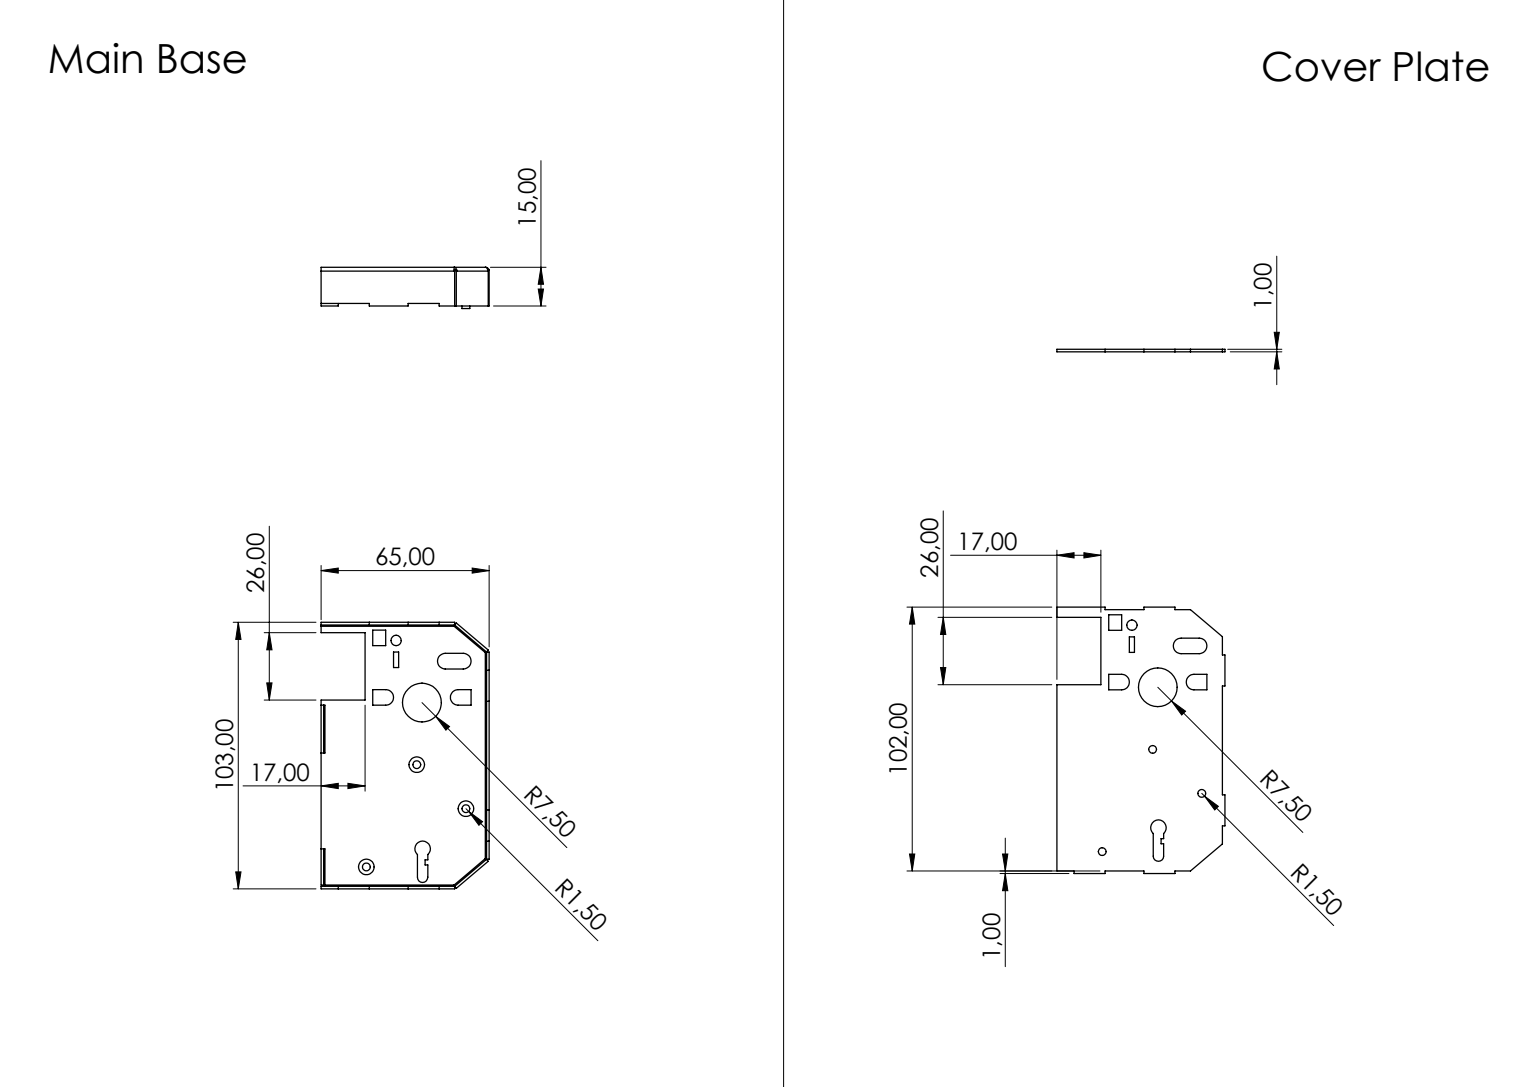
ISO-10303-21;
HEADER;
FILE_DESCRIPTION (('STEP AP214'),
    '1' );
FILE_NAME ('Main Base.step',
    '2026-10-06T13:23:30',
    ( '' ),
    ( '' ),
    'SwSTEP 2.0',
    'SolidWorks 2020',
    '' );
FILE_SCHEMA (( 'AUTOMOTIVE_DESIGN' ));
ENDSEC;

DATA;
#3=VECTOR ( 'NONE', #8048, 1000.000000000000000 ) ;
#6=CARTESIAN_POINT ( 'NONE',  ( -31.50000000000000000, 10.25000000000000000, -137.0552959530000123 ) ) ;
#7=ORIENTED_EDGE ( 'NONE', *, *, #14186, .F. ) ;
#8=PLANE ( 'NONE',  #9401 ) ;
#10=VECTOR ( 'NONE', #7060, 1000.000000000000000 ) ;
#13=DIRECTION ( 'NONE',  ( 0.000000000000000000, 1.000000000000000000, 0.000000000000000000 ) ) ;
#14=CARTESIAN_POINT ( 'NONE',  ( 7.750000000000000000, -40.23606797749999942, -150.0552959529999839 ) ) ;
#16=CARTESIAN_POINT ( 'NONE',  ( -31.00000000000000000, 10.25000000000000000, -150.0552959529999839 ) ) ;
#20=LINE ( 'NONE', #12366, #11445 ) ;
#23=CARTESIAN_POINT ( 'NONE',  ( 6.899000527194547594, -5.343640159924734512, -150.0552959529999839 ) ) ;
#25=EDGE_CURVE ( 'NONE', #1116, #6470, #1636, .T. ) ;
#26=CARTESIAN_POINT ( 'NONE',  ( 32.14594224149999491, 40.79958733410000349, -149.5552959519999945 ) ) ;
#47=ORIENTED_EDGE ( 'NONE', *, *, #19254, .F. ) ;
#51=CARTESIAN_POINT ( 'NONE',  ( 23.00000000000000000, 25.50000000000000000, -151.0552959529999839 ) ) ;
#54=LINE ( 'NONE', #14445, #10 ) ;
#58=CARTESIAN_POINT ( 'NONE',  ( 18.66060904160396916, 20.09818317339116689, -150.0552959529999839 ) ) ;
#59=CARTESIAN_POINT ( 'NONE',  ( -15.75723547076485254, -44.30951848884578226, -150.0552959529999839 ) ) ;
#63=VECTOR ( 'NONE', #17679, 1000.000000000000000 ) ;
#65=LINE ( 'NONE', #14804, #22679 ) ;
#68=EDGE_CURVE ( 'NONE', #3612, #21024, #1516, .T. ) ;
#74=FACE_OUTER_BOUND ( 'NONE', #19510, .T. ) ;
#75=CARTESIAN_POINT ( 'NONE',  ( 7.750000000000000000, -40.23606797749999942, -150.5552959529999839 ) ) ;
#78=EDGE_CURVE ( 'NONE', #537, #6609, #18037, .T. ) ;
#79=CIRCLE ( 'NONE', #13356, 2.000000000000000000 ) ;
#96=VECTOR ( 'NONE', #17767, 1000.000000000000227 ) ;
#102=DIRECTION ( 'NONE',  ( 0.000000000000000000, -1.000000000000000000, 0.000000000000000000 ) ) ;
#103=CARTESIAN_POINT ( 'NONE',  ( -6.024730888589999722, -51.50000000000000000, -149.5552959529999839 ) ) ;
#104=EDGE_CURVE ( 'NONE', #6667, #13256, #16589, .T. ) ;
#105=ORIENTED_EDGE ( 'NONE', *, *, #1127, .F. ) ;
#106=PLANE ( 'NONE',  #15659 ) ;
#111=ORIENTED_EDGE ( 'NONE', *, *, #15327, .F. ) ;
#120=LINE ( 'NONE', #16055, #20099 ) ;
#130=EDGE_LOOP ( 'NONE', ( #1409, #6613, #421, #6495 ) ) ;
#138=DIRECTION ( 'NONE',  ( 1.000000000000000000, 0.000000000000000000, -2.257560236040000027E-12 ) ) ;
#150=EDGE_CURVE ( 'NONE', #19192, #2146, #2095, .T. ) ;
#160=LINE ( 'NONE', #11080, #6868 ) ;
#162=FACE_OUTER_BOUND ( 'NONE', #18152, .T. ) ;
#167=EDGE_LOOP ( 'NONE', ( #4339, #16056, #21520, #10157 ) ) ;
#168=LINE ( 'NONE', #11551, #791 ) ;
#169=CARTESIAN_POINT ( 'NONE',  ( 32.50000000000000000, 40.03620104880000241, -143.0552959529999839 ) ) ;
#170=DIRECTION ( 'NONE',  ( -0.7071067811865474617, -0.7071067811865476838, 0.000000000000000000 ) ) ;
#171=CARTESIAN_POINT ( 'NONE',  ( -3.500000000000000000, 44.50000000000000000, -150.0552959529999839 ) ) ;
#174=VECTOR ( 'NONE', #17768, 1000.000000000000000 ) ;
#186=CARTESIAN_POINT ( 'NONE',  ( 31.50000000000000000, 39.80430157320000006, -149.5552959529999839 ) ) ;
#188=CARTESIAN_POINT ( 'NONE',  ( 31.00000000000000000, 39.80430157320000006, -150.0552959529999839 ) ) ;
#196=CARTESIAN_POINT ( 'NONE',  ( -31.00000000000000000, -50.00000000000000000, -151.0552959529999839 ) ) ;
#198=CARTESIAN_POINT ( 'NONE',  ( 15.50000000000000000, 36.50000000000000000, -151.0552959529999839 ) ) ;
#203=VECTOR ( 'NONE', #22611, 1000.000000000000000 ) ;
#204=CARTESIAN_POINT ( 'NONE',  ( 5.523675324909882001, -48.60111558252668829, -150.0552959529999839 ) ) ;
#211=EDGE_LOOP ( 'NONE', ( #21021, #20847, #5085, #22198, #20574, #16740, #10421 ) ) ;
#212=CARTESIAN_POINT ( 'NONE',  ( -17.62135916506277411, -44.51085694111269930, -150.0552959529999555 ) ) ;
#213=VERTEX_POINT ( 'NONE', #20525 ) ;
#225=EDGE_CURVE ( 'NONE', #11906, #13032, #16136, .T. ) ;
#229=EDGE_CURVE ( 'NONE', #213, #5505, #1240, .T. ) ;
#232=VERTEX_POINT ( 'NONE', #4927 ) ;
#239=CARTESIAN_POINT ( 'NONE',  ( 32.50000000000000000, 0.000000000000000000, -136.0552959530000123 ) ) ;
#240=DIRECTION ( 'NONE',  ( 0.000000000000000000, 0.000000000000000000, 1.000000000000000000 ) ) ;
#244=B_SPLINE_CURVE_WITH_KNOTS ( 'NONE', 3,
 ( #8410, #6271, #1182, #22691, #19238, #11612, #9949, #19010, #11855, #8520, #3074, #13524, #13649, #10184, #20796, #15682, #4613, #4491 ),
 .UNSPECIFIED., .F., .F.,
 ( 4, 2, 2, 2, 2, 2, 2, 2, 4 ),
 ( 0.000000000000000000, 0.1250000000000000000, 0.2500000000000000000, 0.3750000000000000000, 0.5000000000000000000, 0.6250000000000000000, 0.7500000000000000000, 0.8750000000000000000, 1.000000000000000000 ),
 .UNSPECIFIED. ) ;
#250=CARTESIAN_POINT ( 'NONE',  ( 4.107300918301284298, -6.500000000000002665, -150.0552959529999839 ) ) ;
#258=VERTEX_POINT ( 'NONE', #1012 ) ;
#276=ORIENTED_EDGE ( 'NONE', *, *, #19287, .F. ) ;
#278=CARTESIAN_POINT ( 'NONE',  ( 8.750000000000000000, -42.23606797749999942, -150.5552959529999839 ) ) ;
#281=CARTESIAN_POINT ( 'NONE',  ( -15.50000000000000000, 34.50000000000000000, -151.0552959529999839 ) ) ;
#282=DIRECTION ( 'NONE',  ( 0.000000000000000000, -1.000000000000000000, 0.000000000000000000 ) ) ;
#284=FACE_OUTER_BOUND ( 'NONE', #6510, .T. ) ;
#289=CARTESIAN_POINT ( 'NONE',  ( 14.71905350739799623, 33.57650987475365412, -150.0552959530000123 ) ) ;
#294=ORIENTED_EDGE ( 'NONE', *, *, #9256, .T. ) ;
#298=DIRECTION ( 'NONE',  ( 1.000000000000000000, 0.000000000000000000, 0.000000000000000000 ) ) ;
#301=VECTOR ( 'NONE', #7137, 1000.000000000000000 ) ;
#313=PLANE ( 'NONE',  #6728 ) ;
#316=FACE_OUTER_BOUND ( 'NONE', #21887, .T. ) ;
#319=CARTESIAN_POINT ( 'NONE',  ( 6.229273316114841919, -48.94892946173367676, -150.0552959529999839 ) ) ;
#322=VERTEX_POINT ( 'NONE', #6472 ) ;
#328=VERTEX_POINT ( 'NONE', #17655 ) ;
#331=CARTESIAN_POINT ( 'NONE',  ( 13.76008370043819973, 22.44588062467436629, -150.0552959529999839 ) ) ;
#333=LINE ( 'NONE', #16862, #716 ) ;
#335=AXIS2_PLACEMENT_3D ( 'NONE', #20333, #9473, #5804 ) ;
#336=PLANE ( 'NONE',  #4892 ) ;
#340=VECTOR ( 'NONE', #23038, 1000.000000000000000 ) ;
#350=VERTEX_POINT ( 'NONE', #15287 ) ;
#354=EDGE_CURVE ( 'NONE', #22442, #21113, #20876, .T. ) ;
#358=LINE ( 'NONE', #7600, #2620 ) ;
#359=VECTOR ( 'NONE', #21287, 1000.000000000000000 ) ;
#364=DIRECTION ( 'NONE',  ( -1.458135199840000066E-12, 1.723066134159999823E-12, 1.000000000000000000 ) ) ;
#367=LINE ( 'NONE', #7607, #22136 ) ;
#368=EDGE_CURVE ( 'NONE', #19467, #13247, #8432, .T. ) ;
#373=ORIENTED_EDGE ( 'NONE', *, *, #23141, .T. ) ;
#378=AXIS2_PLACEMENT_3D ( 'NONE', #21148, #3175, #6615 ) ;
#381=VECTOR ( 'NONE', #5006, 1000.000000000000000 ) ;
#384=VERTEX_POINT ( 'NONE', #10964 ) ;
#391=EDGE_CURVE ( 'NONE', #6962, #16283, #23127, .T. ) ;
#411=LINE ( 'NONE', #11098, #5597 ) ;
#412=DIRECTION ( 'NONE',  ( 0.000000000000000000, -1.000000000000000000, 0.000000000000000000 ) ) ;
#414=DIRECTION ( 'NONE',  ( 1.000000000000000000, 0.000000000000000000, 0.000000000000000000 ) ) ;
#421=ORIENTED_EDGE ( 'NONE', *, *, #10231, .T. ) ;
#424=CYLINDRICAL_SURFACE ( 'NONE', #5833, 1.500000000000001332 ) ;
#425=ORIENTED_EDGE ( 'NONE', *, *, #10973, .F. ) ;
#427=CARTESIAN_POINT ( 'NONE',  ( 19.45666326950000169, 50.88169314249999786, -136.0552959530000123 ) ) ;
#430=VECTOR ( 'NONE', #16605, 1000.000000000000000 ) ;
#438=CYLINDRICAL_SURFACE ( 'NONE', #17527, 2.999999999999999112 ) ;
#442=CLOSED_SHELL ( 'NONE', ( #9324, #14762, #13056, #18672, #19728, #11827, #3231, #1555, #8168, #17761, #5900, #20748, #17875, #12551, #6898, #10761, #21469, #15064, #5744, #9048, #10757, #19124, #8783, #16660, #5435, #11889, #2238, #21621, #10384, #1685, #10160, #18102, #2306, #16052, #22700, #15391, #3799, #8755, #18283, #22183, #12588, #7262, #14355, #653, #22347, #13377, #4882, #10197, #21282, #7768, #18410, #22521, #11400, #16358, #23317, #3120, #7355, #13403, #22544, #7833, #8957, #20415, #19258, #523, #5604, #17631, #20506, #5512, #10979, #8075, #2679, #9354, #4586, #22200, #23359, #17607, #5542, #23499, #15096, #7365, #9624, #7391, #20151, #23430, #18033, #13348, #7151, #11366, #4409, #5104, #2402, #2042, #18132, #10666, #7930, #20884, #13762, #18713, #18695, #14321, #2065, #14378, #15647, #17406, #4519, #4684, #3694, #21015, #20879, #11134, #7412, #2812, #10561, #7625, #18912, #19316, #9573, #6767, #17249, #18227, #4140, #23025, #5289, #14520, #11229, #648, #6454, #12373, #19083, #6624, #17899, #15037, #11061, #12004, #20941, #16351, #7440, #9553, #16817, #17324, #7025, #19114, #16510, #11613, #13749, #6389, #5831, #9940, #12623, #14887, #20445, #13941, #17758, #16749, #22349, #22437, #10217, #1808, #15771, #12918, #17075, #2483, #7067, #6285, #19351 ) ) ;
#446=ORIENTED_EDGE ( 'NONE', *, *, #8608, .F. ) ;
#450=CARTESIAN_POINT ( 'NONE',  ( -16.51085694111268865, -45.62135916506277056, -150.0552959529999555 ) ) ;
#455=DIRECTION ( 'NONE',  ( -1.000000000000000000, 0.000000000000000000, 0.000000000000000000 ) ) ;
#457=CARTESIAN_POINT ( 'NONE',  ( 19.91945158500000090, -51.14507942810000429, -149.5552959529999839 ) ) ;
#461=LINE ( 'NONE', #9594, #4132 ) ;
#464=AXIS2_PLACEMENT_3D ( 'NONE', #871, #514, #22275 ) ;
#467=VERTEX_POINT ( 'NONE', #15986 ) ;
#479=CARTESIAN_POINT ( 'NONE',  ( 22.50000000000000000, 33.50000000000000000, -150.0552959529999839 ) ) ;
#480=ORIENTED_EDGE ( 'NONE', *, *, #12943, .T. ) ;
#481=PLANE ( 'NONE',  #12091 ) ;
#488=DIRECTION ( 'NONE',  ( 0.000000000000000000, 2.256894259950000208E-12, -1.000000000000000000 ) ) ;
#489=ORIENTED_EDGE ( 'NONE', *, *, #10165, .F. ) ;
#499=ORIENTED_EDGE ( 'NONE', *, *, #14733, .F. ) ;
#501=LINE ( 'NONE', #11416, #1400 ) ;
#502=CARTESIAN_POINT ( 'NONE',  ( -7.500000000000000000, 48.50000000000000000, -150.5552959529999839 ) ) ;
#503=CARTESIAN_POINT ( 'NONE',  ( 31.50000000000000000, -21.03620104879999886, -136.0552959530000123 ) ) ;
#505=ORIENTED_EDGE ( 'NONE', *, *, #9782, .F. ) ;
#507=DIRECTION ( 'NONE',  ( -0.7633862853691872896, 0.6459422414660880296, 5.370703881624201706E-14 ) ) ;
#508=LINE ( 'NONE', #2417, #23112 ) ;
#514=DIRECTION ( 'NONE',  ( 0.000000000000000000, 0.000000000000000000, -1.000000000000000000 ) ) ;
#515=CARTESIAN_POINT ( 'NONE',  ( -12.50000000000000000, 42.50000000000000000, -150.5552959529999839 ) ) ;
#520=DIRECTION ( 'NONE',  ( -1.000000000000000000, 0.000000000000000000, 0.000000000000000000 ) ) ;
#521=EDGE_LOOP ( 'NONE', ( #17341, #16044, #20212, #9730 ) ) ;
#522=DIRECTION ( 'NONE',  ( 0.000000000000000000, 1.000000000000000000, -2.273736754430000208E-12 ) ) ;
#523=ADVANCED_FACE ( 'NONE', ( #5738 ), #15015, .T. ) ;
#529=EDGE_CURVE ( 'NONE', #13555, #22754, #79, .T. ) ;
#533=FACE_OUTER_BOUND ( 'NONE', #22449, .T. ) ;
#537=VERTEX_POINT ( 'NONE', #18717 ) ;
#544=DIRECTION ( 'NONE',  ( 1.000000000000000000, 0.000000000000000000, 0.000000000000000000 ) ) ;
#548=DIRECTION ( 'NONE',  ( 0.000000000000000000, 0.000000000000000000, 1.000000000000000000 ) ) ;
#554=EDGE_CURVE ( 'NONE', #10724, #2155, #2183, .T. ) ;
#556=DIRECTION ( 'NONE',  ( 0.000000000000000000, -1.000000000000000000, 0.000000000000000000 ) ) ;
#557=ORIENTED_EDGE ( 'NONE', *, *, #5693, .F. ) ;
#563=EDGE_LOOP ( 'NONE', ( #12365, #15477, #17819, #6056 ) ) ;
#565=VERTEX_POINT ( 'NONE', #11308 ) ;
#566=CARTESIAN_POINT ( 'NONE',  ( -15.39269908169871393, -46.00000000000000000, -150.0552959529999839 ) ) ;
#567=VERTEX_POINT ( 'NONE', #9642 ) ;
#568=ORIENTED_EDGE ( 'NONE', *, *, #21534, .F. ) ;
#570=CARTESIAN_POINT ( 'NONE',  ( 19.13369214859999801, 51.50000000000000000, -142.8052959529999839 ) ) ;
#571=DIRECTION ( 'NONE',  ( 1.000000000000000000, 0.000000000000000000, -2.255897967639999903E-12 ) ) ;
#575=FACE_OUTER_BOUND ( 'NONE', #12604, .T. ) ;
#581=ORIENTED_EDGE ( 'NONE', *, *, #16197, .T. ) ;
#585=EDGE_LOOP ( 'NONE', ( #1690, #3105, #11478, #4390 ) ) ;
#595=ORIENTED_EDGE ( 'NONE', *, *, #22542, .F. ) ;
#602=CIRCLE ( 'NONE', #14284, 0.5000000000000004441 ) ;
#604=EDGE_LOOP ( 'NONE', ( #581, #786, #19949, #21046 ) ) ;
#605=EDGE_CURVE ( 'NONE', #4355, #13765, #9291, .T. ) ;
#613=CARTESIAN_POINT ( 'NONE',  ( 32.00000000000000000, 32.96379895120000469, -136.0552959530000123 ) ) ;
#617=CARTESIAN_POINT ( 'NONE',  ( 32.50000000000000000, -21.03620104879999886, -136.5552959530000123 ) ) ;
#618=AXIS2_PLACEMENT_3D ( 'NONE', #10592, #19305, #3240 ) ;
#636=FACE_OUTER_BOUND ( 'NONE', #14587, .T. ) ;
#641=CARTESIAN_POINT ( 'NONE',  ( 6.500000000000000000, 13.00000000000000000, -150.0552959529999839 ) ) ;
#648=ADVANCED_FACE ( 'NONE', ( #7405 ), #14667, .F. ) ;
#653=ADVANCED_FACE ( 'NONE', ( #8333 ), #17029, .T. ) ;
#659=VECTOR ( 'NONE', #1651, 1000.000000000000000 ) ;
#663=AXIS2_PLACEMENT_3D ( 'NONE', #6976, #3646, #1872 ) ;
#668=EDGE_CURVE ( 'NONE', #11661, #7563, #4778, .T. ) ;
#671=ORIENTED_EDGE ( 'NONE', *, *, #7862, .F. ) ;
#682=CARTESIAN_POINT ( 'NONE',  ( -32.50000000000000000, 0.000000000000000000, -150.0552959529999839 ) ) ;
#684=EDGE_CURVE ( 'NONE', #11278, #7890, #748, .T. ) ;
#687=DIRECTION ( 'NONE',  ( 0.000000000000000000, -2.256894259950000208E-12, 1.000000000000000000 ) ) ;
#688=FACE_OUTER_BOUND ( 'NONE', #3217, .T. ) ;
#692=EDGE_LOOP ( 'NONE', ( #18060, #16442, #20942, #9453 ) ) ;
#693=CARTESIAN_POINT ( 'NONE',  ( -1.500000000000000222, 44.76558107705237433, -150.0552959530000123 ) ) ;
#707=DIRECTION ( 'NONE',  ( 0.000000000000000000, -2.257144641399999941E-12, -1.000000000000000000 ) ) ;
#709=DIRECTION ( 'NONE',  ( 0.000000000000000000, -1.000000000000000000, 2.257144641399999941E-12 ) ) ;
#710=EDGE_CURVE ( 'NONE', #6873, #1863, #12236, .T. ) ;
#714=VECTOR ( 'NONE', #22848, 1000.000000000000000 ) ;
#715=DIRECTION ( 'NONE',  ( 0.000000000000000000, 1.000000000000000000, 0.000000000000000000 ) ) ;
#716=VECTOR ( 'NONE', #6030, 1000.000000000000227 ) ;
#718=LINE ( 'NONE', #13669, #23526 ) ;
#726=ORIENTED_EDGE ( 'NONE', *, *, #17540, .T. ) ;
#728=CARTESIAN_POINT ( 'NONE',  ( 2.989143058887297588, -0.8786408349372282212, -150.0552959529999839 ) ) ;
#734=ORIENTED_EDGE ( 'NONE', *, *, #17234, .F. ) ;
#748=LINE ( 'NONE', #982, #17937 ) ;
#751=VERTEX_POINT ( 'NONE', #19292 ) ;
#752=DIRECTION ( 'NONE',  ( 0.000000000000000000, 1.000000000000000000, 0.000000000000000000 ) ) ;
#754=ORIENTED_EDGE ( 'NONE', *, *, #1639, .F. ) ;
#759=DIRECTION ( 'NONE',  ( -0.000000000000000000, 1.000000000000000000, 0.000000000000000000 ) ) ;
#763=CARTESIAN_POINT ( 'NONE',  ( 3.175226511974131860, 13.75903940329096287, -150.0552959529999839 ) ) ;
#764=DIRECTION ( 'NONE',  ( 1.000000000000000000, 0.000000000000000000, 0.000000000000000000 ) ) ;
#770=EDGE_CURVE ( 'NONE', #14651, #10724, #872, .T. ) ;
#783=CARTESIAN_POINT ( 'NONE',  ( 19.13369214859999801, 50.50000000000000000, -149.5552959529999839 ) ) ;
#784=EDGE_CURVE ( 'NONE', #19299, #9007, #13572, .T. ) ;
#786=ORIENTED_EDGE ( 'NONE', *, *, #16235, .T. ) ;
#791=VECTOR ( 'NONE', #522, 1000.000000000000000 ) ;
#802=VERTEX_POINT ( 'NONE', #11658 ) ;
#806=ORIENTED_EDGE ( 'NONE', *, *, #21641, .F. ) ;
#809=CARTESIAN_POINT ( 'NONE',  ( 32.50000000000000000, -0.03620104877499999430, -136.0552959530000123 ) ) ;
#816=ORIENTED_EDGE ( 'NONE', *, *, #7911, .T. ) ;
#822=LINE ( 'NONE', #2948, #3 ) ;
#828=CARTESIAN_POINT ( 'NONE',  ( -32.50000000000000000, -24.50000000000000000, -150.0552959529999839 ) ) ;
#837=LINE ( 'NONE', #2962, #359 ) ;
#844=VERTEX_POINT ( 'NONE', #14722 ) ;
#848=AXIS2_PLACEMENT_3D ( 'NONE', #14666, #9179, #20152 ) ;
#850=ORIENTED_EDGE ( 'NONE', *, *, #21643, .T. ) ;
#861=CARTESIAN_POINT ( 'NONE',  ( 31.50000000000000000, -33.03620104880000241, -143.0552959529999839 ) ) ;
#867=CARTESIAN_POINT ( 'NONE',  ( -7.520331543250000195, 50.50000000000000000, -149.5552959529999839 ) ) ;
#871=CARTESIAN_POINT ( 'NONE',  ( 20.50000000000000000, 22.50000000000000000, -151.0552959529999839 ) ) ;
#872=LINE ( 'NONE', #6210, #17180 ) ;
#879=CIRCLE ( 'NONE', #6567, 0.5000000000000004441 ) ;
#902=LINE ( 'NONE', #9909, #21670 ) ;
#903=VERTEX_POINT ( 'NONE', #1455 ) ;
#904=DIRECTION ( 'NONE',  ( 0.000000000000000000, -2.257144641399999941E-12, -1.000000000000000000 ) ) ;
#916=SURFACE_SIDE_STYLE ('',( #15534 ) ) ;
#918=DIRECTION ( 'NONE',  ( 0.000000000000000000, 1.000000000000000000, 0.000000000000000000 ) ) ;
#934=ORIENTED_EDGE ( 'NONE', *, *, #10109, .T. ) ;
#935=VECTOR ( 'NONE', #3004, 1000.000000000000000 ) ;
#938=DIRECTION ( 'NONE',  ( 2.257144641399999941E-12, 0.000000000000000000, 1.000000000000000000 ) ) ;
#944=ORIENTED_EDGE ( 'NONE', *, *, #2669, .F. ) ;
#949=DIRECTION ( 'NONE',  ( -3.552713678800000397E-15, 0.000000000000000000, 1.000000000000000000 ) ) ;
#952=EDGE_CURVE ( 'NONE', #22710, #537, #20436, .T. ) ;
#954=VERTEX_POINT ( 'NONE', #20786 ) ;
#964=CARTESIAN_POINT ( 'NONE',  ( 7.121359165062772334, -1.989143058887300475, -150.0552959530000123 ) ) ;
#968=VERTEX_POINT ( 'NONE', #16742 ) ;
#970=DIRECTION ( 'NONE',  ( 0.000000000000000000, 0.000000000000000000, 1.000000000000000000 ) ) ;
#972=CARTESIAN_POINT ( 'NONE',  ( -13.50000000000000000, -42.80126216859517996, -150.0552959529999839 ) ) ;
#974=DIRECTION ( 'NONE',  ( -1.000000000000000000, 0.000000000000000000, -2.273736754430000208E-12 ) ) ;
#977=DIRECTION ( 'NONE',  ( 0.000000000000000000, 1.000000000000000000, 0.000000000000000000 ) ) ;
#980=EDGE_CURVE ( 'NONE', #11681, #2055, #20670, .T. ) ;
#981=DIRECTION ( 'NONE',  ( 0.000000000000000000, 0.000000000000000000, -1.000000000000000000 ) ) ;
#982=CARTESIAN_POINT ( 'NONE',  ( -31.75000000000000000, 19.50000000000000000, -151.0552959529999839 ) ) ;
#984=EDGE_CURVE ( 'NONE', #1160, #14539, #11488, .T. ) ;
#985=ORIENTED_EDGE ( 'NONE', *, *, #18589, .F. ) ;
#992=AXIS2_PLACEMENT_3D ( 'NONE', #3546, #17821, #18174 ) ;
#995=DIRECTION ( 'NONE',  ( 0.000000000000000000, 1.000000000000000000, 0.000000000000000000 ) ) ;
#1000=CARTESIAN_POINT ( 'NONE',  ( 6.750000000000000000, -36.00000000000000000, -150.0552959529999839 ) ) ;
#1002=PLANE ( 'NONE',  #9686 ) ;
#1003=CARTESIAN_POINT ( 'NONE',  ( 8.701166446538422861, -33.70126136998415944, -150.0552959529999839 ) ) ;
#1012=CARTESIAN_POINT ( 'NONE',  ( 32.14594224169999848, -40.79958733389999992, -136.0552959530000123 ) ) ;
#1017=DIRECTION ( 'NONE',  ( -1.000000000000000000, 0.000000000000000000, 0.000000000000000000 ) ) ;
#1024=AXIS2_PLACEMENT_3D ( 'NONE', #1323, #8898, #21306 ) ;
#1027=ORIENTED_EDGE ( 'NONE', *, *, #68, .F. ) ;
#1029=EDGE_CURVE ( 'NONE', #14361, #2146, #5314, .T. ) ;
#1030=VERTEX_POINT ( 'NONE', #22453 ) ;
#1035=ORIENTED_EDGE ( 'NONE', *, *, #2912, .F. ) ;
#1042=LINE ( 'NONE', #15781, #17871 ) ;
#1048=DIRECTION ( 'NONE',  ( -1.000000000000000000, 0.000000000000000000, 0.000000000000000000 ) ) ;
#1053=DIRECTION ( 'NONE',  ( 1.457985068979999943E-12, -1.723073263340000007E-12, -1.000000000000000000 ) ) ;
#1056=ORIENTED_EDGE ( 'NONE', *, *, #18194, .T. ) ;
#1062=VERTEX_POINT ( 'NONE', #22221 ) ;
#1071=CARTESIAN_POINT ( 'NONE',  ( -7.500000000000000000, 19.50000000000000000, -151.0552959529999839 ) ) ;
#1077=DIRECTION ( 'NONE',  ( -0.7633862853691523176, -0.6459422414661291079, 0.000000000000000000 ) ) ;
#1085=PLANE ( 'NONE',  #7781 ) ;
#1088=EDGE_LOOP ( 'NONE', ( #10214, #10164, #17790, #19615 ) ) ;
#1096=VECTOR ( 'NONE', #10422, 1000.000000000000000 ) ;
#1097=EDGE_CURVE ( 'NONE', #6873, #213, #22682, .T. ) ;
#1102=DIRECTION ( 'NONE',  ( 0.000000000000000000, -1.000000000000000000, 2.273736754430000208E-12 ) ) ;
#1104=VERTEX_POINT ( 'NONE', #12318 ) ;
#1116=VERTEX_POINT ( 'NONE', #19482 ) ;
#1127=EDGE_CURVE ( 'NONE', #7397, #7971, #1042, .T. ) ;
#1128=CARTESIAN_POINT ( 'NONE',  ( 4.055709778248144382, -34.64604587945159864, -150.0552959529999839 ) ) ;
#1132=AXIS2_PLACEMENT_3D ( 'NONE', #9763, #13584, #4554 ) ;
#1134=CIRCLE ( 'NONE', #9463, 3.000000000000000000 ) ;
#1147=CARTESIAN_POINT ( 'NONE',  ( -12.37864083493722589, -41.48914305888730070, -150.0552959530000123 ) ) ;
#1154=AXIS2_PLACEMENT_3D ( 'NONE', #17896, #14566, #16350 ) ;
#1160=VERTEX_POINT ( 'NONE', #8975 ) ;
#1161=DIRECTION ( 'NONE',  ( 1.000000000000000000, 0.000000000000000000, 0.000000000000000000 ) ) ;
#1164=EDGE_LOOP ( 'NONE', ( #6286, #1314, #2583, #12664 ) ) ;
#1167=ORIENTED_EDGE ( 'NONE', *, *, #17932, .F. ) ;
#1176=DIRECTION ( 'NONE',  ( -0.000000000000000000, 1.000000000000000000, 0.000000000000000000 ) ) ;
#1180=EDGE_CURVE ( 'NONE', #7409, #9410, #21742, .T. ) ;
#1181=FACE_OUTER_BOUND ( 'NONE', #20198, .T. ) ;
#1182=CARTESIAN_POINT ( 'NONE',  ( 23.28094649261545612, 39.42349012523344243, -150.0552959530000123 ) ) ;
#1199=PRODUCT_DEFINITION_SHAPE ( 'NONE', 'NONE',  #3542 ) ;
#1205=LINE ( 'NONE', #2743, #20140 ) ;
#1207=CARTESIAN_POINT ( 'NONE',  ( -25.86630785139999844, -51.50000000000000000, -136.5552959530000123 ) ) ;
#1217=VERTEX_POINT ( 'NONE', #20763 ) ;
#1219=CARTESIAN_POINT ( 'NONE',  ( 20.49999999999999645, -20.10730091830128430, -150.0552959529999839 ) ) ;
#1223=VECTOR ( 'NONE', #7853, 1000.000000000000000 ) ;
#1225=AXIS2_PLACEMENT_3D ( 'NONE', #4775, #17268, #977 ) ;
#1226=DIRECTION ( 'NONE',  ( 0.000000000000000000, 2.256988247010000033E-12, 1.000000000000000000 ) ) ;
#1229=DIRECTION ( 'NONE',  ( -1.000000000000000000, 0.000000000000000000, 0.000000000000000000 ) ) ;
#1235=CARTESIAN_POINT ( 'NONE',  ( 3.190548969991207962, -2.742602116062627271, -150.0552959529999839 ) ) ;
#1236=ORIENTED_EDGE ( 'NONE', *, *, #2105, .F. ) ;
#1240=CIRCLE ( 'NONE', #2374, 1.499999999999998446 ) ;
#1241=DIRECTION ( 'NONE',  ( 0.000000000000000000, 0.000000000000000000, 1.000000000000000000 ) ) ;
#1247=DIRECTION ( 'NONE',  ( 1.000000000000000000, 0.000000000000000000, 0.000000000000000000 ) ) ;
#1261=DIRECTION ( 'NONE',  ( 0.7633862853691524286, 0.6459422414661292189, -7.105427357551423529E-15 ) ) ;
#1265=DIRECTION ( 'NONE',  ( 2.257144641399999941E-12, 0.000000000000000000, 1.000000000000000000 ) ) ;
#1267=EDGE_CURVE ( 'NONE', #22797, #7563, #11340, .T. ) ;
#1269=CARTESIAN_POINT ( 'NONE',  ( -16.20076496858231963, -43.91979154561150267, -150.0552959529999839 ) ) ;
#1273=CARTESIAN_POINT ( 'NONE',  ( 5.419791545609164984, -4.700764968563650115, -150.0552959529999555 ) ) ;
#1280=ORIENTED_EDGE ( 'NONE', *, *, #16797, .F. ) ;
#1281=EDGE_LOOP ( 'NONE', ( #19318, #13543, #14266, #17955 ) ) ;
#1287=DIRECTION ( 'NONE',  ( 0.000000000000000000, 0.000000000000000000, -1.000000000000000000 ) ) ;
#1300=DIRECTION ( 'NONE',  ( 0.7071067811865473507, 0.7071067811865477948, 0.000000000000000000 ) ) ;
#1301=VERTEX_POINT ( 'NONE', #20648 ) ;
#1307=ORIENTED_EDGE ( 'NONE', *, *, #10406, .T. ) ;
#1308=VECTOR ( 'NONE', #949, 1000.000000000000000 ) ;
#1313=EDGE_CURVE ( 'NONE', #18451, #1301, #8009, .T. ) ;
#1314=ORIENTED_EDGE ( 'NONE', *, *, #19463, .T. ) ;
#1315=CARTESIAN_POINT ( 'NONE',  ( 32.50000000000000000, 20.96379895120000114, -137.0552959530000123 ) ) ;
#1316=CARTESIAN_POINT ( 'NONE',  ( -32.50000000000000000, 47.50000000000000000, -151.0552959529999839 ) ) ;
#1317=ORIENTED_EDGE ( 'NONE', *, *, #12829, .F. ) ;
#1318=DIRECTION ( 'NONE',  ( 1.000000000000000000, 0.000000000000000000, 0.000000000000000000 ) ) ;
#1320=CARTESIAN_POINT ( 'NONE',  ( 31.50000000000000000, -0.1159497378070000057, -149.5552959529999839 ) ) ;
#1322=ORIENTED_EDGE ( 'NONE', *, *, #3520, .T. ) ;
#1323=CARTESIAN_POINT ( 'NONE',  ( -6.683153925719999222, -51.50000000000000000, -150.0552959529999839 ) ) ;
#1327=EDGE_LOOP ( 'NONE', ( #7904, #19498, #22770, #2319 ) ) ;
#1328=PLANE ( 'NONE',  #6291 ) ;
#1329=FACE_OUTER_BOUND ( 'NONE', #21772, .T. ) ;
#1335=EDGE_CURVE ( 'NONE', #322, #21462, #16714, .T. ) ;
#1344=ORIENTED_EDGE ( 'NONE', *, *, #21880, .F. ) ;
#1355=DIRECTION ( 'NONE',  ( 0.000000000000000000, 0.000000000000000000, 1.000000000000000000 ) ) ;
#1357=DIRECTION ( 'NONE',  ( 0.000000000000000000, 0.000000000000000000, 1.000000000000000000 ) ) ;
#1363=DIRECTION ( 'NONE',  ( 1.457985068979999943E-12, 1.723073263340000007E-12, -1.000000000000000000 ) ) ;
#1370=CARTESIAN_POINT ( 'NONE',  ( -32.50000000000000000, 19.50000000000000000, -151.0552959529999839 ) ) ;
#1371=EDGE_CURVE ( 'NONE', #21536, #6962, #23017, .T. ) ;
#1386=VERTEX_POINT ( 'NONE', #8243 ) ;
#1390=EDGE_LOOP ( 'NONE', ( #8124, #20683, #10522, #22148 ) ) ;
#1391=ORIENTED_EDGE ( 'NONE', *, *, #18377, .F. ) ;
#1392=DIRECTION ( 'NONE',  ( 0.000000000000000000, 1.000000000000000000, 0.000000000000000000 ) ) ;
#1397=ORIENTED_EDGE ( 'NONE', *, *, #13616, .T. ) ;
#1400=VECTOR ( 'NONE', #9278, 1000.000000000000000 ) ;
#1404=B_SPLINE_CURVE_WITH_KNOTS ( 'NONE', 1,
 ( #18749, #9917 ),
 .UNSPECIFIED., .F., .F.,
 ( 2, 2 ),
 ( -6.000000000000000000, 6.000000000000000000 ),
 .UNSPECIFIED. ) ;
#1409=ORIENTED_EDGE ( 'NONE', *, *, #7932, .F. ) ;
#1411=FACE_OUTER_BOUND ( 'NONE', #3594, .T. ) ;
#1417=EDGE_LOOP ( 'NONE', ( #11256, #21139, #23417, #7533 ) ) ;
#1424=VERTEX_POINT ( 'NONE', #21360 ) ;
#1434=ORIENTED_EDGE ( 'NONE', *, *, #9513, .T. ) ;
#1439=EDGE_CURVE ( 'NONE', #1936, #23105, #902, .T. ) ;
#1443=CARTESIAN_POINT ( 'NONE',  ( 23.50000000000000000, -20.50000000000000000, -137.0552959530000123 ) ) ;
#1444=CARTESIAN_POINT ( 'NONE',  ( -13.50000000000000000, -43.00000000000000000, -150.0552959529999839 ) ) ;
#1446=CARTESIAN_POINT ( 'NONE',  ( 18.95053822279999878, 51.50000000000000000, -149.5552959529999839 ) ) ;
#1452=CARTESIAN_POINT ( 'NONE',  ( -6.366307851710000243, -51.50000000000000000, -136.0552959530000123 ) ) ;
#1455=CARTESIAN_POINT ( 'NONE',  ( -31.50000000000000000, 19.50000000000000000, -149.5552959529999839 ) ) ;
#1457=ORIENTED_EDGE ( 'NONE', *, *, #22542, .T. ) ;
#1461=DIRECTION ( 'NONE',  ( 0.000000000000000000, -2.256894259950000208E-12, 1.000000000000000000 ) ) ;
#1463=DIRECTION ( 'NONE',  ( 0.000000000000000000, -1.000000000000000000, 2.257453483404482811E-12 ) ) ;
#1465=CARTESIAN_POINT ( 'NONE',  ( 22.00000000000000000, -20.50000000000000000, -135.0552959530000123 ) ) ;
#1479=FACE_OUTER_BOUND ( 'NONE', #12093, .T. ) ;
#1485=AXIS2_PLACEMENT_3D ( 'NONE', #19777, #12621, #18343 ) ;
#1488=CARTESIAN_POINT ( 'NONE',  ( -31.00000000000000000, 0.000000000000000000, -150.0552959529999839 ) ) ;
#1496=CARTESIAN_POINT ( 'NONE',  ( -15.39269908169872814, -40.00000000000000000, -150.0552959529999555 ) ) ;
#1502=DIRECTION ( 'NONE',  ( 0.000000000000000000, 1.000000000000000000, 0.000000000000000000 ) ) ;
#1505=AXIS2_PLACEMENT_3D ( 'NONE', #2481, #16980, #20221 ) ;
#1516=LINE ( 'NONE', #8738, #9157 ) ;
#1517=ORIENTED_EDGE ( 'NONE', *, *, #20608, .F. ) ;
#1518=CARTESIAN_POINT ( 'NONE',  ( -5.660514123339918768, 20.09808825513541208, -150.0552959529999839 ) ) ;
#1523=DIRECTION ( 'NONE',  ( -0.7633862853691524286, 0.6459422414661292189, -2.886579864030575227E-15 ) ) ;
#1533=EDGE_CURVE ( 'NONE', #17988, #2949, #23369, .T. ) ;
#1536=EDGE_LOOP ( 'NONE', ( #20552, #1056, #13949, #18491 ) ) ;
#1539=ORIENTED_EDGE ( 'NONE', *, *, #18978, .T. ) ;
#1540=CARTESIAN_POINT ( 'NONE',  ( 26.50000000000000000, -20.50000000000000000, -150.0552959529999839 ) ) ;
#1541=ORIENTED_EDGE ( 'NONE', *, *, #3184, .T. ) ;
#1545=EDGE_LOOP ( 'NONE', ( #12281, #19267, #14801, #9609 ) ) ;
#1547=VECTOR ( 'NONE', #16114, 1000.000000000000000 ) ;
#1553=ORIENTED_EDGE ( 'NONE', *, *, #6685, .F. ) ;
#1555=ADVANCED_FACE ( 'NONE', ( #3374 ), #10615, .T. ) ;
#1560=EDGE_CURVE ( 'NONE', #16877, #6475, #54, .T. ) ;
#1562=ORIENTED_EDGE ( 'NONE', *, *, #14186, .T. ) ;
#1564=AXIS2_PLACEMENT_3D ( 'NONE', #18973, #1265, #13968 ) ;
#1572=PLANE ( 'NONE',  #22828 ) ;
#1579=CARTESIAN_POINT ( 'NONE',  ( 1.578081969995054568, -4.285243653077847270, -150.0552959530000123 ) ) ;
#1581=CIRCLE ( 'NONE', #663, 1.499999999999996225 ) ;
#1584=CARTESIAN_POINT ( 'NONE',  ( 18.95053822279999878, -50.00000000000000000, -150.5552959529999839 ) ) ;
#1585=VECTOR ( 'NONE', #13004, 1000.000000000000000 ) ;
#1591=CARTESIAN_POINT ( 'NONE',  ( -10.00000000000000000, 25.50000000000000000, -150.0552959529999839 ) ) ;
#1600=AXIS2_PLACEMENT_3D ( 'NONE', #16675, #18813, #11188 ) ;
#1602=AXIS2_PLACEMENT_3D ( 'NONE', #19669, #3608, #14558 ) ;
#1608=ORIENTED_EDGE ( 'NONE', *, *, #1097, .T. ) ;
#1614=CARTESIAN_POINT ( 'NONE',  ( 8.750000000000000000, -44.61803398880000060, -150.0552959529999839 ) ) ;
#1621=CARTESIAN_POINT ( 'NONE',  ( 19.71940181154762328, 25.42378041200768379, -150.0552959530000123 ) ) ;
#1624=DIRECTION ( 'NONE',  ( -0.6459422414661291079, -0.7633862853691523176, -2.273736754430455399E-12 ) ) ;
#1626=CARTESIAN_POINT ( 'NONE',  ( 1.500000000000000000, -3.500000000000000000, -145.5552959529999839 ) ) ;
#1627=CARTESIAN_POINT ( 'NONE',  ( -13.86630785140000022, 51.50000000000000000, -137.0552959530000123 ) ) ;
#1628=DIRECTION ( 'NONE',  ( 0.000000000000000000, 1.000000000000000000, 0.000000000000000000 ) ) ;
#1632=ORIENTED_EDGE ( 'NONE', *, *, #11313, .T. ) ;
#1634=DIRECTION ( 'NONE',  ( -1.457985068979999943E-12, -1.723073263340000007E-12, 1.000000000000000000 ) ) ;
#1636=LINE ( 'NONE', #23390, #19437 ) ;
#1637=DIRECTION ( 'NONE',  ( -1.000000000000000000, 0.000000000000000000, 0.000000000000000000 ) ) ;
#1639=EDGE_CURVE ( 'NONE', #8510, #12200, #10492, .T. ) ;
#1645=ORIENTED_EDGE ( 'NONE', *, *, #18967, .F. ) ;
#1650=DIRECTION ( 'NONE',  ( -0.000000000000000000, 1.000000000000000000, 0.000000000000000000 ) ) ;
#1651=DIRECTION ( 'NONE',  ( 0.000000000000000000, 2.256894259919999967E-12, 1.000000000000000000 ) ) ;
#1653=CYLINDRICAL_SURFACE ( 'NONE', #14492, 2.000000000000001776 ) ;
#1685=ADVANCED_FACE ( 'NONE', ( #1329 ), #6779, .T. ) ;
#1687=FACE_OUTER_BOUND ( 'NONE', #3541, .T. ) ;
#1688=PLANE ( 'NONE',  #13621 ) ;
#1690=ORIENTED_EDGE ( 'NONE', *, *, #8351, .T. ) ;
#1694=LINE ( 'NONE', #9027, #12502 ) ;
#1697=DIRECTION ( 'NONE',  ( -1.000000000000000000, 0.000000000000000000, 0.000000000000000000 ) ) ;
#1699=VECTOR ( 'NONE', #13346, 1000.000000000000000 ) ;
#1705=VERTEX_POINT ( 'NONE', #1444 ) ;
#1719=DIRECTION ( 'NONE',  ( 0.000000000000000000, 0.000000000000000000, 1.000000000000000000 ) ) ;
#1721=EDGE_CURVE ( 'NONE', #9450, #15840, #16517, .T. ) ;
#1729=ORIENTED_EDGE ( 'NONE', *, *, #12566, .T. ) ;
#1731=CARTESIAN_POINT ( 'NONE',  ( 18.09808825512843455, 20.66051412331523451, -150.0552959529999839 ) ) ;
#1733=AXIS2_PLACEMENT_3D ( 'NONE', #18267, #7423, #1856 ) ;
#1734=LINE ( 'NONE', #12531, #20139 ) ;
#1736=CARTESIAN_POINT ( 'NONE',  ( 31.50000000000000000, -33.03620104880000241, -136.0552959530000123 ) ) ;
#1741=EDGE_LOOP ( 'NONE', ( #373, #5143, #19981, #17412 ) ) ;
#1744=ORIENTED_EDGE ( 'NONE', *, *, #18092, .T. ) ;
#1745=CIRCLE ( 'NONE', #10058, 1.500000000000001332 ) ;
#1748=CARTESIAN_POINT ( 'NONE',  ( 15.50000000000000000, 33.50000000000000000, -150.5552959529999839 ) ) ;
#1750=DIRECTION ( 'NONE',  ( 0.000000000000000000, 0.000000000000000000, 1.000000000000000000 ) ) ;
#1751=EDGE_LOOP ( 'NONE', ( #7956, #16364 ) ) ;
#1752=CARTESIAN_POINT ( 'NONE',  ( -4.500000000000000000, 37.00000000000000000, -150.0552959529999839 ) ) ;
#1755=FACE_OUTER_BOUND ( 'NONE', #6923, .T. ) ;
#1758=EDGE_LOOP ( 'NONE', ( #23285, #13392 ) ) ;
#1760=CARTESIAN_POINT ( 'NONE',  ( -31.50000000000000000, 19.50000000000000000, -143.3052959529999839 ) ) ;
#1763=VECTOR ( 'NONE', #6573, 1000.000000000000000 ) ;
#1764=EDGE_LOOP ( 'NONE', ( #7838, #22300, #568, #5436, #6540, #6553, #20066, #16969, #22280, #14198, #5137, #4958, #14790, #3028, #111 ) ) ;
#1767=FACE_OUTER_BOUND ( 'NONE', #16448, .T. ) ;
#1768=ORIENTED_EDGE ( 'NONE', *, *, #5585, .F. ) ;
#1773=FACE_OUTER_BOUND ( 'NONE', #8786, .T. ) ;
#1776=CARTESIAN_POINT ( 'NONE',  ( -5.449266527207747401, 43.97928331370365385, -150.0552959530000123 ) ) ;
#1782=ORIENTED_EDGE ( 'NONE', *, *, #3711, .T. ) ;
#1783=AXIS2_PLACEMENT_3D ( 'NONE', #3514, #16004, #3050 ) ;
#1786=CARTESIAN_POINT ( 'NONE',  ( 8.750000000000000000, -38.23606797749999942, -151.0552959529999839 ) ) ;
#1787=EDGE_LOOP ( 'NONE', ( #4671, #15389, #22325, #20050 ) ) ;
#1789=ORIENTED_EDGE ( 'NONE', *, *, #10649, .F. ) ;
#1793=DIRECTION ( 'NONE',  ( 0.000000000000000000, -1.000000000000000000, 0.000000000000000000 ) ) ;
#1794=VECTOR ( 'NONE', #22122, 1000.000000000000000 ) ;
#1797=EDGE_CURVE ( 'NONE', #322, #7233, #14526, .T. ) ;
#1799=CARTESIAN_POINT ( 'NONE',  ( 32.50000000000000000, -39.80430157320000006, -149.5552959529999839 ) ) ;
#1803=EDGE_LOOP ( 'NONE', ( #22187, #5500, #20182, #8623 ) ) ;
#1806=LINE ( 'NONE', #14287, #7614 ) ;
#1807=CARTESIAN_POINT ( 'NONE',  ( 7.421918030004952094, -4.285243653077828618, -150.0552959530000123 ) ) ;
#1808=ADVANCED_FACE ( 'NONE', ( #3812, #21902, #18327, #16533, #12834, #3331, #1924, #17854, #2039 ), #1572, .F. ) ;
#1811=CIRCLE ( 'NONE', #15854, 0.5000000000000004441 ) ;
#1814=VECTOR ( 'NONE', #10597, 1000.000000000000000 ) ;
#1815=CARTESIAN_POINT ( 'NONE',  ( -32.50000000000000000, -51.50000000000000000, -149.5552959519999945 ) ) ;
#1831=ORIENTED_EDGE ( 'NONE', *, *, #19563, .T. ) ;
#1833=DIRECTION ( 'NONE',  ( 0.000000000000000000, 0.000000000000000000, 1.000000000000000000 ) ) ;
#1836=CARTESIAN_POINT ( 'NONE',  ( 31.82297112080000190, 40.41789419139999495, -149.5552959529999839 ) ) ;
#1840=EDGE_LOOP ( 'NONE', ( #12851, #21123, #11960, #23063 ) ) ;
#1841=FACE_OUTER_BOUND ( 'NONE', #9955, .T. ) ;
#1844=VECTOR ( 'NONE', #23210, 1000.000000000000000 ) ;
#1846=PLANE ( 'NONE',  #21250 ) ;
#1852=CARTESIAN_POINT ( 'NONE',  ( 32.14594224149999491, 40.79958733410000349, -142.8052959529999839 ) ) ;
#1854=CARTESIAN_POINT ( 'NONE',  ( 19.59648046430000079, -50.76338628540000286, -149.5552959529999839 ) ) ;
#1856=DIRECTION ( 'NONE',  ( 0.000000000000000000, -0.7071067811870332953, 0.7071067811860618502 ) ) ;
#1859=UNCERTAINTY_MEASURE_WITH_UNIT (LENGTH_MEASURE( 1.000000000000000082E-05 ), #20777, 'distance_accuracy_value', 'NONE');
#1860=AXIS2_PLACEMENT_3D ( 'NONE', #4174, #13436, #6191 ) ;
#1863=VERTEX_POINT ( 'NONE', #1799 ) ;
#1872=DIRECTION ( 'NONE',  ( 0.6459422414661299960, -0.7633862853691516515, 0.000000000000000000 ) ) ;
#1879=CIRCLE ( 'NONE', #335, 2.000000000000000000 ) ;
#1881=CIRCLE ( 'NONE', #14023, 7.499999999999999112 ) ;
#1882=CARTESIAN_POINT ( 'NONE',  ( -31.50000000000000000, 19.50000000000000000, -137.0552959530000123 ) ) ;
#1886=LINE ( 'NONE', #7226, #2707 ) ;
#1904=VECTOR ( 'NONE', #5881, 1000.000000000000000 ) ;
#1907=CIRCLE ( 'NONE', #3053, 2.000000000000000888 ) ;
#1914=CARTESIAN_POINT ( 'NONE',  ( 7.750000000000000000, -42.23606797749999942, -150.0552959529999839 ) ) ;
#1921=VECTOR ( 'NONE', #548, 1000.000000000000000 ) ;
#1924=FACE_BOUND ( 'NONE', #3093, .T. ) ;
#1933=CARTESIAN_POINT ( 'NONE',  ( 1.878640834937229442, -5.010856941112704632, -150.0552959530000123 ) ) ;
#1936=VERTEX_POINT ( 'NONE', #12615 ) ;
#1947=DIRECTION ( 'NONE',  ( 0.000000000000000000, 1.000000000000000000, -2.245315044929999938E-12 ) ) ;
#1955=FACE_OUTER_BOUND ( 'NONE', #9695, .T. ) ;
#1969=VECTOR ( 'NONE', #544, 1000.000000000000000 ) ;
#1970=CARTESIAN_POINT ( 'NONE',  ( 4.750000000000000000, -42.61803398880000060, -150.0552959529999839 ) ) ;
#1971=VECTOR ( 'NONE', #138, 1000.000000000000000 ) ;
#1983=EDGE_CURVE ( 'NONE', #23428, #9439, #1806, .T. ) ;
#1989=VECTOR ( 'NONE', #20619, 1000.000000000000000 ) ;
#1991=VECTOR ( 'NONE', #3846, 1000.000000000000227 ) ;
#1993=ORIENTED_EDGE ( 'NONE', *, *, #14572, .F. ) ;
#2002=LINE ( 'NONE', #1760, #15023 ) ;
#2023=DIRECTION ( 'NONE',  ( 0.000000000000000000, 0.000000000000000000, 1.000000000000000000 ) ) ;
#2024=DIRECTION ( 'NONE',  ( -2.257242012349999735E-12, 0.000000000000000000, 1.000000000000000000 ) ) ;
#2027=CARTESIAN_POINT ( 'NONE',  ( 19.84954298779999959, 51.20423285649999912, -150.0552959529999839 ) ) ;
#2028=VERTEX_POINT ( 'NONE', #14642 ) ;
#2030=CARTESIAN_POINT ( 'NONE',  ( 18.95053822279999878, 50.00000000000000000, -149.5552959529999839 ) ) ;
#2033=DIRECTION ( 'NONE',  ( 1.000000000000000000, 0.000000000000000000, 0.000000000000000000 ) ) ;
#2039=FACE_OUTER_BOUND ( 'NONE', #4407, .T. ) ;
#2042=ADVANCED_FACE ( 'NONE', ( #23216 ), #16888, .F. ) ;
#2045=VERTEX_POINT ( 'NONE', #22138 ) ;
#2053=PLANE ( 'NONE',  #1485 ) ;
#2055=VERTEX_POINT ( 'NONE', #4285 ) ;
#2065=ADVANCED_FACE ( 'NONE', ( #16651 ), #2157, .F. ) ;
#2066=CARTESIAN_POINT ( 'NONE',  ( 19.84954298759999958, -51.20423285660000090, -149.5552959529999839 ) ) ;
#2069=CARTESIAN_POINT ( 'NONE',  ( -32.50000000000000000, -36.00000000000000000, -137.0552959530000123 ) ) ;
#2070=EDGE_CURVE ( 'NONE', #350, #12137, #20467, .T. ) ;
#2074=CARTESIAN_POINT ( 'NONE',  ( -3.500000000000000000, 44.50000000000000000, -150.0552959529999839 ) ) ;
#2082=DIRECTION ( 'NONE',  ( 0.7071067811865473507, -0.7071067811865477948, 0.000000000000000000 ) ) ;
#2086=PLANE ( 'NONE',  #2566 ) ;
#2087=DIRECTION ( 'NONE',  ( -2.257144641399999941E-12, 0.000000000000000000, 1.000000000000000000 ) ) ;
#2095=LINE ( 'NONE', #22078, #1969 ) ;
#2102=ORIENTED_EDGE ( 'NONE', *, *, #2124, .T. ) ;
#2105=EDGE_CURVE ( 'NONE', #3167, #20530, #9376, .T. ) ;
#2110=CARTESIAN_POINT ( 'NONE',  ( 31.00000000000000000, 0.000000000000000000, -150.0552959529999839 ) ) ;
#2113=CARTESIAN_POINT ( 'NONE',  ( 31.50000000000000000, -21.03620104879999886, -143.0552959529999839 ) ) ;
#2119=CARTESIAN_POINT ( 'NONE',  ( -15.78524365307783306, -45.92191803000493877, -150.0552959529999839 ) ) ;
#2124=EDGE_CURVE ( 'NONE', #12686, #10612, #4164, .T. ) ;
#2126=CARTESIAN_POINT ( 'NONE',  ( 13.24084097724026243, 23.82487805068920395, -150.0552959529999839 ) ) ;
#2134=AXIS2_PLACEMENT_3D ( 'NONE', #2956, #12223, #21048 ) ;
#2138=EDGE_CURVE ( 'NONE', #11594, #258, #11515, .T. ) ;
#2143=EDGE_CURVE ( 'NONE', #18702, #14446, #16539, .T. ) ;
#2146=VERTEX_POINT ( 'NONE', #20243 ) ;
#2148=CARTESIAN_POINT ( 'NONE',  ( 32.00000000000000000, -40.03620104880000241, -149.5552959529999839 ) ) ;
#2149=VERTEX_POINT ( 'NONE', #3934 ) ;
#2151=DIRECTION ( 'NONE',  ( 0.000000000000000000, -1.000000000000000000, 0.000000000000000000 ) ) ;
#2152=PLANE ( 'NONE',  #21239 ) ;
#2155=VERTEX_POINT ( 'NONE', #11170 ) ;
#2157=PLANE ( 'NONE',  #9509 ) ;
#2159=CARTESIAN_POINT ( 'NONE',  ( 0.000000000000000000, 19.50000000000000000, -150.0552959529999839 ) ) ;
#2170=CARTESIAN_POINT ( 'NONE',  ( 31.96891336220000213, -40.94938100119999547, -149.5552959529999839 ) ) ;
#2171=LINE ( 'NONE', #18112, #10515 ) ;
#2174=LINE ( 'NONE', #9984, #7127 ) ;
#2176=DIRECTION ( 'NONE',  ( -1.449507180940000069E-12, -1.705302565810000055E-12, 1.000000000000000000 ) ) ;
#2177=LINE ( 'NONE', #2525, #1223 ) ;
#2180=CIRCLE ( 'NONE', #20413, 2.999999999999999112 ) ;
#2183=LINE ( 'NONE', #515, #19455 ) ;
#2189=EDGE_CURVE ( 'NONE', #19467, #19419, #6288, .T. ) ;
#2205=LINE ( 'NONE', #3981, #8691 ) ;
#2206=ORIENTED_EDGE ( 'NONE', *, *, #20348, .T. ) ;
#2211=CYLINDRICAL_SURFACE ( 'NONE', #10765, 1.499999999999999556 ) ;
#2212=AXIS2_PLACEMENT_3D ( 'NONE', #7400, #20372, #18578 ) ;
#2223=LINE ( 'NONE', #4348, #16177 ) ;
#2226=CIRCLE ( 'NONE', #5252, 1.500000000000001332 ) ;
#2230=CARTESIAN_POINT ( 'NONE',  ( 4.750000000000000000, -47.00000000000000000, -150.0552959529999839 ) ) ;
#2231=ORIENTED_EDGE ( 'NONE', *, *, #16925, .F. ) ;
#2236=DIRECTION ( 'NONE',  ( 1.000000000000000000, 0.000000000000000000, 0.000000000000000000 ) ) ;
#2237=VERTEX_POINT ( 'NONE', #20696 ) ;
#2238=ADVANCED_FACE ( 'NONE', ( #11990 ), #3397, .T. ) ;
#2245=VECTOR ( 'NONE', #18530, 1000.000000000000000 ) ;
#2250=EDGE_CURVE ( 'NONE', #7971, #2516, #14233, .T. ) ;
#2253=VECTOR ( 'NONE', #14511, 1000.000000000000227 ) ;
#2264=EDGE_LOOP ( 'NONE', ( #18770, #22845, #17331, #9934 ) ) ;
#2268=CARTESIAN_POINT ( 'NONE',  ( 22.50000000000000000, 36.50000000000000000, -151.0552959529999839 ) ) ;
#2273=DIRECTION ( 'NONE',  ( 1.000000000000000000, 0.000000000000000000, 0.000000000000000000 ) ) ;
#2280=EDGE_CURVE ( 'NONE', #4867, #17914, #19704, .T. ) ;
#2293=AXIS2_PLACEMENT_3D ( 'NONE', #20911, #22681, #4836 ) ;
#2300=DIRECTION ( 'NONE',  ( 0.000000000000000000, 0.000000000000000000, 1.000000000000000000 ) ) ;
#2301=DIRECTION ( 'NONE',  ( -1.457985068979999943E-12, 1.723073263340000007E-12, 1.000000000000000000 ) ) ;
#2306=ADVANCED_FACE ( 'NONE', ( #4389 ), #11628, .F. ) ;
#2313=AXIS2_PLACEMENT_3D ( 'NONE', #12312, #21258, #12198 ) ;
#2319=ORIENTED_EDGE ( 'NONE', *, *, #6179, .T. ) ;
#2323=CARTESIAN_POINT ( 'NONE',  ( 19.04211518580000018, -51.50000000000000000, -150.0552959529999839 ) ) ;
#2333=ORIENTED_EDGE ( 'NONE', *, *, #4922, .F. ) ;
#2336=DIRECTION ( 'NONE',  ( -1.000000000000000000, 0.000000000000000000, 2.257453483404482811E-12 ) ) ;
#2345=DIRECTION ( 'NONE',  ( 1.000000000000000000, 0.000000000000000000, 0.000000000000000000 ) ) ;
#2346=DIRECTION ( 'NONE',  ( 0.000000000000000000, -1.000000000000000000, 0.000000000000000000 ) ) ;
#2351=CARTESIAN_POINT ( 'NONE',  ( 8.698929461718192258, -47.52072668388614574, -150.0552959530000123 ) ) ;
#2355=EDGE_LOOP ( 'NONE', ( #21561, #2696, #15045, #934, #13188, #21639, #9708, #5880 ) ) ;
#2362=EDGE_CURVE ( 'NONE', #14060, #11337, #12904, .T. ) ;
#2366=CARTESIAN_POINT ( 'NONE',  ( 18.95053822279999878, 51.50000000000000000, -149.5552959529999839 ) ) ;
#2367=DIRECTION ( 'NONE',  ( 0.7633862853691524286, -0.6459422414661293299, 0.000000000000000000 ) ) ;
#2372=CARTESIAN_POINT ( 'NONE',  ( 13.13369214859999978, 50.50000000000000000, -142.8052959529999839 ) ) ;
#2374=AXIS2_PLACEMENT_3D ( 'NONE', #3874, #20644, #11111 ) ;
#2382=ORIENTED_EDGE ( 'NONE', *, *, #1560, .F. ) ;
#2385=ORIENTED_EDGE ( 'NONE', *, *, #4992, .T. ) ;
#2389=CARTESIAN_POINT ( 'NONE',  ( -5.246523349696126104, 45.51000832343219571, -150.0552959530000123 ) ) ;
#2402=ADVANCED_FACE ( 'NONE', ( #21961 ), #2211, .F. ) ;
#2410=FACE_OUTER_BOUND ( 'NONE', #1741, .T. ) ;
#2417=CARTESIAN_POINT ( 'NONE',  ( -32.50000000000000000, -43.00000000000000000, -149.5552959529999839 ) ) ;
#2426=LINE ( 'NONE', #16805, #21069 ) ;
#2429=FACE_BOUND ( 'NONE', #16832, .T. ) ;
#2433=CARTESIAN_POINT ( 'NONE',  ( 1.133692148550000001, -51.50000000000000000, -136.5552959530000123 ) ) ;
#2435=PLANE ( 'NONE',  #1132 ) ;
#2443=EDGE_CURVE ( 'NONE', #22710, #23189, #3641, .T. ) ;
#2449=DIRECTION ( 'NONE',  ( 0.000000000000000000, 0.000000000000000000, 1.000000000000000000 ) ) ;
#2451=ORIENTED_EDGE ( 'NONE', *, *, #16184, .F. ) ;
#2452=CARTESIAN_POINT ( 'NONE',  ( 25.50000000000000000, 25.50000000000000000, -150.5552959529999839 ) ) ;
#2455=AXIS2_PLACEMENT_3D ( 'NONE', #5739, #10731, #23477 ) ;
#2459=EDGE_CURVE ( 'NONE', #3522, #17914, #14792, .T. ) ;
#2465=ORIENTED_EDGE ( 'NONE', *, *, #8630, .T. ) ;
#2472=CARTESIAN_POINT ( 'NONE',  ( -14.21475634692214740, -45.92191803000493877, -150.0552959529999839 ) ) ;
#2477=LINE ( 'NONE', #20215, #22509 ) ;
#2481=CARTESIAN_POINT ( 'NONE',  ( 4.500000000000000000, -3.500000000000000000, -145.5552959529999839 ) ) ;
#2483=ADVANCED_FACE ( 'NONE', ( #2557 ), #424, .T. ) ;
#2489=CARTESIAN_POINT ( 'NONE',  ( 19.13369214859999801, -51.50000000000000000, -143.0552959529999839 ) ) ;
#2491=ORIENTED_EDGE ( 'NONE', *, *, #19317, .F. ) ;
#2496=CARTESIAN_POINT ( 'NONE',  ( 25.31684607480000082, -45.26810052400000473, -149.5552959529999839 ) ) ;
#2497=FACE_OUTER_BOUND ( 'NONE', #23066, .T. ) ;
#2513=VERTEX_POINT ( 'NONE', #13485 ) ;
#2516=VERTEX_POINT ( 'NONE', #22303 ) ;
#2518=LINE ( 'NONE', #14890, #203 ) ;
#2524=DIRECTION ( 'NONE',  ( 0.000000000000000000, 0.000000000000000000, 1.000000000000000000 ) ) ;
#2525=CARTESIAN_POINT ( 'NONE',  ( -4.500000000000000000, 0.000000000000000000, -150.0552959529999839 ) ) ;
#2532=CARTESIAN_POINT ( 'NONE',  ( 6.000000000000000000, -3.500000000000000000, -140.0552959529999839 ) ) ;
#2537=ORIENTED_EDGE ( 'NONE', *, *, #5328, .F. ) ;
#2541=DIRECTION ( 'NONE',  ( 0.000000000000000000, 1.000000000000000000, 0.000000000000000000 ) ) ;
#2546=CARTESIAN_POINT ( 'NONE',  ( -7.500000000000000000, 42.50000000000000000, -150.5552959529999839 ) ) ;
#2549=EDGE_CURVE ( 'NONE', #21164, #3612, #9668, .T. ) ;
#2557=FACE_OUTER_BOUND ( 'NONE', #10683, .T. ) ;
#2566=AXIS2_PLACEMENT_3D ( 'NONE', #21950, #11323, #3862 ) ;
#2578=EDGE_LOOP ( 'NONE', ( #16493, #15663, #9579, #17088 ) ) ;
#2581=LINE ( 'NONE', #22565, #7194 ) ;
#2583=ORIENTED_EDGE ( 'NONE', *, *, #15352, .F. ) ;
#2605=ORIENTED_EDGE ( 'NONE', *, *, #15186, .F. ) ;
#2607=CARTESIAN_POINT ( 'NONE',  ( 31.50000000020000002, -40.03620104850000416, -136.0552959530000123 ) ) ;
#2620=VECTOR ( 'NONE', #14874, 1000.000000000000000 ) ;
#2624=VERTEX_POINT ( 'NONE', #15862 ) ;
#2631=VECTOR ( 'NONE', #11038, 1000.000000000000000 ) ;
#2638=DIRECTION ( 'NONE',  ( -0.4567501391959232770, -0.5397956190499111351, 0.7071067811858601226 ) ) ;
#2640=CARTESIAN_POINT ( 'NONE',  ( -16.50000000000000000, -43.00000000000000000, -150.0552959529999839 ) ) ;
#2642=VECTOR ( 'NONE', #3185, 1000.000000000000000 ) ;
#2648=DIRECTION ( 'NONE',  ( 1.000000000000000000, 0.000000000000000000, 0.000000000000000000 ) ) ;
#2651=ORIENTED_EDGE ( 'NONE', *, *, #18429, .F. ) ;
#2658=CIRCLE ( 'NONE', #13264, 7.499999999999999112 ) ;
#2662=ORIENTED_EDGE ( 'NONE', *, *, #9008, .T. ) ;
#2668=DIRECTION ( 'NONE',  ( -1.000000000000000000, 0.000000000000000000, 0.000000000000000000 ) ) ;
#2669=EDGE_CURVE ( 'NONE', #9439, #4983, #11932, .T. ) ;
#2670=CARTESIAN_POINT ( 'NONE',  ( 9.736704675116099494, -36.41257638424534093, -150.0552959529999555 ) ) ;
#2679=ADVANCED_FACE ( 'NONE', ( #15987 ), #21468, .F. ) ;
#2690=AXIS2_PLACEMENT_3D ( 'NONE', #6355, #904, #19094 ) ;
#2691=DIRECTION ( 'NONE',  ( 0.000000000000000000, -1.000000000000000000, 0.000000000000000000 ) ) ;
#2693=DIRECTION ( 'NONE',  ( -1.000000000000000000, 0.000000000000000000, 0.000000000000000000 ) ) ;
#2696=ORIENTED_EDGE ( 'NONE', *, *, #1439, .T. ) ;
#2697=CARTESIAN_POINT ( 'NONE',  ( 31.00000000000000000, -39.80430157320000006, -150.0552959529999839 ) ) ;
#2699=ORIENTED_EDGE ( 'NONE', *, *, #22898, .F. ) ;
#2701=CARTESIAN_POINT ( 'NONE',  ( -15.00000000000000000, -43.00000000000000000, -145.5552959529999839 ) ) ;
#2707=VECTOR ( 'NONE', #21869, 1000.000000000000000 ) ;
#2708=VECTOR ( 'NONE', #16689, 1000.000000000000000 ) ;
#2720=VECTOR ( 'NONE', #5141, 1000.000000000000000 ) ;
#2733=ORIENTED_EDGE ( 'NONE', *, *, #21429, .T. ) ;
#2742=ORIENTED_EDGE ( 'NONE', *, *, #7932, .T. ) ;
#2743=CARTESIAN_POINT ( 'NONE',  ( -32.50000000000000000, -51.00000000000000000, -149.5552959529999839 ) ) ;
#2745=VECTOR ( 'NONE', #15481, 1000.000000000000000 ) ;
#2751=CARTESIAN_POINT ( 'NONE',  ( 7.500000000000000888, -3.107300918301275416, -150.0552959530000123 ) ) ;
#2755=EDGE_CURVE ( 'NONE', #16273, #2844, #19674, .T. ) ;
#2756=CARTESIAN_POINT ( 'NONE',  ( 19.04211518569999839, -51.50000000000000000, -150.0552959529999839 ) ) ;
#2761=AXIS2_PLACEMENT_3D ( 'NONE', #16975, #2023, #14961 ) ;
#2762=PLANE ( 'NONE',  #20444 ) ;
#2765=ORIENTED_EDGE ( 'NONE', *, *, #16235, .F. ) ;
#2771=ORIENTED_EDGE ( 'NONE', *, *, #225, .T. ) ;
#2774=CARTESIAN_POINT ( 'NONE',  ( -32.50000000000000000, 19.50000000020000002, -137.0552959530000123 ) ) ;
#2777=CARTESIAN_POINT ( 'NONE',  ( 32.00000000000000000, 40.03620104880000241, -136.0552959530000123 ) ) ;
#2782=CARTESIAN_POINT ( 'NONE',  ( 20.50000000000000000, -20.50000000000000000, -150.0552959529999839 ) ) ;
#2783=PLANE ( 'NONE',  #9361 ) ;
#2786=EDGE_CURVE ( 'NONE', #3754, #16830, #16459, .T. ) ;
#2790=( NAMED_UNIT ( * ) SI_UNIT ( $, .STERADIAN. ) SOLID_ANGLE_UNIT ( ) );
#2807=ORIENTED_EDGE ( 'NONE', *, *, #8060, .T. ) ;
#2812=ADVANCED_FACE ( 'NONE', ( #10845 ), #5397, .T. ) ;
#2817=CARTESIAN_POINT ( 'NONE',  ( 8.750000000000000000, -40.23606797749999942, -150.5552959529999839 ) ) ;
#2828=LINE ( 'NONE', #17456, #18607 ) ;
#2838=LINE ( 'NONE', #15334, #10249 ) ;
#2839=CARTESIAN_POINT ( 'NONE',  ( 21.10099947280546218, -22.34364015992474961, -150.0552959529999839 ) ) ;
#2844=VERTEX_POINT ( 'NONE', #18013 ) ;
#2848=DIRECTION ( 'NONE',  ( -0.7071067811865474617, 0.7071067811865476838, 0.000000000000000000 ) ) ;
#2850=ORIENTED_EDGE ( 'NONE', *, *, #14751, .F. ) ;
#2851=CARTESIAN_POINT ( 'NONE',  ( 0.000000000000000000, -36.00000000000000000, -150.0552959529999839 ) ) ;
#2855=EDGE_CURVE ( 'NONE', #21958, #6865, #16226, .T. ) ;
#2856=LINE ( 'NONE', #3096, #10200 ) ;
#2857=VECTOR ( 'NONE', #7846, 1000.000000000000000 ) ;
#2870=CARTESIAN_POINT ( 'NONE',  ( -14.24276452920772051, -41.69048151115483591, -150.0552959529999839 ) ) ;
#2875=ORIENTED_EDGE ( 'NONE', *, *, #22649, .F. ) ;
#2884=DIRECTION ( 'NONE',  ( 0.000000000000000000, 1.000000000000000000, 0.000000000000000000 ) ) ;
#2891=LINE ( 'NONE', #2777, #9448 ) ;
#2893=CARTESIAN_POINT ( 'NONE',  ( -12.50000000000000000, 0.000000000000000000, -150.0552959529999839 ) ) ;
#2897=CARTESIAN_POINT ( 'NONE',  ( -0.009529796614447350739, 16.74243713058418237, -150.0552959529999839 ) ) ;
#2900=CARTESIAN_POINT ( 'NONE',  ( 5.519240656394276634, 27.95201674008764314, -150.0552959530000123 ) ) ;
#2901=CARTESIAN_POINT ( 'NONE',  ( 5.569521322412388287, -33.22557888555225247, -150.0552959530000123 ) ) ;
#2902=ORIENTED_EDGE ( 'NONE', *, *, #9008, .F. ) ;
#2906=AXIS2_PLACEMENT_3D ( 'NONE', #23201, #23316, #21540 ) ;
#2912=EDGE_CURVE ( 'NONE', #1217, #4350, #11196, .T. ) ;
#2918=DIRECTION ( 'NONE',  ( 1.000000000000000000, 0.000000000000000000, 0.000000000000000000 ) ) ;
#2920=CARTESIAN_POINT ( 'NONE',  ( -31.00000000000000000, 19.50000000000000000, -150.5552959529999839 ) ) ;
#2921=VECTOR ( 'NONE', #13977, 1000.000000000000000 ) ;
#2930=DIRECTION ( 'NONE',  ( 1.000000000000000000, 0.000000000000000000, 0.000000000000000000 ) ) ;
#2941=EDGE_CURVE ( 'NONE', #1936, #19224, #9535, .T. ) ;
#2948=CARTESIAN_POINT ( 'NONE',  ( -4.500000000000000000, 37.00000000000000000, -151.0552959529999839 ) ) ;
#2949=VERTEX_POINT ( 'NONE', #11435 ) ;
#2956=CARTESIAN_POINT ( 'NONE',  ( 19.91945158500000090, -51.14507942810000429, -149.5552959529999839 ) ) ;
#2962=CARTESIAN_POINT ( 'NONE',  ( 6.500000000000000000, 13.00000000000000000, -150.5552959529999839 ) ) ;
#2971=DIRECTION ( 'NONE',  ( 0.000000000000000000, 0.000000000000000000, -1.000000000000000000 ) ) ;
#2972=EDGE_LOOP ( 'NONE', ( #3946, #14498, #19451, #3090 ) ) ;
#2975=VECTOR ( 'NONE', #13953, 1000.000000000000000 ) ;
#2977=CIRCLE ( 'NONE', #16272, 1.499999999999999556 ) ;
#2979=EDGE_CURVE ( 'NONE', #9664, #21739, #2426, .T. ) ;
#2981=CARTESIAN_POINT ( 'NONE',  ( 4.892699081698721919, -0.4999999999999995559, -150.0552959529999839 ) ) ;
#2985=ORIENTED_EDGE ( 'NONE', *, *, #5466, .T. ) ;
#2989=EDGE_CURVE ( 'NONE', #7959, #22754, #17153, .T. ) ;
#2990=CARTESIAN_POINT ( 'NONE',  ( 25.34364015992474961, -18.10099947280545862, -150.0552959529999839 ) ) ;
#3004=DIRECTION ( 'NONE',  ( 0.000000000000000000, 0.000000000000000000, 1.000000000000000000 ) ) ;
#3007=PLANE ( 'NONE',  #19489 ) ;
#3008=DIRECTION ( 'NONE',  ( 1.000000000000000000, 0.000000000000000000, 0.000000000000000000 ) ) ;
#3020=CARTESIAN_POINT ( 'NONE',  ( -15.00000000000000000, -43.00000000000000000, -140.0552959529999839 ) ) ;
#3026=CARTESIAN_POINT ( 'NONE',  ( 5.298801200312091453, -33.35703351611178391, -150.0552959530000123 ) ) ;
#3028=ORIENTED_EDGE ( 'NONE', *, *, #20273, .F. ) ;
#3035=CARTESIAN_POINT ( 'NONE',  ( 25.96278831570000278, 46.03148680969999873, -136.0552959530000123 ) ) ;
#3037=VERTEX_POINT ( 'NONE', #2532 ) ;
#3050=DIRECTION ( 'NONE',  ( -1.000000000000000000, 2.312964634635743450E-15, 0.000000000000000000 ) ) ;
#3053=AXIS2_PLACEMENT_3D ( 'NONE', #16643, #5930, #3928 ) ;
#3074=CARTESIAN_POINT ( 'NONE',  ( 25.42349012524837093, 35.71905350741751306, -150.0552959529999839 ) ) ;
#3081=DIRECTION ( 'NONE',  ( 1.000000000000000000, 0.000000000000000000, 0.000000000000000000 ) ) ;
#3090=ORIENTED_EDGE ( 'NONE', *, *, #2989, .F. ) ;
#3093=EDGE_LOOP ( 'NONE', ( #12559, #10314, #22259, #7596 ) ) ;
#3096=CARTESIAN_POINT ( 'NONE',  ( 25.94418247360000152, 46.04723021459999899, -149.5552959529999839 ) ) ;
#3099=VECTOR ( 'NONE', #12871, 1000.000000000000227 ) ;
#3101=DIRECTION ( 'NONE',  ( 0.6459422414661292189, -0.7633862853691524286, 2.257144641400451094E-12 ) ) ;
#3105=ORIENTED_EDGE ( 'NONE', *, *, #4201, .F. ) ;
#3108=LINE ( 'NONE', #8550, #3259 ) ;
#3110=CARTESIAN_POINT ( 'NONE',  ( 26.12135916506276345, -18.98914305888729714, -150.0552959530000123 ) ) ;
#3111=PLANE ( 'NONE',  #18615 ) ;
#3112=DIRECTION ( 'NONE',  ( 0.000000000000000000, -1.000000000000000000, 0.000000000000000000 ) ) ;
#3117=CIRCLE ( 'NONE', #19457, 1.500000000000000444 ) ;
#3119=CARTESIAN_POINT ( 'NONE',  ( -31.00000000000000000, -50.00000000000000000, -151.0552959529999839 ) ) ;
#3120=ADVANCED_FACE ( 'NONE', ( #13826 ), #3123, .F. ) ;
#3123=PLANE ( 'NONE',  #22201 ) ;
#3125=DIRECTION ( 'NONE',  ( -2.257144641399999941E-12, 0.000000000000000000, 1.000000000000000000 ) ) ;
#3131=ORIENTED_EDGE ( 'NONE', *, *, #1335, .T. ) ;
#3135=CYLINDRICAL_SURFACE ( 'NONE', #3654, 7.500000000000005329 ) ;
#3137=CARTESIAN_POINT ( 'NONE',  ( 19.13369214879999802, 50.49999999980000354, -136.0552959530000123 ) ) ;
#3138=VERTEX_POINT ( 'NONE', #4897 ) ;
#3140=CARTESIAN_POINT ( 'NONE',  ( -0.2409605966970265190, 23.82477348803106310, -150.0552959529999839 ) ) ;
#3143=ORIENTED_EDGE ( 'NONE', *, *, #15508, .F. ) ;
#3153=DIRECTION ( 'NONE',  ( 0.000000000000000000, 1.000000000000000000, 0.000000000000000000 ) ) ;
#3158=CARTESIAN_POINT ( 'NONE',  ( 18.66051412330858383, 24.90191174486891867, -150.0552959529999839 ) ) ;
#3160=PLANE ( 'NONE',  #3671 ) ;
#3163=DIRECTION ( 'NONE',  ( 1.000000000000000000, 0.000000000000000000, -2.257157423930000049E-12 ) ) ;
#3167=VERTEX_POINT ( 'NONE', #11782 ) ;
#3171=PLANE ( 'NONE',  #18577 ) ;
#3172=LINE ( 'NONE', #13873, #5388 ) ;
#3174=EDGE_LOOP ( 'NONE', ( #2231, #8769, #20425, #47 ) ) ;
#3175=DIRECTION ( 'NONE',  ( 0.000000000000000000, 0.000000000000000000, 1.000000000000000000 ) ) ;
#3183=DIRECTION ( 'NONE',  ( 0.000000000000000000, 0.000000000000000000, 1.000000000000000000 ) ) ;
#3184=EDGE_CURVE ( 'NONE', #7540, #21170, #14994, .T. ) ;
#3185=DIRECTION ( 'NONE',  ( 0.000000000000000000, 0.000000000000000000, 1.000000000000000000 ) ) ;
#3191=CYLINDRICAL_SURFACE ( 'NONE', #10849, 1.500000000000001332 ) ;
#3203=VERTEX_POINT ( 'NONE', #6440 ) ;
#3208=ORIENTED_EDGE ( 'NONE', *, *, #20168, .T. ) ;
#3209=DIRECTION ( 'NONE',  ( 2.257144641399999941E-12, 0.000000000000000000, 1.000000000000000000 ) ) ;
#3210=EDGE_CURVE ( 'NONE', #13163, #3680, #12023, .T. ) ;
#3213=FACE_OUTER_BOUND ( 'NONE', #8069, .T. ) ;
#3217=EDGE_LOOP ( 'NONE', ( #985, #5840, #3336, #1391 ) ) ;
#3219=DIRECTION ( 'NONE',  ( 2.326943610902514898E-15, 0.000000000000000000, 1.000000000000000000 ) ) ;
#3221=CARTESIAN_POINT ( 'NONE',  ( 32.50000000000000000, 32.96379895120000469, -137.0552959530000123 ) ) ;
#3227=FACE_OUTER_BOUND ( 'NONE', #13579, .T. ) ;
#3231=ADVANCED_FACE ( 'NONE', ( #10237 ), #13934, .F. ) ;
#3232=DIRECTION ( 'NONE',  ( 0.000000000000000000, 0.000000000000000000, 1.000000000000000000 ) ) ;
#3233=CARTESIAN_POINT ( 'NONE',  ( 32.50000000000000000, 20.96379895120000114, -136.0552959530000123 ) ) ;
#3235=VERTEX_POINT ( 'NONE', #10937 ) ;
#3240=DIRECTION ( 'NONE',  ( 1.000000000000000000, 0.000000000000000000, -2.257453483404485639E-12 ) ) ;
#3250=( NAMED_UNIT ( * ) PLANE_ANGLE_UNIT ( ) SI_UNIT ( $, .RADIAN. ) );
#3252=EDGE_LOOP ( 'NONE', ( #15305, #13897, #15340, #2662 ) ) ;
#3259=VECTOR ( 'NONE', #12128, 1000.000000000000000 ) ;
#3263=DIRECTION ( 'NONE',  ( 0.000000000000000000, 0.000000000000000000, -1.000000000000000000 ) ) ;
#3264=DIRECTION ( 'NONE',  ( 2.257144641399999941E-12, 0.000000000000000000, 1.000000000000000000 ) ) ;
#3273=VECTOR ( 'NONE', #14136, 1000.000000000000000 ) ;
#3285=CARTESIAN_POINT ( 'NONE',  ( -7.500000000000000000, 19.50000000000000000, -150.0552959529999839 ) ) ;
#3292=ADVANCED_BREP_SHAPE_REPRESENTATION ( '', ( #11774, #5025 ), #8794 ) ;
#3293=VERTEX_POINT ( 'NONE', #26 ) ;
#3301=CARTESIAN_POINT ( 'NONE',  ( -6.683153925719999222, 51.50000000000000000, -150.0552959529999839 ) ) ;
#3302=FACE_OUTER_BOUND ( 'NONE', #3780, .T. ) ;
#3306=ORIENTED_EDGE ( 'NONE', *, *, #1983, .F. ) ;
#3317=CARTESIAN_POINT ( 'NONE',  ( 4.750000000000000000, -47.00000000000000000, -151.0552959529999839 ) ) ;
#3319=ORIENTED_EDGE ( 'NONE', *, *, #17732, .F. ) ;
#3320=CARTESIAN_POINT ( 'NONE',  ( -2.979194667911468919, 46.44907581354189574, -150.0552959529999839 ) ) ;
#3321=AXIS2_PLACEMENT_3D ( 'NONE', #2489, #20926, #17221 ) ;
#3328=ORIENTED_EDGE ( 'NONE', *, *, #16339, .T. ) ;
#3331=FACE_BOUND ( 'NONE', #9585, .T. ) ;
#3334=EDGE_CURVE ( 'NONE', #4867, #6268, #5596, .T. ) ;
#3335=DIRECTION ( 'NONE',  ( 0.000000000000000000, 1.000000000000000000, 0.000000000000000000 ) ) ;
#3336=ORIENTED_EDGE ( 'NONE', *, *, #4732, .T. ) ;
#3345=EDGE_LOOP ( 'NONE', ( #21709, #3988, #14253, #8703 ) ) ;
#3351=LINE ( 'NONE', #6926, #20502 ) ;
#3354=AXIS2_PLACEMENT_3D ( 'NONE', #14225, #21490, #20149 ) ;
#3357=ORIENTED_EDGE ( 'NONE', *, *, #12944, .T. ) ;
#3361=CARTESIAN_POINT ( 'NONE',  ( 31.50000000000000000, 39.80430157320000006, -143.0552959529999839 ) ) ;
#3365=FACE_OUTER_BOUND ( 'NONE', #8140, .T. ) ;
#3371=VECTOR ( 'NONE', #1048, 1000.000000000000000 ) ;
#3372=ORIENTED_EDGE ( 'NONE', *, *, #17087, .F. ) ;
#3374=FACE_OUTER_BOUND ( 'NONE', #13985, .T. ) ;
#3380=CARTESIAN_POINT ( 'NONE',  ( 17.49993271304850140, 22.89748944252527352, -150.0552959529999839 ) ) ;
#3381=CARTESIAN_POINT ( 'NONE',  ( -16.50000000000000000, -43.00000000000000000, -150.0552959529999839 ) ) ;
#3384=FACE_OUTER_BOUND ( 'NONE', #20907, .T. ) ;
#3389=EDGE_CURVE ( 'NONE', #19876, #11512, #16315, .T. ) ;
#3390=ORIENTED_EDGE ( 'NONE', *, *, #1097, .F. ) ;
#3392=VECTOR ( 'NONE', #6509, 1000.000000000000000 ) ;
#3394=DIRECTION ( 'NONE',  ( 0.000000000000000000, 1.000000000000000000, 0.000000000000000000 ) ) ;
#3397=PLANE ( 'NONE',  #22069 ) ;
#3400=EDGE_CURVE ( 'NONE', #11681, #10143, #23337, .T. ) ;
#3411=CIRCLE ( 'NONE', #22403, 0.5000000000000004441 ) ;
#3417=CARTESIAN_POINT ( 'NONE',  ( 0.8371776177479999248, 14.00000000000000000, -144.0552959529999839 ) ) ;
#3419=EDGE_CURVE ( 'NONE', #16273, #6526, #18796, .T. ) ;
#3421=PLANE ( 'NONE',  #5734 ) ;
#3426=CARTESIAN_POINT ( 'NONE',  ( 25.34364015992475316, -22.89900052719453427, -150.0552959529999839 ) ) ;
#3430=ORIENTED_EDGE ( 'NONE', *, *, #2459, .T. ) ;
#3431=VECTOR ( 'NONE', #23044, 1000.000000000000000 ) ;
#3437=CARTESIAN_POINT ( 'NONE',  ( -31.50000000000000000, 1.000000000000000000, -149.5552959529999839 ) ) ;
#3438=ORIENTED_EDGE ( 'NONE', *, *, #1335, .F. ) ;
#3439=CARTESIAN_POINT ( 'NONE',  ( -32.50000000000000000, 19.50000000000000000, -150.5552959529999839 ) ) ;
#3448=VECTOR ( 'NONE', #5360, 1000.000000000000227 ) ;
#3449=AXIS2_PLACEMENT_3D ( 'NONE', #17447, #1176, #12437 ) ;
#3451=EDGE_CURVE ( 'NONE', #1104, #565, #16656, .T. ) ;
#3455=LINE ( 'NONE', #8662, #6371 ) ;
#3464=DIRECTION ( 'NONE',  ( 0.000000000000000000, -1.000000000000000000, -2.257144641399999941E-12 ) ) ;
#3476=ORIENTED_EDGE ( 'NONE', *, *, #4659, .T. ) ;
#3492=EDGE_LOOP ( 'NONE', ( #4975, #17946, #1517, #5112 ) ) ;
#3506=CARTESIAN_POINT ( 'NONE',  ( 20.10199673422639322, 25.50000000000000355, -150.0552959529999839 ) ) ;
#3513=DIRECTION ( 'NONE',  ( 0.000000000000000000, -1.000000000000000000, -2.273736754430000208E-12 ) ) ;
#3514=CARTESIAN_POINT ( 'NONE',  ( 22.50000000000000000, 36.50000000000000000, -150.0552959529999839 ) ) ;
#3515=CARTESIAN_POINT ( 'NONE',  ( 32.05742780220000299, -40.87448416729999678, -150.0552959529999839 ) ) ;
#3520=EDGE_CURVE ( 'NONE', #3906, #16283, #8539, .T. ) ;
#3522=VERTEX_POINT ( 'NONE', #15348 ) ;
#3524=DIRECTION ( 'NONE',  ( 0.6459422414661339928, -0.7633862853691482098, 0.000000000000000000 ) ) ;
#3527=VERTEX_POINT ( 'NONE', #21181 ) ;
#3528=DIRECTION ( 'NONE',  ( 1.000000000000000000, 0.000000000000000000, 0.000000000000000000 ) ) ;
#3531=DIRECTION ( 'NONE',  ( -0.000000000000000000, 1.000000000000000000, 0.000000000000000000 ) ) ;
#3537=EDGE_CURVE ( 'NONE', #19834, #8510, #4749, .T. ) ;
#3539=DIRECTION ( 'NONE',  ( 0.000000000000000000, -1.000000000000000000, 0.000000000000000000 ) ) ;
#3541=EDGE_LOOP ( 'NONE', ( #20081, #14631, #21867, #7152 ) ) ;
#3542=PRODUCT_DEFINITION ( 'UNKNOWN', '', #9995, #14687 ) ;
#3546=CARTESIAN_POINT ( 'NONE',  ( 0.000000000000000000, 0.000000000000000000, -140.0552959529999839 ) ) ;
#3550=CARTESIAN_POINT ( 'NONE',  ( -31.50000000000000000, 16.00000000000000000, -144.0552959529999839 ) ) ;
#3560=DIRECTION ( 'NONE',  ( 0.000000000000000000, -1.000000000000000000, 0.000000000000000000 ) ) ;
#3562=DIRECTION ( 'NONE',  ( 0.000000000000000000, 1.000000000000000000, 0.000000000000000000 ) ) ;
#3563=ORIENTED_EDGE ( 'NONE', *, *, #11008, .F. ) ;
#3566=ORIENTED_EDGE ( 'NONE', *, *, #15586, .F. ) ;
#3569=EDGE_CURVE ( 'NONE', #4645, #232, #1205, .T. ) ;
#3576=CARTESIAN_POINT ( 'NONE',  ( 0.000000000000000000, 0.000000000000000000, -151.0552959529999839 ) ) ;
#3579=CARTESIAN_POINT ( 'NONE',  ( -18.00000000000000000, -43.00000000000000000, -150.0552959529999839 ) ) ;
#3580=ORIENTED_EDGE ( 'NONE', *, *, #9946, .F. ) ;
#3590=AXIS2_PLACEMENT_3D ( 'NONE', #3035, #1363, #23249 ) ;
#3594=EDGE_LOOP ( 'NONE', ( #1608, #16064, #8873, #5714 ) ) ;
#3608=DIRECTION ( 'NONE',  ( 0.000000000000000000, 0.000000000000000000, 1.000000000000000000 ) ) ;
#3612=VERTEX_POINT ( 'NONE', #19261 ) ;
#3616=ORIENTED_EDGE ( 'NONE', *, *, #980, .F. ) ;
#3619=ORIENTED_EDGE ( 'NONE', *, *, #22626, .F. ) ;
#3623=AXIS2_PLACEMENT_3D ( 'NONE', #5109, #21895, #23434 ) ;
#3635=ORIENTED_EDGE ( 'NONE', *, *, #14869, .T. ) ;
#3641=LINE ( 'NONE', #10875, #21424 ) ;
#3643=CARTESIAN_POINT ( 'NONE',  ( -7.500000000000000000, 25.50000000000000000, -150.0552959529999839 ) ) ;
#3646=DIRECTION ( 'NONE',  ( -0.7633862853691524286, -0.6459422414661293299, 5.800915303671162679E-15 ) ) ;
#3654=AXIS2_PLACEMENT_3D ( 'NONE', #17640, #11920, #8468 ) ;
#3671=AXIS2_PLACEMENT_3D ( 'NONE', #4699, #3264, #14213 ) ;
#3673=ORIENTED_EDGE ( 'NONE', *, *, #18818, .F. ) ;
#3679=DIRECTION ( 'NONE',  ( 0.000000000000000000, 1.000000000000000000, 0.000000000000000000 ) ) ;
#3680=VERTEX_POINT ( 'NONE', #19031 ) ;
#3692=CARTESIAN_POINT ( 'NONE',  ( -31.00000000000000000, -51.50000000000000000, -149.5552959529999839 ) ) ;
#3693=CYLINDRICAL_SURFACE ( 'NONE', #3750, 1.500000000000001554 ) ;
#3694=ADVANCED_FACE ( 'NONE', ( #4639 ), #20947, .T. ) ;
#3704=CARTESIAN_POINT ( 'NONE',  ( -31.50000000000000000, 12.00000000000000000, -144.0552959529999839 ) ) ;
#3705=ORIENTED_EDGE ( 'NONE', *, *, #12699, .T. ) ;
#3711=EDGE_CURVE ( 'NONE', #11278, #1062, #5569, .T. ) ;
#3718=FACE_OUTER_BOUND ( 'NONE', #13500, .T. ) ;
#3721=DIRECTION ( 'NONE',  ( 1.000000000000000000, 0.000000000000000000, 2.257144641399999941E-12 ) ) ;
#3736=CARTESIAN_POINT ( 'NONE',  ( -14.08020845438083235, -44.20076496858382598, -150.0552959529999839 ) ) ;
#3743=LINE ( 'NONE', #10983, #16613 ) ;
#3744=DIRECTION ( 'NONE',  ( -1.000000000000000000, 0.000000000000000000, 0.000000000000000000 ) ) ;
#3750=AXIS2_PLACEMENT_3D ( 'NONE', #11052, #21795, #7139 ) ;
#3753=CARTESIAN_POINT ( 'NONE',  ( 32.50000000000000000, 20.96379895120000114, -136.0552959530000123 ) ) ;
#3754=VERTEX_POINT ( 'NONE', #3317 ) ;
#3756=ORIENTED_EDGE ( 'NONE', *, *, #1371, .T. ) ;
#3763=ORIENTED_EDGE ( 'NONE', *, *, #6126, .F. ) ;
#3768=AXIS2_PLACEMENT_3D ( 'NONE', #1000, #22644, #13718 ) ;
#3773=VECTOR ( 'NONE', #3539, 1000.000000000000000 ) ;
#3774=DIRECTION ( 'NONE',  ( 1.000000000000000000, 0.000000000000000000, 0.000000000000000000 ) ) ;
#3780=EDGE_LOOP ( 'NONE', ( #4972, #20052 ) ) ;
#3789=VECTOR ( 'NONE', #16063, 1000.000000000000000 ) ;
#3793=AXIS2_PLACEMENT_3D ( 'NONE', #17478, #19145, #2848 ) ;
#3794=CARTESIAN_POINT ( 'NONE',  ( 32.50000000000000000, 0.000000000000000000, -136.0552959530000123 ) ) ;
#3796=DIRECTION ( 'NONE',  ( 0.000000000000000000, 1.000000000000000000, 0.000000000000000000 ) ) ;
#3797=VERTEX_POINT ( 'NONE', #10907 ) ;
#3799=ADVANCED_FACE ( 'NONE', ( #10438 ), #19744, .T. ) ;
#3803=CARTESIAN_POINT ( 'NONE',  ( 4.109450702737304617, -4.961822747171590997, -150.0552959529999839 ) ) ;
#3807=ORIENTED_EDGE ( 'NONE', *, *, #13030, .T. ) ;
#3812=FACE_BOUND ( 'NONE', #21940, .T. ) ;
#3820=CARTESIAN_POINT ( 'NONE',  ( -13.86630785140000022, -50.50000000000000000, -143.0552959529999839 ) ) ;
#3824=ORIENTED_EDGE ( 'NONE', *, *, #18377, .T. ) ;
#3843=VECTOR ( 'NONE', #20387, 1000.000000000000000 ) ;
#3846=DIRECTION ( 'NONE',  ( -0.6459422414661291079, -0.7633862853691523176, -2.273736754430455399E-12 ) ) ;
#3848=CARTESIAN_POINT ( 'NONE',  ( 4.750000000000000000, -47.00000000000000000, -150.5552959529999839 ) ) ;
#3850=ORIENTED_EDGE ( 'NONE', *, *, #225, .F. ) ;
#3853=LINE ( 'NONE', #4321, #2708 ) ;
#3861=DIRECTION ( 'NONE',  ( 0.000000000000000000, -1.000000000000000000, 0.000000000000000000 ) ) ;
#3862=DIRECTION ( 'NONE',  ( 0.000000000000000000, 0.000000000000000000, -1.000000000000000000 ) ) ;
#3863=LINE ( 'NONE', #5286, #18515 ) ;
#3870=VERTEX_POINT ( 'NONE', #22336 ) ;
#3874=CARTESIAN_POINT ( 'NONE',  ( 31.00000000000000000, 39.80430157320000006, -149.5552959529999839 ) ) ;
#3878=VECTOR ( 'NONE', #18845, 1000.000000000000000 ) ;
#3885=DIRECTION ( 'NONE',  ( 0.000000000000000000, 0.000000000000000000, 1.000000000000000000 ) ) ;
#3889=EDGE_CURVE ( 'NONE', #565, #13650, #5798, .T. ) ;
#3892=FACE_OUTER_BOUND ( 'NONE', #11757, .T. ) ;
#3893=ORIENTED_EDGE ( 'NONE', *, *, #14106, .T. ) ;
#3904=LINE ( 'NONE', #682, #19720 ) ;
#3905=VERTEX_POINT ( 'NONE', #15199 ) ;
#3906=VERTEX_POINT ( 'NONE', #457 ) ;
#3910=CARTESIAN_POINT ( 'NONE',  ( 12.46241645105735607, 25.07592078380848477, -150.0552959529999839 ) ) ;
#3928=DIRECTION ( 'NONE',  ( 1.000000000000000000, 0.000000000000000000, 0.000000000000000000 ) ) ;
#3934=CARTESIAN_POINT ( 'NONE',  ( 20.50000000000000000, 25.50000000000000000, -150.0552959529999839 ) ) ;
#3938=EDGE_CURVE ( 'NONE', #9007, #12574, #4130, .T. ) ;
#3941=LINE ( 'NONE', #9383, #5278 ) ;
#3945=VECTOR ( 'NONE', #16254, 1000.000000000000000 ) ;
#3946=ORIENTED_EDGE ( 'NONE', *, *, #12869, .F. ) ;
#3951=DIRECTION ( 'NONE',  ( -2.252420472359999842E-12, 0.000000000000000000, 1.000000000000000000 ) ) ;
#3959=EDGE_CURVE ( 'NONE', #23250, #15992, #333, .T. ) ;
#3965=ORIENTED_EDGE ( 'NONE', *, *, #7207, .F. ) ;
#3968=DIRECTION ( 'NONE',  ( 0.7071067811870332953, 0.000000000000000000, 0.7071067811860618502 ) ) ;
#3981=CARTESIAN_POINT ( 'NONE',  ( -4.500000000000000000, 34.00000000000000000, -150.5552959529999839 ) ) ;
#3982=ORIENTED_EDGE ( 'NONE', *, *, #17873, .T. ) ;
#3988=ORIENTED_EDGE ( 'NONE', *, *, #13351, .T. ) ;
#3991=VECTOR ( 'NONE', #18606, 1000.000000000000000 ) ;
#3999=CARTESIAN_POINT ( 'NONE',  ( -32.50000000000000000, 50.00000000000000000, -149.5552959529999839 ) ) ;
#4004=CARTESIAN_POINT ( 'NONE',  ( 8.250000000000000000, -42.23606797749999942, -151.0552959529999839 ) ) ;
#4007=CARTESIAN_POINT ( 'NONE',  ( 7.750000000000000000, -41.23606797749999942, -151.0552959529999839 ) ) ;
#4015=CARTESIAN_POINT ( 'NONE',  ( -17.39900052719453072, -44.84364015992474606, -150.0552959529999555 ) ) ;
#4020=CARTESIAN_POINT ( 'NONE',  ( -31.00000000000000000, -36.00000000000000000, -149.5552959529999839 ) ) ;
#4029=ORIENTED_EDGE ( 'NONE', *, *, #12431, .T. ) ;
#4030=DIRECTION ( 'NONE',  ( 0.000000000000000000, 0.000000000000000000, 1.000000000000000000 ) ) ;
#4038=VERTEX_POINT ( 'NONE', #23046 ) ;
#4044=CIRCLE ( 'NONE', #10471, 1.500000000000001332 ) ;
#4047=CARTESIAN_POINT ( 'NONE',  ( 19.13369214859999801, 50.50000000000000000, -142.8052959529999839 ) ) ;
#4053=CARTESIAN_POINT ( 'NONE',  ( -31.50000000000000000, -36.00000000000000000, -137.0552959530000123 ) ) ;
#4061=CARTESIAN_POINT ( 'NONE',  ( -7.500000000000000000, 42.50000000000000000, -150.0552959529999839 ) ) ;
#4063=ORIENTED_EDGE ( 'NONE', *, *, #16184, .T. ) ;
#4065=FACE_OUTER_BOUND ( 'NONE', #6237, .T. ) ;
#4067=CYLINDRICAL_SURFACE ( 'NONE', #1600, 7.500000000000005329 ) ;
#4082=ORIENTED_EDGE ( 'NONE', *, *, #20435, .T. ) ;
#4086=CARTESIAN_POINT ( 'NONE',  ( -2.500000000000000000, 40.00000000000000000, -151.0552959529999839 ) ) ;
#4088=CARTESIAN_POINT ( 'NONE',  ( 13.13369214859999978, 51.50000000000000000, -137.0552959530000123 ) ) ;
#4090=EDGE_CURVE ( 'NONE', #13352, #13032, #9939, .T. ) ;
#4103=VECTOR ( 'NONE', #102, 1000.000000000000000 ) ;
#4116=CARTESIAN_POINT ( 'NONE',  ( 8.750000000000001776, -47.26504245777761071, -150.0552959530000123 ) ) ;
#4117=ORIENTED_EDGE ( 'NONE', *, *, #984, .F. ) ;
#4126=ORIENTED_EDGE ( 'NONE', *, *, #2070, .T. ) ;
#4127=DIRECTION ( 'NONE',  ( 1.000000000000000000, 0.000000000000000000, 0.000000000000000000 ) ) ;
#4129=LINE ( 'NONE', #20437, #11090 ) ;
#4130=LINE ( 'NONE', #7693, #12856 ) ;
#4132=VECTOR ( 'NONE', #7924, 1000.000000000000000 ) ;
#4135=VERTEX_POINT ( 'NONE', #23397 ) ;
#4140=ADVANCED_FACE ( 'NONE', ( #1755 ), #8744, .F. ) ;
#4141=PLANE ( 'NONE',  #19347 ) ;
#4151=LINE ( 'NONE', #14870, #10079 ) ;
#4153=ORIENTED_EDGE ( 'NONE', *, *, #12358, .F. ) ;
#4158=EDGE_CURVE ( 'NONE', #21164, #3905, #23516, .T. ) ;
#4159=VECTOR ( 'NONE', #13233, 1000.000000000000000 ) ;
#4163=VECTOR ( 'NONE', #17355, 1000.000000000000227 ) ;
#4164=LINE ( 'NONE', #4047, #20930 ) ;
#4168=DIRECTION ( 'NONE',  ( -1.000000000000000000, 0.000000000000000000, 0.000000000000000000 ) ) ;
#4174=CARTESIAN_POINT ( 'NONE',  ( -32.50000000000000000, 10.25000000000000000, -137.0552959530000123 ) ) ;
#4182=DIRECTION ( 'NONE',  ( 0.000000000000000000, 0.000000000000000000, 1.000000000000000000 ) ) ;
#4186=DIRECTION ( 'NONE',  ( 0.000000000000000000, 1.000000000000000000, 0.000000000000000000 ) ) ;
#4190=DIRECTION ( 'NONE',  ( 0.000000000000000000, -1.000000000000000000, 0.000000000000000000 ) ) ;
#4201=EDGE_CURVE ( 'NONE', #18280, #4867, #15996, .T. ) ;
#4204=EDGE_CURVE ( 'NONE', #19876, #3906, #1581, .T. ) ;
#4206=LINE ( 'NONE', #2433, #17133 ) ;
#4209=ORIENTED_EDGE ( 'NONE', *, *, #18818, .T. ) ;
#4211=CARTESIAN_POINT ( 'NONE',  ( 12.49993271304849252, 36.89748944252419705, -150.0552959529999839 ) ) ;
#4228=CARTESIAN_POINT ( 'NONE',  ( 18.95053822279999878, -51.50000000000000000, -149.8052959529999839 ) ) ;
#4236=CARTESIAN_POINT ( 'NONE',  ( -31.00000000000000000, -7.105427357599999217E-15, -149.5552959529999839 ) ) ;
#4243=ORIENTED_EDGE ( 'NONE', *, *, #17001, .F. ) ;
#4244=( NAMED_UNIT ( * ) PLANE_ANGLE_UNIT ( ) SI_UNIT ( $, .RADIAN. ) );
#4245=ORIENTED_EDGE ( 'NONE', *, *, #1560, .T. ) ;
#4248=DIRECTION ( 'NONE',  ( 0.000000000000000000, 2.256988247090000272E-12, 1.000000000000000000 ) ) ;
#4253=CARTESIAN_POINT ( 'NONE',  ( 11.45511797032570911, 26.15112731433314153, -150.0552959529999839 ) ) ;
#4257=CARTESIAN_POINT ( 'NONE',  ( 19.27350934360000068, 50.38169314270000143, -149.5552959529999839 ) ) ;
#4262=AXIS2_PLACEMENT_3D ( 'NONE', #22394, #11194, #22162 ) ;
#4271=EDGE_LOOP ( 'NONE', ( #12112, #13477, #16670, #13883 ) ) ;
#4273=PLANE ( 'NONE',  #14283 ) ;
#4275=ORIENTED_EDGE ( 'NONE', *, *, #9679, .F. ) ;
#4285=CARTESIAN_POINT ( 'NONE',  ( 19.13369214859999801, 51.50000000000000000, -136.0552959530000123 ) ) ;
#4287=DIRECTION ( 'NONE',  ( 0.000000000000000000, -1.000000000000000000, 0.000000000000000000 ) ) ;
#4291=ORIENTED_EDGE ( 'NONE', *, *, #17001, .T. ) ;
#4314=DIRECTION ( 'NONE',  ( 0.000000000000000000, 0.000000000000000000, 1.000000000000000000 ) ) ;
#4316=DIRECTION ( 'NONE',  ( 0.000000000000000000, 1.000000000000000000, 0.000000000000000000 ) ) ;
#4320=ORIENTED_EDGE ( 'NONE', *, *, #8018, .T. ) ;
#4321=CARTESIAN_POINT ( 'NONE',  ( 0.000000000000000000, -50.00000000000000000, -150.0552959529999839 ) ) ;
#4323=PLANE ( 'NONE',  #9074 ) ;
#4328=CARTESIAN_POINT ( 'NONE',  ( 32.50000000000000000, 0.000000000000000000, -136.0552959530000123 ) ) ;
#4330=CARTESIAN_POINT ( 'NONE',  ( 9.763108217333922312, -36.11272049728156475, -150.0552959529999839 ) ) ;
#4332=VERTEX_POINT ( 'NONE', #18940 ) ;
#4339=ORIENTED_EDGE ( 'NONE', *, *, #2443, .T. ) ;
#4346=CARTESIAN_POINT ( 'NONE',  ( 0.000000000000000000, 42.50000000000000000, -150.0552959529999839 ) ) ;
#4348=CARTESIAN_POINT ( 'NONE',  ( -32.50000000000000000, 1.000000000000000000, -143.3052959529999839 ) ) ;
#4350=VERTEX_POINT ( 'NONE', #19063 ) ;
#4352=CARTESIAN_POINT ( 'NONE',  ( 1.133692148550000001, -50.50000000000000000, -136.0552959530000123 ) ) ;
#4355=VERTEX_POINT ( 'NONE', #20063 ) ;
#4359=CARTESIAN_POINT ( 'NONE',  ( -25.86630785139999844, -50.50000000000000000, -136.0552959530000123 ) ) ;
#4360=VERTEX_POINT ( 'NONE', #2774 ) ;
#4364=DIRECTION ( 'NONE',  ( 1.000000000000000000, 0.000000000000000000, -2.257453483404482811E-12 ) ) ;
#4365=DIRECTION ( 'NONE',  ( -1.000000000000000000, 0.000000000000000000, 0.000000000000000000 ) ) ;
#4369=CARTESIAN_POINT ( 'NONE',  ( -1.753667363961266989, 45.51009696919363989, -150.0552959529999839 ) ) ;
#4370=CARTESIAN_POINT ( 'NONE',  ( 32.50000000000000000, -21.03620104879999886, -137.0552959530000123 ) ) ;
#4379=EDGE_CURVE ( 'NONE', #5378, #22981, #14383, .T. ) ;
#4381=ORIENTED_EDGE ( 'NONE', *, *, #23081, .F. ) ;
#4383=CARTESIAN_POINT ( 'NONE',  ( 20.57808196999505412, -21.28524365307785260, -150.0552959530000123 ) ) ;
#4389=FACE_OUTER_BOUND ( 'NONE', #5302, .T. ) ;
#4390=ORIENTED_EDGE ( 'NONE', *, *, #229, .F. ) ;
#4396=DIRECTION ( 'NONE',  ( -1.000000000000000000, 0.000000000000000000, -2.245315044929999938E-12 ) ) ;
#4399=EDGE_LOOP ( 'NONE', ( #7208, #944, #20037, #2985 ) ) ;
#4401=VERTEX_POINT ( 'NONE', #18390 ) ;
#4402=CARTESIAN_POINT ( 'NONE',  ( 1.878640834937223669, -1.989143058887305804, -150.0552959529999839 ) ) ;
#4405=DIRECTION ( 'NONE',  ( -1.000000000000000000, 0.000000000000000000, -2.245315044999999693E-12 ) ) ;
#4407=EDGE_LOOP ( 'NONE', ( #20782, #9100, #14886, #3390, #16281, #17318, #18636, #5271, #5469, #18972, #1344, #8117, #5906, #21456, #13109, #11576 ) ) ;
#4409=ADVANCED_FACE ( 'NONE', ( #9321 ), #18498, .F. ) ;
#4412=CARTESIAN_POINT ( 'NONE',  ( -1.500000000000000000, 44.50000000000000000, -151.0552959529999839 ) ) ;
#4418=FACE_OUTER_BOUND ( 'NONE', #8584, .T. ) ;
#4425=AXIS2_PLACEMENT_3D ( 'NONE', #23411, #7106, #14367 ) ;
#4438=CARTESIAN_POINT ( 'NONE',  ( 6.007375567780162129, 13.00000000000000000, -150.0552959530000123 ) ) ;
#4444=ORIENTED_EDGE ( 'NONE', *, *, #18967, .T. ) ;
#4453=DIRECTION ( 'NONE',  ( 0.000000000000000000, 1.000000000000000000, -2.273736754430000208E-12 ) ) ;
#4468=AXIS2_PLACEMENT_3D ( 'NONE', #21549, #15827, #14280 ) ;
#4471=CYLINDRICAL_SURFACE ( 'NONE', #12110, 2.999999999999999112 ) ;
#4472=ORIENTED_EDGE ( 'NONE', *, *, #22118, .T. ) ;
#4476=DIRECTION ( 'NONE',  ( 0.000000000000000000, 0.000000000000000000, 1.000000000000000000 ) ) ;
#4477=CARTESIAN_POINT ( 'NONE',  ( 19.00000000000000000, 33.50000000000000000, -151.0552959529999839 ) ) ;
#4485=B_SPLINE_CURVE_WITH_KNOTS ( 'NONE', 3,
 ( #7311, #16696, #289, #5634, #18604, #7529, #22067, #18482, #5755, #4211, #16820, #7764, #13011, #20393, #9070, #16359, #14574, #21840 ),
 .UNSPECIFIED., .F., .F.,
 ( 4, 2, 2, 2, 2, 2, 2, 2, 4 ),
 ( 0.000000000000000000, 0.1250000000000000000, 0.2500000000000000000, 0.3750000000000000000, 0.5000000000000000000, 0.6250000000000000000, 0.7500000000000000000, 0.8750000000000000000, 1.000000000000000000 ),
 .UNSPECIFIED. ) ;
#4486=DIRECTION ( 'NONE',  ( 0.000000000000000000, 1.000000000000000000, -2.245315044999999693E-12 ) ) ;
#4488=VECTOR ( 'NONE', #19047, 1000.000000000000000 ) ;
#4491=CARTESIAN_POINT ( 'NONE',  ( 22.50000000000000000, 33.50000000000000000, -150.0552959529999839 ) ) ;
#4497=ORIENTED_EDGE ( 'NONE', *, *, #7862, .T. ) ;
#4499=PLANE ( 'NONE',  #9185 ) ;
#4507=EDGE_LOOP ( 'NONE', ( #8172, #16810, #17638, #11067 ) ) ;
#4508=CARTESIAN_POINT ( 'NONE',  ( -31.00000000000000000, -50.00000000000000000, -149.5552959529999839 ) ) ;
#4513=VECTOR ( 'NONE', #14501, 1000.000000000000227 ) ;
#4514=ORIENTED_EDGE ( 'NONE', *, *, #11559, .T. ) ;
#4518=CYLINDRICAL_SURFACE ( 'NONE', #23148, 3.000000000000000000 ) ;
#4519=ADVANCED_FACE ( 'NONE', ( #8339 ), #14181, .T. ) ;
#4521=VERTEX_POINT ( 'NONE', #21446 ) ;
#4523=VECTOR ( 'NONE', #16175, 1000.000000000000000 ) ;
#4530=DIRECTION ( 'NONE',  ( -1.000000000000000000, 0.000000000000000000, 0.000000000000000000 ) ) ;
#4532=CARTESIAN_POINT ( 'NONE',  ( -13.86630785140000022, 51.50000000000000000, -136.5552959530000123 ) ) ;
#4541=VECTOR ( 'NONE', #2541, 1000.000000000000000 ) ;
#4547=EDGE_CURVE ( 'NONE', #23292, #16505, #16938, .T. ) ;
#4548=ORIENTED_EDGE ( 'NONE', *, *, #1983, .T. ) ;
#4551=VECTOR ( 'NONE', #21648, 1000.000000000000000 ) ;
#4554=DIRECTION ( 'NONE',  ( 0.000000000000000000, 0.000000000000000000, 1.000000000000000000 ) ) ;
#4563=CARTESIAN_POINT ( 'NONE',  ( 3.839256067998265465, -35.21302158184240483, -150.0552959529999839 ) ) ;
#4567=EDGE_CURVE ( 'NONE', #11744, #3203, #9275, .T. ) ;
#4569=ORIENTED_EDGE ( 'NONE', *, *, #18194, .F. ) ;
#4570=LINE ( 'NONE', #16833, #3878 ) ;
#4571=CARTESIAN_POINT ( 'NONE',  ( -32.50000000000000000, 50.50000000000000000, -142.8052959529999839 ) ) ;
#4573=ORIENTED_EDGE ( 'NONE', *, *, #11887, .F. ) ;
#4577=CARTESIAN_POINT ( 'NONE',  ( -3.500000000000000000, 34.00000000000000000, -151.0552959529999839 ) ) ;
#4579=VECTOR ( 'NONE', #7722, 1000.000000000000000 ) ;
#4582=DIRECTION ( 'NONE',  ( 0.000000000000000000, 0.000000000000000000, 1.000000000000000000 ) ) ;
#4586=ADVANCED_FACE ( 'NONE', ( #12496 ), #2053, .F. ) ;
#4590=CARTESIAN_POINT ( 'NONE',  ( 0.000000000000000000, 0.000000000000000000, 0.000000000000000000 ) ) ;
#4592=VERTEX_POINT ( 'NONE', #3704 ) ;
#4599=VECTOR ( 'NONE', #3774, 1000.000000000000000 ) ;
#4608=CARTESIAN_POINT ( 'NONE',  ( 0.8371776177479999248, 12.00000000000000000, -144.0552959529999839 ) ) ;
#4613=CARTESIAN_POINT ( 'NONE',  ( 22.89800326577686462, 33.50000000000000000, -150.0552959529999839 ) ) ;
#4616=VECTOR ( 'NONE', #20028, 1000.000000000000227 ) ;
#4634=ORIENTED_EDGE ( 'NONE', *, *, #6385, .T. ) ;
#4639=FACE_OUTER_BOUND ( 'NONE', #17567, .T. ) ;
#4643=CARTESIAN_POINT ( 'NONE',  ( -31.50000000000000000, 1.000000000000000000, -143.3052959529999839 ) ) ;
#4644=EDGE_LOOP ( 'NONE', ( #23206, #11135, #22818, #8606, #7592, #15919, #14416, #23110, #294, #23197, #3430, #23172, #13316, #2699, #20994, #21859 ) ) ;
#4645=VERTEX_POINT ( 'NONE', #1815 ) ;
#4652=LINE ( 'NONE', #23090, #5895 ) ;
#4654=CARTESIAN_POINT ( 'NONE',  ( 23.10730091830127719, -17.50000000000000000, -150.0552959529999839 ) ) ;
#4656=DIRECTION ( 'NONE',  ( -1.457881434619999915E-12, 1.723066134219999902E-12, 1.000000000000000000 ) ) ;
#4658=CARTESIAN_POINT ( 'NONE',  ( -2.500000000000000000, 0.000000000000000000, -150.0552959529999839 ) ) ;
#4659=EDGE_CURVE ( 'NONE', #6470, #20530, #7275, .T. ) ;
#4668=CARTESIAN_POINT ( 'NONE',  ( -31.00000000000000000, 19.50000000000000000, -149.5552959529999839 ) ) ;
#4671=ORIENTED_EDGE ( 'NONE', *, *, #14903, .F. ) ;
#4675=DIRECTION ( 'NONE',  ( 1.000000000000000000, 0.000000000000000000, 0.000000000000000000 ) ) ;
#4684=ADVANCED_FACE ( 'NONE', ( #22374 ), #15111, .F. ) ;
#4693=ORIENTED_EDGE ( 'NONE', *, *, #20534, .T. ) ;
#4699=CARTESIAN_POINT ( 'NONE',  ( 3.611212474210000402E-11, 0.000000000000000000, -135.0552959530000123 ) ) ;
#4702=LINE ( 'NONE', #10622, #15791 ) ;
#4710=EDGE_LOOP ( 'NONE', ( #19752, #17367, #20755, #19476 ) ) ;
#4713=LINE ( 'NONE', #4831, #340 ) ;
#4721=FACE_OUTER_BOUND ( 'NONE', #16269, .T. ) ;
#4732=EDGE_CURVE ( 'NONE', #4332, #751, #22497, .T. ) ;
#4735=VERTEX_POINT ( 'NONE', #22144 ) ;
#4739=CARTESIAN_POINT ( 'NONE',  ( -6.683153925719999222, -51.50000000000000000, -136.0552959530000123 ) ) ;
#4749=LINE ( 'NONE', #2851, #17077 ) ;
#4767=B_SPLINE_CURVE_WITH_KNOTS ( 'NONE', 3,
 ( #6431, #972, #15124, #8324, #20717, #13449, #2870, #9634, #19281, #17377, #16907, #15600, #8205, #15250, #6312, #13817, #6087, #2640 ),
 .UNSPECIFIED., .F., .F.,
 ( 4, 2, 2, 2, 2, 2, 2, 2, 4 ),
 ( 0.000000000000000000, 0.1249999999999998335, 0.2499999999999996669, 0.3749999999999995004, 0.4999999999999993339, 0.6250000000000002220, 0.7500000000000002220, 0.8750000000000001110, 1.000000000000000000 ),
 .UNSPECIFIED. ) ;
#4768=CARTESIAN_POINT ( 'NONE',  ( 20.87864083493722234, -18.98914305888730425, -150.0552959529999839 ) ) ;
#4771=CARTESIAN_POINT ( 'NONE',  ( 8.750000000000000000, -47.00000000000000000, -150.0552959529999839 ) ) ;
#4775=CARTESIAN_POINT ( 'NONE',  ( -31.00000000000000000, -51.50000000000000000, -149.5552959529999839 ) ) ;
#4777=LINE ( 'NONE', #17271, #2745 ) ;
#4778=LINE ( 'NONE', #20725, #9925 ) ;
#4782=CARTESIAN_POINT ( 'NONE',  ( -6.683153925719999222, 50.50000000000000000, -149.5552959529999839 ) ) ;
#4785=PRODUCT ( 'Main Base', 'Main Base', '', ( #23379 ) ) ;
#4799=CARTESIAN_POINT ( 'NONE',  ( 9.479581287884620622, -37.28079462196955518, -150.0552959529999839 ) ) ;
#4800=DIRECTION ( 'NONE',  ( -1.000000000000000000, 0.000000000000000000, 2.245315044999999693E-12 ) ) ;
#4802=SURFACE_STYLE_FILL_AREA ( #19445 ) ;
#4805=VECTOR ( 'NONE', #21719, 1000.000000000000000 ) ;
#4815=EDGE_CURVE ( 'NONE', #21392, #5806, #2226, .T. ) ;
#4817=CARTESIAN_POINT ( 'NONE',  ( -13.48914305888730425, -40.37864083493721523, -150.0552959529999839 ) ) ;
#4823=LINE ( 'NONE', #19336, #2921 ) ;
#4831=CARTESIAN_POINT ( 'NONE',  ( -32.50000000000000000, -50.50000000000000000, -143.0552959529999839 ) ) ;
#4836=DIRECTION ( 'NONE',  ( 0.000000000000000000, 0.000000000000000000, -1.000000000000000000 ) ) ;
#4839=CARTESIAN_POINT ( 'NONE',  ( -10.00000000000000000, 25.50000000000000000, -151.0552959529999839 ) ) ;
#4844=EDGE_CURVE ( 'NONE', #13274, #18962, #6766, .T. ) ;
#4848=AXIS2_PLACEMENT_3D ( 'NONE', #828, #7314, #14335 ) ;
#4857=CARTESIAN_POINT ( 'NONE',  ( 6.000000000000000000, -3.500000000000000000, -150.0552959529999839 ) ) ;
#4867=VERTEX_POINT ( 'NONE', #12118 ) ;
#4871=DIRECTION ( 'NONE',  ( 0.000000000000000000, 1.000000000000000000, 0.000000000000000000 ) ) ;
#4878=CARTESIAN_POINT ( 'NONE',  ( -31.00000000000000000, 0.000000000000000000, -151.0552959529999839 ) ) ;
#4882=ADVANCED_FACE ( 'NONE', ( #20823 ), #4518, .T. ) ;
#4885=LINE ( 'NONE', #17621, #301 ) ;
#4886=LINE ( 'NONE', #867, #16775 ) ;
#4892=AXIS2_PLACEMENT_3D ( 'NONE', #9352, #7810, #20219 ) ;
#4894=EDGE_CURVE ( 'NONE', #5505, #18280, #2856, .T. ) ;
#4897=CARTESIAN_POINT ( 'NONE',  ( -12.50000000000000000, 19.50000000000000000, -150.0552959529999839 ) ) ;
#4900=DIRECTION ( 'NONE',  ( 1.000000000000000000, 0.000000000000000000, 0.000000000000000000 ) ) ;
#4901=CARTESIAN_POINT ( 'NONE',  ( 4.698575659221273071, -2.000067229902509514, -150.0552959529999839 ) ) ;
#4902=ORIENTED_EDGE ( 'NONE', *, *, #20300, .T. ) ;
#4903=VECTOR ( 'NONE', #5788, 1000.000000000000000 ) ;
#4908=AXIS2_PLACEMENT_3D ( 'NONE', #10933, #16313, #3464 ) ;
#4911=VECTOR ( 'NONE', #17103, 1000.000000000000000 ) ;
#4913=CYLINDRICAL_SURFACE ( 'NONE', #3768, 3.000000000000002665 ) ;
#4918=DIRECTION ( 'NONE',  ( 1.000000000000000000, 0.000000000000000000, 0.000000000000000000 ) ) ;
#4922=EDGE_CURVE ( 'NONE', #9664, #1217, #6414, .T. ) ;
#4923=VECTOR ( 'NONE', #1793, 1000.000000000000000 ) ;
#4927=CARTESIAN_POINT ( 'NONE',  ( -32.50000000000000000, -50.50000000000000000, -149.5552959529999839 ) ) ;
#4929=CIRCLE ( 'NONE', #378, 1.499999999999999556 ) ;
#4937=FACE_OUTER_BOUND ( 'NONE', #9115, .T. ) ;
#4941=CARTESIAN_POINT ( 'NONE',  ( 18.95053822279999878, -50.00000000000000000, -149.5552959529999839 ) ) ;
#4946=AXIS2_PLACEMENT_3D ( 'NONE', #6533, #13802, #3560 ) ;
#4954=FACE_OUTER_BOUND ( 'NONE', #1545, .T. ) ;
#4958=ORIENTED_EDGE ( 'NONE', *, *, #19703, .F. ) ;
#4959=CARTESIAN_POINT ( 'NONE',  ( -15.00000000000000000, -43.00000000000000000, -145.5552959529999839 ) ) ;
#4966=VERTEX_POINT ( 'NONE', #10557 ) ;
#4972=ORIENTED_EDGE ( 'NONE', *, *, #9302, .T. ) ;
#4975=ORIENTED_EDGE ( 'NONE', *, *, #3419, .T. ) ;
#4977=FACE_OUTER_BOUND ( 'NONE', #21229, .T. ) ;
#4983=VERTEX_POINT ( 'NONE', #5573 ) ;
#4988=ORIENTED_EDGE ( 'NONE', *, *, #21807, .T. ) ;
#4992=EDGE_CURVE ( 'NONE', #23292, #3037, #19868, .T. ) ;
#4993=CARTESIAN_POINT ( 'NONE',  ( 4.500000000000000000, -3.500000000000000000, -145.5552959529999839 ) ) ;
#4994=VECTOR ( 'NONE', #4800, 1000.000000000000000 ) ;
#4995=CIRCLE ( 'NONE', #8012, 0.5000000000000009992 ) ;
#4997=DIRECTION ( 'NONE',  ( 0.000000000000000000, -2.956752937091289955E-12, -1.000000000000000000 ) ) ;
#5002=ORIENTED_EDGE ( 'NONE', *, *, #14270, .F. ) ;
#5005=CARTESIAN_POINT ( 'NONE',  ( 26.50000000000000000, -20.10730091830127009, -150.0552959530000123 ) ) ;
#5006=DIRECTION ( 'NONE',  ( 1.000000000000000000, 0.000000000000000000, 0.000000000000000000 ) ) ;
#5007=LINE ( 'NONE', #14528, #21361 ) ;
#5012=AXIS2_PLACEMENT_3D ( 'NONE', #5622, #8214, #17388 ) ;
#5015=DIRECTION ( 'NONE',  ( 1.000000000000000000, 0.000000000000000000, 0.000000000000000000 ) ) ;
#5019=ORIENTED_EDGE ( 'NONE', *, *, #13843, .T. ) ;
#5020=FACE_OUTER_BOUND ( 'NONE', #4644, .T. ) ;
#5024=CARTESIAN_POINT ( 'NONE',  ( -32.50000000000000000, 14.00000000000000000, -144.0552959529999839 ) ) ;
#5025=AXIS2_PLACEMENT_3D ( 'NONE', #4590, #17084, #1161 ) ;
#5026=CYLINDRICAL_SURFACE ( 'NONE', #22767, 1.500000000000001332 ) ;
#5030=EDGE_CURVE ( 'NONE', #7233, #3293, #12708, .T. ) ;
#5037=CARTESIAN_POINT ( 'NONE',  ( -0.6175362654710214727, 22.91577772018773729, -150.0552959529999839 ) ) ;
#5038=EDGE_CURVE ( 'NONE', #6002, #22754, #8383, .T. ) ;
#5041=EDGE_CURVE ( 'NONE', #21465, #8058, #461, .T. ) ;
#5043=PRESENTATION_STYLE_ASSIGNMENT (( #12283 ) ) ;
#5048=CARTESIAN_POINT ( 'NONE',  ( 25.50000000000000000, 22.50000000000000000, -150.0552959529999839 ) ) ;
#5050=VERTEX_POINT ( 'NONE', #11606 ) ;
#5057=CARTESIAN_POINT ( 'NONE',  ( -17.39900052719454138, -41.15635984007523973, -150.0552959530000123 ) ) ;
#5073=CARTESIAN_POINT ( 'NONE',  ( -5.985028652404004390, 19.88109793996616403, -150.0552959529999839 ) ) ;
#5085=ORIENTED_EDGE ( 'NONE', *, *, #21376, .T. ) ;
#5088=EDGE_LOOP ( 'NONE', ( #7, #16480, #19975, #17867 ) ) ;
#5095=ORIENTED_EDGE ( 'NONE', *, *, #9122, .F. ) ;
#5098=CARTESIAN_POINT ( 'NONE',  ( 0.000000000000000000, 0.000000000000000000, -140.0552959529999839 ) ) ;
#5104=ADVANCED_FACE ( 'NONE', ( #18771 ), #12942, .F. ) ;
#5109=CARTESIAN_POINT ( 'NONE',  ( -0.7500000000009999779, -50.00000000000000000, -149.5552959529999839 ) ) ;
#5112=ORIENTED_EDGE ( 'NONE', *, *, #2755, .F. ) ;
#5120=CARTESIAN_POINT ( 'NONE',  ( 32.00000000000000000, -33.03620104880000241, -137.0552959530000123 ) ) ;
#5125=CARTESIAN_POINT ( 'NONE',  ( -6.774730888589999722, 50.00000000000000000, -151.0552959529999839 ) ) ;
#5127=LINE ( 'NONE', #4782, #6943 ) ;
#5128=CARTESIAN_POINT ( 'NONE',  ( 5.809692093864619267, -2.742832019563268720, -150.0552959530000123 ) ) ;
#5129=ORIENTED_EDGE ( 'NONE', *, *, #14500, .T. ) ;
#5136=VECTOR ( 'NONE', #2668, 1000.000000000000000 ) ;
#5137=ORIENTED_EDGE ( 'NONE', *, *, #9808, .F. ) ;
#5140=CARTESIAN_POINT ( 'NONE',  ( 13.13369214859999978, 51.00000000000000000, -137.0552959530000123 ) ) ;
#5141=DIRECTION ( 'NONE',  ( -1.000000000000000000, 0.000000000000000000, 0.000000000000000000 ) ) ;
#5143=ORIENTED_EDGE ( 'NONE', *, *, #3389, .T. ) ;
#5144=DIRECTION ( 'NONE',  ( 0.000000000000000000, 1.000000000000000000, 0.000000000000000000 ) ) ;
#5158=EDGE_CURVE ( 'NONE', #954, #10456, #9823, .T. ) ;
#5160=CARTESIAN_POINT ( 'NONE',  ( -12.00000000000000000, -42.60730091830127719, -150.0552959530000123 ) ) ;
#5162=CARTESIAN_POINT ( 'NONE',  ( 19.45666326950000169, 50.88169314249999786, -150.0552959529999839 ) ) ;
#5166=CARTESIAN_POINT ( 'NONE',  ( 32.05742780150000470, 40.87448416799999507, -149.5552959529999839 ) ) ;
#5178=DIRECTION ( 'NONE',  ( 0.000000000000000000, 0.000000000000000000, 1.000000000000000000 ) ) ;
#5180=ORIENTED_EDGE ( 'NONE', *, *, #6691, .F. ) ;
#5183=EDGE_CURVE ( 'NONE', #12670, #11634, #14857, .T. ) ;
#5187=LINE ( 'NONE', #5545, #21691 ) ;
#5188=EDGE_CURVE ( 'NONE', #21084, #4592, #1879, .T. ) ;
#5191=VECTOR ( 'NONE', #5198, 1000.000000000000000 ) ;
#5198=DIRECTION ( 'NONE',  ( 0.000000000000000000, -2.256683728769999802E-12, 1.000000000000000000 ) ) ;
#5208=ORIENTED_EDGE ( 'NONE', *, *, #11081, .T. ) ;
#5218=CARTESIAN_POINT ( 'NONE',  ( -2.273230205684010574, 46.10147512692400085, -150.0552959530000123 ) ) ;
#5237=EDGE_CURVE ( 'NONE', #9123, #11298, #21272, .T. ) ;
#5238=CARTESIAN_POINT ( 'NONE',  ( 6.343640159924754940, -5.899000527194532495, -150.0552959529999839 ) ) ;
#5240=CARTESIAN_POINT ( 'NONE',  ( -3.500000000000000000, 44.50000000000000000, -151.0552959529999839 ) ) ;
#5250=EDGE_LOOP ( 'NONE', ( #22987, #11568 ) ) ;
#5251=DIRECTION ( 'NONE',  ( 1.000000000000000000, 0.000000000000000000, 0.000000000000000000 ) ) ;
#5252=AXIS2_PLACEMENT_3D ( 'NONE', #8436, #3209, #10441 ) ;
#5254=VECTOR ( 'NONE', #11829, 1000.000000000000000 ) ;
#5259=CARTESIAN_POINT ( 'NONE',  ( -0.9519686233540903819, 21.48063989304597499, -150.0552959530000123 ) ) ;
#5262=ORIENTED_EDGE ( 'NONE', *, *, #14126, .T. ) ;
#5263=LINE ( 'NONE', #14665, #3099 ) ;
#5270=AXIS2_PLACEMENT_3D ( 'NONE', #6511, #15429, #19233 ) ;
#5271=ORIENTED_EDGE ( 'NONE', *, *, #150, .F. ) ;
#5277=VECTOR ( 'NONE', #9617, 1000.000000000000000 ) ;
#5278=VECTOR ( 'NONE', #16659, 1000.000000000000000 ) ;
#5280=CARTESIAN_POINT ( 'NONE',  ( 20.50000000000000000, 25.50000000000000000, -150.0552959529999839 ) ) ;
#5281=CARTESIAN_POINT ( 'NONE',  ( -13.53810979399600001, -43.39038688405765498, -150.0552959530000123 ) ) ;
#5283=CARTESIAN_POINT ( 'NONE',  ( 19.13369214859999801, -50.50000000000000000, -143.0552959529999839 ) ) ;
#5286=CARTESIAN_POINT ( 'NONE',  ( 19.13369214859999801, 51.00000000000000000, -136.0552959530000123 ) ) ;
#5289=ADVANCED_FACE ( 'NONE', ( #19008 ), #22819, .F. ) ;
#5292=VERTEX_POINT ( 'NONE', #12211 ) ;
#5295=CIRCLE ( 'NONE', #21655, 2.000000000000000000 ) ;
#5302=EDGE_LOOP ( 'NONE', ( #15112, #22922, #17589, #6132 ) ) ;
#5303=PLANE ( 'NONE',  #11503 ) ;
#5311=EDGE_CURVE ( 'NONE', #13247, #17813, #19487, .T. ) ;
#5314=CIRCLE ( 'NONE', #8341, 1.500000000000001332 ) ;
#5321=ORIENTED_EDGE ( 'NONE', *, *, #19563, .F. ) ;
#5325=ORIENTED_EDGE ( 'NONE', *, *, #4922, .T. ) ;
#5328=EDGE_CURVE ( 'NONE', #4355, #3527, #13520, .T. ) ;
#5339=ORIENTED_EDGE ( 'NONE', *, *, #23349, .T. ) ;
#5340=AXIS2_PLACEMENT_3D ( 'NONE', #23153, #16134, #3394 ) ;
#5342=DIRECTION ( 'NONE',  ( 0.000000000000000000, 1.000000000000000000, 0.000000000000000000 ) ) ;
#5358=DIRECTION ( 'NONE',  ( 1.000000000000000000, 0.000000000000000000, 0.000000000000000000 ) ) ;
#5359=DIRECTION ( 'NONE',  ( -1.000000000000000000, 0.000000000000000000, 0.000000000000000000 ) ) ;
#5360=DIRECTION ( 'NONE',  ( 0.7633862853691523176, -0.6459422414661291079, 0.000000000000000000 ) ) ;
#5362=DIRECTION ( 'NONE',  ( -1.456612608300000016E-12, 1.733724275239999964E-12, 1.000000000000000000 ) ) ;
#5367=CARTESIAN_POINT ( 'NONE',  ( 1.500000000000000000, -3.892699081698731245, -150.0552959530000123 ) ) ;
#5378=VERTEX_POINT ( 'NONE', #196 ) ;
#5382=DIRECTION ( 'NONE',  ( -0.7071067811870332953, 0.000000000000000000, 0.7071067811860618502 ) ) ;
#5388=VECTOR ( 'NONE', #21145, 1000.000000000000000 ) ;
#5394=ORIENTED_EDGE ( 'NONE', *, *, #13587, .T. ) ;
#5397=PLANE ( 'NONE',  #2455 ) ;
#5399=ORIENTED_EDGE ( 'NONE', *, *, #784, .F. ) ;
#5402=MECHANICAL_DESIGN_GEOMETRIC_PRESENTATION_REPRESENTATION('',(#21752),#21377);
#5414=PLANE ( 'NONE',  #14313 ) ;
#5422=ORIENTED_EDGE ( 'NONE', *, *, #10406, .F. ) ;
#5429=LINE ( 'NONE', #8741, #6821 ) ;
#5430=CARTESIAN_POINT ( 'NONE',  ( -15.50000000000000000, 47.50000000000000000, -150.5552959529999839 ) ) ;
#5432=DIRECTION ( 'NONE',  ( 0.6459422414661299960, 0.7633862853691516515, 0.000000000000000000 ) ) ;
#5435=ADVANCED_FACE ( 'NONE', ( #6949 ), #1846, .F. ) ;
#5436=ORIENTED_EDGE ( 'NONE', *, *, #17963, .F. ) ;
#5439=DIRECTION ( 'NONE',  ( -2.257252162960000001E-12, 0.000000000000000000, -1.000000000000000000 ) ) ;
#5466=EDGE_CURVE ( 'NONE', #14773, #2149, #17560, .T. ) ;
#5469=ORIENTED_EDGE ( 'NONE', *, *, #8630, .F. ) ;
#5475=DIRECTION ( 'NONE',  ( 0.000000000000000000, -1.000000000000000000, 0.000000000000000000 ) ) ;
#5484=CARTESIAN_POINT ( 'NONE',  ( 1.500000000000000000, -3.500000000000000000, -150.0552959529999839 ) ) ;
#5500=ORIENTED_EDGE ( 'NONE', *, *, #6889, .F. ) ;
#5505=VERTEX_POINT ( 'NONE', #16573 ) ;
#5506=LINE ( 'NONE', #12754, #4616 ) ;
#5511=ORIENTED_EDGE ( 'NONE', *, *, #22750, .F. ) ;
#5512=ADVANCED_FACE ( 'NONE', ( #9297 ), #20163, .F. ) ;
#5515=ORIENTED_EDGE ( 'NONE', *, *, #9632, .F. ) ;
#5526=DIRECTION ( 'NONE',  ( -0.7633862853691524286, -0.6459422414661293299, 0.000000000000000000 ) ) ;
#5529=EDGE_LOOP ( 'NONE', ( #8370, #9237, #14934, #2807 ) ) ;
#5532=VECTOR ( 'NONE', #8091, 1000.000000000000000 ) ;
#5534=CARTESIAN_POINT ( 'NONE',  ( 32.50000000000000000, -39.80430157320000006, -149.5552959529999839 ) ) ;
#5535=ORIENTED_EDGE ( 'NONE', *, *, #6029, .T. ) ;
#5536=VECTOR ( 'NONE', #17425, 1000.000000000000000 ) ;
#5542=ADVANCED_FACE ( 'NONE', ( #12883 ), #20039, .F. ) ;
#5545=CARTESIAN_POINT ( 'NONE',  ( 32.00000000000000000, -21.03620104879999886, -136.0552959530000123 ) ) ;
#5549=AXIS2_PLACEMENT_3D ( 'NONE', #6051, #15332, #18783 ) ;
#5555=CARTESIAN_POINT ( 'NONE',  ( 7.270619713743966983, -48.94911951120975857, -150.0552959529999839 ) ) ;
#5566=VECTOR ( 'NONE', #2918, 1000.000000000000000 ) ;
#5568=EDGE_CURVE ( 'NONE', #6870, #2237, #11092, .T. ) ;
#5569=LINE ( 'NONE', #3439, #6840 ) ;
#5573=CARTESIAN_POINT ( 'NONE',  ( 25.50000000000000000, 25.50000000000000000, -150.0552959529999839 ) ) ;
#5577=PLANE ( 'NONE',  #8982 ) ;
#5578=LINE ( 'NONE', #18321, #22999 ) ;
#5583=CARTESIAN_POINT ( 'NONE',  ( -13.86630785140000022, 50.50000000000000000, -137.0552959530000123 ) ) ;
#5585=EDGE_CURVE ( 'NONE', #9664, #9123, #9191, .T. ) ;
#5586=CARTESIAN_POINT ( 'NONE',  ( 25.96278831669999931, 46.03148680889999866, -136.0552959530000123 ) ) ;
#5593=DIRECTION ( 'NONE',  ( 1.000000000000000000, 0.000000000000000000, 0.000000000000000000 ) ) ;
#5594=CARTESIAN_POINT ( 'NONE',  ( 2.100999472805463064, -5.343640159924751387, -150.0552959529999839 ) ) ;
#5596=LINE ( 'NONE', #5125, #16139 ) ;
#5597=VECTOR ( 'NONE', #20282, 1000.000000000000000 ) ;
#5598=ORIENTED_EDGE ( 'NONE', *, *, #21643, .F. ) ;
#5604=ADVANCED_FACE ( 'NONE', ( #636 ), #4323, .T. ) ;
#5612=AXIS2_PLACEMENT_3D ( 'NONE', #19432, #14073, #17880 ) ;
#5622=CARTESIAN_POINT ( 'NONE',  ( 25.31684607429999900, 45.26810052439999765, -150.0552959529999839 ) ) ;
#5628=VECTOR ( 'NONE', #2176, 1000.000000000000000 ) ;
#5629=DIRECTION ( 'NONE',  ( 0.000000000000000000, 0.000000000000000000, -1.000000000000000000 ) ) ;
#5630=VECTOR ( 'NONE', #7562, 1000.000000000000227 ) ;
#5634=CARTESIAN_POINT ( 'NONE',  ( 13.98537695654772328, 33.88080765319283927, -150.0552959530000123 ) ) ;
#5637=DIRECTION ( 'NONE',  ( -2.257144641399999941E-12, 0.000000000000000000, -1.000000000000000000 ) ) ;
#5639=EDGE_CURVE ( 'NONE', #18084, #13274, #15547, .T. ) ;
#5642=ORIENTED_EDGE ( 'NONE', *, *, #20887, .F. ) ;
#5658=AXIS2_PLACEMENT_3D ( 'NONE', #2268, #9494, #11984 ) ;
#5659=ORIENTED_EDGE ( 'NONE', *, *, #10981, .T. ) ;
#5664=CARTESIAN_POINT ( 'NONE',  ( 23.50000000000000000, -20.50000000000000000, -143.5552959529999839 ) ) ;
#5666=CARTESIAN_POINT ( 'NONE',  ( 8.496192186297829352, -48.00965300675227354, -150.0552959530000123 ) ) ;
#5668=VERTEX_POINT ( 'NONE', #13711 ) ;
#5671=LINE ( 'NONE', #13157, #4903 ) ;
#5676=AXIS2_PLACEMENT_3D ( 'NONE', #10975, #14798, #21834 ) ;
#5679=AXIS2_PLACEMENT_3D ( 'NONE', #20484, #4186, #7396 ) ;
#5681=CARTESIAN_POINT ( 'NONE',  ( 10.25767361203778805, 27.00937110137719444, -150.0552959529999839 ) ) ;
#5683=AXIS2_PLACEMENT_3D ( 'NONE', #4959, #12205, #19481 ) ;
#5690=ORIENTED_EDGE ( 'NONE', *, *, #21880, .T. ) ;
#5691=CARTESIAN_POINT ( 'NONE',  ( -15.50000000000000000, 21.50000000000000000, -150.0552959529999839 ) ) ;
#5693=EDGE_CURVE ( 'NONE', #2155, #12574, #19182, .T. ) ;
#5695=DIRECTION ( 'NONE',  ( 0.000000000000000000, 0.000000000000000000, 1.000000000000000000 ) ) ;
#5709=CARTESIAN_POINT ( 'NONE',  ( -31.00000000000000000, -50.00000000000000000, -150.0552959529999839 ) ) ;
#5711=CARTESIAN_POINT ( 'NONE',  ( 7.500000000000000000, -3.500000000000000000, -150.0552959529999839 ) ) ;
#5712=LINE ( 'NONE', #2159, #7678 ) ;
#5714=ORIENTED_EDGE ( 'NONE', *, *, #710, .F. ) ;
#5715=CARTESIAN_POINT ( 'NONE',  ( -10.00000000000000000, 48.50000000000000000, -150.0552959529999839 ) ) ;
#5724=CARTESIAN_POINT ( 'NONE',  ( 31.00000000000000000, -0.7500000000009999779, -149.5552959529999839 ) ) ;
#5733=AXIS2_PLACEMENT_3D ( 'NONE', #21744, #16261, #5432 ) ;
#5734=AXIS2_PLACEMENT_3D ( 'NONE', #10657, #23059, #13894 ) ;
#5738=FACE_OUTER_BOUND ( 'NONE', #17518, .T. ) ;
#5739=CARTESIAN_POINT ( 'NONE',  ( 19.77963439019999825, -51.26338628519999929, -142.8052959529999839 ) ) ;
#5743=DIRECTION ( 'NONE',  ( 0.000000000000000000, -1.000000000000000000, 0.000000000000000000 ) ) ;
#5744=ADVANCED_FACE ( 'NONE', ( #11553 ), #2435, .T. ) ;
#5746=FACE_OUTER_BOUND ( 'NONE', #1088, .T. ) ;
#5748=DIRECTION ( 'NONE',  ( 0.000000000000000000, 1.000000000000000000, 0.000000000000000000 ) ) ;
#5755=CARTESIAN_POINT ( 'NONE',  ( 12.50006728695150926, 36.10251055745180082, -150.0552959529999839 ) ) ;
#5756=DIRECTION ( 'NONE',  ( 0.000000000000000000, -1.000000000000000000, 0.000000000000000000 ) ) ;
#5757=CARTESIAN_POINT ( 'NONE',  ( -3.500000000000000000, 44.50000000000000000, -151.0552959529999839 ) ) ;
#5762=ORIENTED_EDGE ( 'NONE', *, *, #19207, .T. ) ;
#5788=DIRECTION ( 'NONE',  ( 0.000000000000000000, -1.000000000000000000, 0.000000000000000000 ) ) ;
#5791=ORIENTED_EDGE ( 'NONE', *, *, #11985, .T. ) ;
#5798=LINE ( 'NONE', #11371, #14768 ) ;
#5804=DIRECTION ( 'NONE',  ( 0.000000000000000000, -1.000000000000000000, 0.000000000000000000 ) ) ;
#5806=VERTEX_POINT ( 'NONE', #17876 ) ;
#5807=DIRECTION ( 'NONE',  ( 0.000000000000000000, 2.256988247090000272E-12, 1.000000000000000000 ) ) ;
#5813=CARTESIAN_POINT ( 'NONE',  ( -32.50000000000000000, -36.00000000000000000, -150.0552959529999839 ) ) ;
#5818=CARTESIAN_POINT ( 'NONE',  ( 18.95053822279999878, -50.00000000000000000, -149.5552959529999839 ) ) ;
#5823=CARTESIAN_POINT ( 'NONE',  ( 19.77963439019999825, -51.26338628519999929, -142.8052959529999839 ) ) ;
#5827=EDGE_LOOP ( 'NONE', ( #21279, #446, #276, #12698 ) ) ;
#5831=ADVANCED_FACE ( 'NONE', ( #15620 ), #6800, .F. ) ;
#5833=AXIS2_PLACEMENT_3D ( 'NONE', #18620, #16835, #2336 ) ;
#5837=CARTESIAN_POINT ( 'NONE',  ( 32.50000000000000000, -33.03620104880000241, -136.0552959530000123 ) ) ;
#5840=ORIENTED_EDGE ( 'NONE', *, *, #17681, .T. ) ;
#5843=FACE_OUTER_BOUND ( 'NONE', #22466, .T. ) ;
#5856=ORIENTED_EDGE ( 'NONE', *, *, #10165, .T. ) ;
#5857=CARTESIAN_POINT ( 'NONE',  ( -31.00000000000000000, -7.105427357599999217E-15, -149.5552959529999839 ) ) ;
#5860=EDGE_LOOP ( 'NONE', ( #11363, #3982, #1789, #16154 ) ) ;
#5866=CYLINDRICAL_SURFACE ( 'NONE', #7498, 2.000000000000000000 ) ;
#5868=CARTESIAN_POINT ( 'NONE',  ( 4.332174032634473093, -37.80157851245341760, -150.0552959529999555 ) ) ;
#5871=ORIENTED_EDGE ( 'NONE', *, *, #16910, .F. ) ;
#5880=ORIENTED_EDGE ( 'NONE', *, *, #7675, .T. ) ;
#5881=DIRECTION ( 'NONE',  ( 0.000000000000000000, 0.000000000000000000, 1.000000000000000000 ) ) ;
#5889=EDGE_CURVE ( 'NONE', #213, #3522, #13834, .T. ) ;
#5892=ORIENTED_EDGE ( 'NONE', *, *, #15345, .F. ) ;
#5895=VECTOR ( 'NONE', #10342, 1000.000000000000000 ) ;
#5900=ADVANCED_FACE ( 'NONE', ( #19425 ), #5026, .T. ) ;
#5905=DIRECTION ( 'NONE',  ( 0.000000000000000000, -1.000000000000000000, 0.000000000000000000 ) ) ;
#5906=ORIENTED_EDGE ( 'NONE', *, *, #11985, .F. ) ;
#5909=VERTEX_POINT ( 'NONE', #13174 ) ;
#5920=DIRECTION ( 'NONE',  ( 0.000000000000000000, 1.000000000000000000, 2.245315043809999812E-12 ) ) ;
#5926=ORIENTED_EDGE ( 'NONE', *, *, #13843, .F. ) ;
#5929=ORIENTED_EDGE ( 'NONE', *, *, #22327, .F. ) ;
#5930=DIRECTION ( 'NONE',  ( 0.000000000000000000, 0.000000000000000000, -1.000000000000000000 ) ) ;
#5933=ORIENTED_EDGE ( 'NONE', *, *, #10246, .T. ) ;
#5934=DIRECTION ( 'NONE',  ( 3.494344380199214996E-12, 0.000000000000000000, -1.000000000000000000 ) ) ;
#5939=ORIENTED_EDGE ( 'NONE', *, *, #21313, .T. ) ;
#5943=DIRECTION ( 'NONE',  ( -1.000000000000000000, 0.000000000000000000, 2.245315044999999693E-12 ) ) ;
#5949=ORIENTED_EDGE ( 'NONE', *, *, #14618, .F. ) ;
#5973=FACE_BOUND ( 'NONE', #1281, .T. ) ;
#5974=EDGE_LOOP ( 'NONE', ( #15184, #2605, #17443, #16857 ) ) ;
#5985=DIRECTION ( 'NONE',  ( -1.000000000000000000, 0.000000000000000000, 2.257144641399999941E-12 ) ) ;
#5986=ORIENTED_EDGE ( 'NONE', *, *, #368, .T. ) ;
#5997=ORIENTED_EDGE ( 'NONE', *, *, #3334, .T. ) ;
#5998=CARTESIAN_POINT ( 'NONE',  ( 7.750000000000000000, -42.23606797749999942, -151.0552959529999839 ) ) ;
#6002=VERTEX_POINT ( 'NONE', #17994 ) ;
#6008=LINE ( 'NONE', #13261, #16239 ) ;
#6009=EDGE_LOOP ( 'NONE', ( #2537, #6884, #3824, #21235 ) ) ;
#6011=CARTESIAN_POINT ( 'NONE',  ( -32.50000000000000000, -36.00000000000000000, -143.3052959529999839 ) ) ;
#6014=CARTESIAN_POINT ( 'NONE',  ( 6.485119744325247737, -49.00006725843046951, -150.0552959529999839 ) ) ;
#6016=EDGE_LOOP ( 'NONE', ( #1645, #22299, #480, #15898 ) ) ;
#6021=ORIENTED_EDGE ( 'NONE', *, *, #12130, .T. ) ;
#6022=CARTESIAN_POINT ( 'NONE',  ( -11.99999999999999467, -43.39269908169870860, -150.0552959529999555 ) ) ;
#6029=EDGE_CURVE ( 'NONE', #1030, #23189, #244, .T. ) ;
#6030=DIRECTION ( 'NONE',  ( -0.7633862853691523176, -0.6459422414661291079, 0.000000000000000000 ) ) ;
#6047=PLANE ( 'NONE',  #3321 ) ;
#6051=CARTESIAN_POINT ( 'NONE',  ( -31.00000000000000000, -7.105427357599999217E-15, -149.5552959529999839 ) ) ;
#6056=ORIENTED_EDGE ( 'NONE', *, *, #6974, .T. ) ;
#6057=DIRECTION ( 'NONE',  ( -1.000000000000000000, 0.000000000000000000, 2.257144641399999941E-12 ) ) ;
#6067=CARTESIAN_POINT ( 'NONE',  ( 31.50000000000000000, 0.000000000000000000, -150.0552959529999839 ) ) ;
#6072=DIRECTION ( 'NONE',  ( -1.000000000000000000, 0.000000000000000000, 0.000000000000000000 ) ) ;
#6085=DIRECTION ( 'NONE',  ( 1.000000000000000000, 0.000000000000000000, 0.000000000000000000 ) ) ;
#6087=CARTESIAN_POINT ( 'NONE',  ( -16.50000000000000711, -42.80091057724988701, -150.0552959530000123 ) ) ;
#6099=FACE_BOUND ( 'NONE', #1758, .T. ) ;
#6100=ORIENTED_EDGE ( 'NONE', *, *, #4204, .F. ) ;
#6107=CARTESIAN_POINT ( 'NONE',  ( 2.742326387956447231, 13.99062889862865156, -150.0552959529999839 ) ) ;
#6126=EDGE_CURVE ( 'NONE', #18702, #14107, #6626, .T. ) ;
#6130=CARTESIAN_POINT ( 'NONE',  ( 31.50000000000000000, 0.000000000000000000, -136.0552959530000123 ) ) ;
#6132=ORIENTED_EDGE ( 'NONE', *, *, #12829, .T. ) ;
#6133=CARTESIAN_POINT ( 'NONE',  ( 32.00000000000000000, -21.03620104879999886, -137.0552959530000123 ) ) ;
#6136=VECTOR ( 'NONE', #8553, 1000.000000000000000 ) ;
#6138=VECTOR ( 'NONE', #21959, 1000.000000000000000 ) ;
#6140=( LENGTH_UNIT ( ) NAMED_UNIT ( * ) SI_UNIT ( .MILLI., .METRE. ) );
#6143=ORIENTED_EDGE ( 'NONE', *, *, #17903, .T. ) ;
#6146=EDGE_CURVE ( 'NONE', #968, #18797, #822, .T. ) ;
#6157=AXIS2_PLACEMENT_3D ( 'NONE', #5818, #22241, #2151 ) ;
#6161=ORIENTED_EDGE ( 'NONE', *, *, #19673, .F. ) ;
#6168=ORIENTED_EDGE ( 'NONE', *, *, #18589, .T. ) ;
#6170=LINE ( 'NONE', #13421, #12610 ) ;
#6172=FACE_OUTER_BOUND ( 'NONE', #17970, .T. ) ;
#6179=EDGE_CURVE ( 'NONE', #11337, #14361, #2828, .T. ) ;
#6181=EDGE_LOOP ( 'NONE', ( #21491, #5511, #16663, #14229 ) ) ;
#6182=DIRECTION ( 'NONE',  ( 0.000000000000000000, 1.000000000000000000, 0.000000000000000000 ) ) ;
#6184=DIRECTION ( 'NONE',  ( -1.000000000000000000, 0.000000000000000000, 2.257144641399999941E-12 ) ) ;
#6191=DIRECTION ( 'NONE',  ( -1.000000000000000000, 0.000000000000000000, 2.257144641399999941E-12 ) ) ;
#6192=VERTEX_POINT ( 'NONE', #1882 ) ;
#6194=DIRECTION ( 'NONE',  ( 0.000000000000000000, 0.000000000000000000, 1.000000000000000000 ) ) ;
#6196=DIRECTION ( 'NONE',  ( 0.000000000000000000, -1.000000000000000000, 0.000000000000000000 ) ) ;
#6198=ORIENTED_EDGE ( 'NONE', *, *, #1029, .T. ) ;
#6199=LINE ( 'NONE', #22266, #11656 ) ;
#6200=PLANE ( 'NONE',  #17302 ) ;
#6210=CARTESIAN_POINT ( 'NONE',  ( -10.00000000000000000, 42.50000000000000000, -151.0552959529999839 ) ) ;
#6223=CARTESIAN_POINT ( 'NONE',  ( -1.000000000000000222, 20.00701398444616785, -150.0552959529999839 ) ) ;
#6224=DIRECTION ( 'NONE',  ( 0.000000000000000000, 0.000000000000000000, -1.000000000000000000 ) ) ;
#6235=CARTESIAN_POINT ( 'NONE',  ( -6.683153925719999222, -50.50000000000000000, -150.0552959529999839 ) ) ;
#6237=EDGE_LOOP ( 'NONE', ( #17727, #6523, #19912, #20247 ) ) ;
#6247=CARTESIAN_POINT ( 'NONE',  ( 3.038350857853684861, -3.890616787572018342, -150.0552959529999839 ) ) ;
#6249=PLANE ( 'NONE',  #7285 ) ;
#6258=CARTESIAN_POINT ( 'NONE',  ( 13.13369214859999978, -50.50000000000000000, -143.0552959529999839 ) ) ;
#6266=CARTESIAN_POINT ( 'NONE',  ( -13.86630785140000022, 50.50000000000000000, -137.0552959530000123 ) ) ;
#6268=VERTEX_POINT ( 'NONE', #14128 ) ;
#6269=CARTESIAN_POINT ( 'NONE',  ( -6.683153925719999222, -50.50000000000000000, -136.0552959530000123 ) ) ;
#6271=CARTESIAN_POINT ( 'NONE',  ( 22.89765167458959283, 39.50000000000000000, -150.0552959530000123 ) ) ;
#6281=CARTESIAN_POINT ( 'NONE',  ( 23.10730091830129140, -23.50000000000000355, -150.0552959529999839 ) ) ;
#6285=ADVANCED_FACE ( 'NONE', ( #7224 ), #9107, .F. ) ;
#6286=ORIENTED_EDGE ( 'NONE', *, *, #710, .T. ) ;
#6288=LINE ( 'NONE', #8068, #21304 ) ;
#6291=AXIS2_PLACEMENT_3D ( 'NONE', #15598, #17728, #3219 ) ;
#6300=ORIENTED_EDGE ( 'NONE', *, *, #15268, .T. ) ;
#6304=LINE ( 'NONE', #13557, #8144 ) ;
#6310=CARTESIAN_POINT ( 'NONE',  ( 19.16617820230000291, 49.81753540199999719, -149.5552959529999839 ) ) ;
#6312=CARTESIAN_POINT ( 'NONE',  ( -16.30945103002074958, -42.24260211602405235, -150.0552959530000123 ) ) ;
#6313=CARTESIAN_POINT ( 'NONE',  ( -31.50000000000000000, -43.00000000000000000, -149.5552959529999839 ) ) ;
#6314=CARTESIAN_POINT ( 'NONE',  ( 31.50000000000000000, 39.80430157320000006, -150.0552959529999839 ) ) ;
#6327=EDGE_CURVE ( 'NONE', #4645, #21739, #23291, .T. ) ;
#6336=CARTESIAN_POINT ( 'NONE',  ( -0.2408409772196719867, 17.17512194927157410, -150.0552959529999839 ) ) ;
#6340=EDGE_CURVE ( 'NONE', #537, #2949, #21187, .T. ) ;
#6342=CARTESIAN_POINT ( 'NONE',  ( 8.201139657833619978, -33.35711941572422745, -150.0552959529999839 ) ) ;
#6345=CIRCLE ( 'NONE', #11640, 0.5000000000000004441 ) ;
#6349=DIRECTION ( 'NONE',  ( 0.000000000000000000, 0.000000000000000000, -1.000000000000000000 ) ) ;
#6355=CARTESIAN_POINT ( 'NONE',  ( -6.683153925719999222, -51.50000000000000000, -136.0552959530000123 ) ) ;
#6360=CYLINDRICAL_SURFACE ( 'NONE', #19978, 2.999999999999999112 ) ;
#6361=EDGE_CURVE ( 'NONE', #21164, #4735, #1811, .T. ) ;
#6366=VECTOR ( 'NONE', #11101, 1000.000000000000000 ) ;
#6371=VECTOR ( 'NONE', #5475, 1000.000000000000000 ) ;
#6385=EDGE_CURVE ( 'NONE', #23438, #21392, #6008, .T. ) ;
#6388=DIRECTION ( 'NONE',  ( -1.000000000000000000, 0.000000000000000000, 0.000000000000000000 ) ) ;
#6389=ADVANCED_FACE ( 'NONE', ( #3892 ), #20538, .F. ) ;
#6390=ORIENTED_EDGE ( 'NONE', *, *, #11820, .T. ) ;
#6394=PLANE ( 'NONE',  #2134 ) ;
#6403=DIRECTION ( 'NONE',  ( 0.000000000000000000, 1.000000000000000000, 0.000000000000000000 ) ) ;
#6404=VERTEX_POINT ( 'NONE', #20197 ) ;
#6412=AXIS2_PLACEMENT_3D ( 'NONE', #21535, #19865, #3796 ) ;
#6414=LINE ( 'NONE', #1207, #20872 ) ;
#6415=ORIENTED_EDGE ( 'NONE', *, *, #9056, .F. ) ;
#6430=CARTESIAN_POINT ( 'NONE',  ( 25.01085694111269930, -17.87864083493722944, -150.0552959529999839 ) ) ;
#6431=CARTESIAN_POINT ( 'NONE',  ( -13.50000000000000000, -43.00000000000000000, -150.0552959529999839 ) ) ;
#6440=CARTESIAN_POINT ( 'NONE',  ( -31.00000000000000000, 1.000000000000000000, -151.0552959529999839 ) ) ;
#6442=EDGE_CURVE ( 'NONE', #20932, #12161, #9445, .T. ) ;
#6447=CARTESIAN_POINT ( 'NONE',  ( 4.890549297259640937, -2.038177252827572339, -150.0552959529999839 ) ) ;
#6452=VECTOR ( 'NONE', #21559, 1000.000000000000000 ) ;
#6453=CARTESIAN_POINT ( 'NONE',  ( -32.50000000000000000, 19.50000000000000000, -149.5552959529999839 ) ) ;
#6454=ADVANCED_FACE ( 'NONE', ( #11123 ), #313, .F. ) ;
#6459=CARTESIAN_POINT ( 'NONE',  ( 5.519360106948777656, 13.04803137664723423, -150.0552959530000123 ) ) ;
#6465=EDGE_LOOP ( 'NONE', ( #22973, #12741, #19625, #6100 ) ) ;
#6470=VERTEX_POINT ( 'NONE', #9224 ) ;
#6472=CARTESIAN_POINT ( 'NONE',  ( 19.77963439019999825, 51.26338628519999929, -136.0552959530000123 ) ) ;
#6475=VERTEX_POINT ( 'NONE', #13146 ) ;
#6484=CARTESIAN_POINT ( 'NONE',  ( -12.00000000000000000, -43.00000000000000000, -150.0552959529999839 ) ) ;
#6487=AXIS2_PLACEMENT_3D ( 'NONE', #16145, #1523, #8747 ) ;
#6488=LINE ( 'NONE', #6130, #16926 ) ;
#6490=CARTESIAN_POINT ( 'NONE',  ( 5.700859806000233121, -4.419886383052269885, -150.0552959530000123 ) ) ;
#6495=ORIENTED_EDGE ( 'NONE', *, *, #15071, .F. ) ;
#6501=AXIS2_PLACEMENT_3D ( 'NONE', #16388, #14489, #12688 ) ;
#6504=DIRECTION ( 'NONE',  ( 0.000000000000000000, -1.000000000000000000, 0.000000000000000000 ) ) ;
#6509=DIRECTION ( 'NONE',  ( 1.000000000000000000, 0.000000000000000000, -2.257560236040000027E-12 ) ) ;
#6510=EDGE_LOOP ( 'NONE', ( #2733, #12339, #16089, #16614 ) ) ;
#6511=CARTESIAN_POINT ( 'NONE',  ( -6.683153925719999222, 50.50000000000000000, -150.0552959529999839 ) ) ;
#6515=ORIENTED_EDGE ( 'NONE', *, *, #78, .F. ) ;
#6523=ORIENTED_EDGE ( 'NONE', *, *, #13448, .T. ) ;
#6526=VERTEX_POINT ( 'NONE', #1736 ) ;
#6533=CARTESIAN_POINT ( 'NONE',  ( 32.50000000000000000, 39.92025131090000656, -150.0552959529999839 ) ) ;
#6539=ORIENTED_EDGE ( 'NONE', *, *, #25, .F. ) ;
#6540=ORIENTED_EDGE ( 'NONE', *, *, #3889, .F. ) ;
#6546=LINE ( 'NONE', #13814, #14364 ) ;
#6549=CARTESIAN_POINT ( 'NONE',  ( 21.65635984007525394, -18.10099947280546573, -150.0552959529999839 ) ) ;
#6553=ORIENTED_EDGE ( 'NONE', *, *, #9782, .T. ) ;
#6554=LINE ( 'NONE', #13930, #17922 ) ;
#6566=ORIENTED_EDGE ( 'NONE', *, *, #22379, .F. ) ;
#6567=AXIS2_PLACEMENT_3D ( 'NONE', #4668, #2884, #21092 ) ;
#6568=CARTESIAN_POINT ( 'NONE',  ( -10.00000000000000000, 19.50000000000000000, -151.0552959529999839 ) ) ;
#6569=LINE ( 'NONE', #19067, #15555 ) ;
#6573=DIRECTION ( 'NONE',  ( 1.000000000000000000, 0.000000000000000000, 0.000000000000000000 ) ) ;
#6577=DIRECTION ( 'NONE',  ( 0.000000000000000000, -1.000000000000000000, 0.000000000000000000 ) ) ;
#6578=CARTESIAN_POINT ( 'NONE',  ( 4.204281436780199499, -34.38417682219860438, -150.0552959529999839 ) ) ;
#6597=DIRECTION ( 'NONE',  ( 1.000000000000000000, 0.000000000000000000, -2.257453483404485639E-12 ) ) ;
#6600=CYLINDRICAL_SURFACE ( 'NONE', #1783, 2.999999999999999112 ) ;
#6602=ORIENTED_EDGE ( 'NONE', *, *, #12420, .T. ) ;
#6603=DIRECTION ( 'NONE',  ( 2.257242012349999735E-12, 0.000000000000000000, -1.000000000000000000 ) ) ;
#6609=VERTEX_POINT ( 'NONE', #18263 ) ;
#6613=ORIENTED_EDGE ( 'NONE', *, *, #21402, .T. ) ;
#6614=VECTOR ( 'NONE', #21712, 1000.000000000000000 ) ;
#6615=DIRECTION ( 'NONE',  ( 1.000000000000000000, 0.000000000000000000, 0.000000000000000000 ) ) ;
#6624=ADVANCED_FACE ( 'NONE', ( #7651 ), #2086, .F. ) ;
#6626=LINE ( 'NONE', #15556, #9834 ) ;
#6627=ORIENTED_EDGE ( 'NONE', *, *, #19817, .T. ) ;
#6628=EDGE_CURVE ( 'NONE', #3906, #21536, #9419, .T. ) ;
#6629=EDGE_CURVE ( 'NONE', #2237, #20657, #411, .T. ) ;
#6648=LINE ( 'NONE', #1320, #9806 ) ;
#6650=AXIS2_PLACEMENT_3D ( 'NONE', #15116, #21192, #10092 ) ;
#6659=CARTESIAN_POINT ( 'NONE',  ( 13.13369214859999978, -50.50000000000000000, -137.0552959530000123 ) ) ;
#6667=VERTEX_POINT ( 'NONE', #4088 ) ;
#6669=DIRECTION ( 'NONE',  ( -1.000000000000000000, 0.000000000000000000, 0.000000000000000000 ) ) ;
#6672=DIRECTION ( 'NONE',  ( -0.000000000000000000, 1.000000000000000000, 0.000000000000000000 ) ) ;
#6678=CIRCLE ( 'NONE', #14673, 1.500000000000001332 ) ;
#6680=VECTOR ( 'NONE', #16467, 1000.000000000000000 ) ;
#6682=ORIENTED_EDGE ( 'NONE', *, *, #18429, .T. ) ;
#6685=EDGE_CURVE ( 'NONE', #22568, #14539, #65, .T. ) ;
#6691=EDGE_CURVE ( 'NONE', #6609, #4038, #4485, .T. ) ;
#6692=CARTESIAN_POINT ( 'NONE',  ( 4.084326842523585910, 27.61765588495835644, -150.0552959529999839 ) ) ;
#6693=LINE ( 'NONE', #5140, #2975 ) ;
#6695=ORIENTED_EDGE ( 'NONE', *, *, #9122, .T. ) ;
#6703=EDGE_LOOP ( 'NONE', ( #14346, #15084, #13232, #8890 ) ) ;
#6707=FACE_OUTER_BOUND ( 'NONE', #2578, .T. ) ;
#6717=CARTESIAN_POINT ( 'NONE',  ( 19.00000000000000000, 39.50000000000000000, -150.0552959529999839 ) ) ;
#6719=FACE_OUTER_BOUND ( 'NONE', #3345, .T. ) ;
#6721=ORIENTED_EDGE ( 'NONE', *, *, #10981, .F. ) ;
#6728=AXIS2_PLACEMENT_3D ( 'NONE', #18397, #21866, #18750 ) ;
#6753=EDGE_CURVE ( 'NONE', #5050, #19419, #8729, .T. ) ;
#6763=CARTESIAN_POINT ( 'NONE',  ( 25.96278831649999930, -46.03148680910000223, -136.0552959530000123 ) ) ;
#6766=LINE ( 'NONE', #4643, #714 ) ;
#6767=ADVANCED_FACE ( 'NONE', ( #17402 ), #2783, .F. ) ;
#6769=ORIENTED_EDGE ( 'NONE', *, *, #17380, .T. ) ;
#6774=LINE ( 'NONE', #4878, #4923 ) ;
#6779=PLANE ( 'NONE',  #23185 ) ;
#6782=DIRECTION ( 'NONE',  ( -2.256988247010000033E-12, 0.000000000000000000, 1.000000000000000000 ) ) ;
#6787=VECTOR ( 'NONE', #13060, 1000.000000000000000 ) ;
#6799=DIRECTION ( 'NONE',  ( 0.000000000000000000, 0.000000000000000000, -1.000000000000000000 ) ) ;
#6800=PLANE ( 'NONE',  #20891 ) ;
#6802=VECTOR ( 'NONE', #5015, 1000.000000000000000 ) ;
#6810=CARTESIAN_POINT ( 'NONE',  ( -1.000000000000000222, 20.99262443222763608, -150.0552959530000123 ) ) ;
#6812=LINE ( 'NONE', #6133, #4994 ) ;
#6814=LINE ( 'NONE', #8118, #15240 ) ;
#6821=VECTOR ( 'NONE', #16019, 1000.000000000000227 ) ;
#6832=DIRECTION ( 'NONE',  ( 0.000000000000000000, 0.000000000000000000, 1.000000000000000000 ) ) ;
#6833=LINE ( 'NONE', #17780, #15412 ) ;
#6837=CARTESIAN_POINT ( 'NONE',  ( 31.50000000010000178, 40.03620104870000063, -143.0552959529999839 ) ) ;
#6840=VECTOR ( 'NONE', #16053, 1000.000000000000000 ) ;
#6844=ORIENTED_EDGE ( 'NONE', *, *, #2138, .T. ) ;
#6847=CARTESIAN_POINT ( 'NONE',  ( -12.50000000000000000, 25.50000000000000000, -150.5552959529999839 ) ) ;
#6851=CARTESIAN_POINT ( 'NONE',  ( -4.499932713042313459, 22.10251055751543348, -150.0552959529999839 ) ) ;
#6865=VERTEX_POINT ( 'NONE', #10258 ) ;
#6868=VECTOR ( 'NONE', #5144, 1000.000000000000000 ) ;
#6870=VERTEX_POINT ( 'NONE', #8692 ) ;
#6872=CARTESIAN_POINT ( 'NONE',  ( 26.12135916506278122, -22.01085694111269220, -150.0552959529999839 ) ) ;
#6873=VERTEX_POINT ( 'NONE', #15973 ) ;
#6875=CARTESIAN_POINT ( 'NONE',  ( -12.50000000000000000, 48.50000000000000000, -151.0552959529999839 ) ) ;
#6876=ORIENTED_EDGE ( 'NONE', *, *, #104, .F. ) ;
#6883=LINE ( 'NONE', #17960, #2253 ) ;
#6884=ORIENTED_EDGE ( 'NONE', *, *, #605, .T. ) ;
#6886=VECTOR ( 'NONE', #6986, 1000.000000000000000 ) ;
#6889=EDGE_CURVE ( 'NONE', #21170, #7540, #2180, .T. ) ;
#6898=ADVANCED_FACE ( 'NONE', ( #22997 ), #14189, .T. ) ;
#6923=EDGE_LOOP ( 'NONE', ( #17541, #21523, #19105, #5321 ) ) ;
#6926=CARTESIAN_POINT ( 'NONE',  ( -13.50000000000000000, -43.00000000000000000, -145.5552959529999839 ) ) ;
#6938=PLANE ( 'NONE',  #19812 ) ;
#6943=VECTOR ( 'NONE', #19420, 1000.000000000000000 ) ;
#6949=FACE_OUTER_BOUND ( 'NONE', #17833, .T. ) ;
#6955=DIRECTION ( 'NONE',  ( 0.000000000000000000, 0.000000000000000000, 1.000000000000000000 ) ) ;
#6962=VERTEX_POINT ( 'NONE', #17998 ) ;
#6974=EDGE_CURVE ( 'NONE', #7890, #17493, #23096, .T. ) ;
#6976=CARTESIAN_POINT ( 'NONE',  ( 18.95053822279999878, -50.00000000000000000, -149.5552959529999839 ) ) ;
#6986=DIRECTION ( 'NONE',  ( 2.255973186040000320E-12, 0.000000000000000000, 1.000000000000000000 ) ) ;
#6990=CARTESIAN_POINT ( 'NONE',  ( -31.00000000000000000, 1.000000000000000000, -150.0552959529999839 ) ) ;
#6991=EDGE_LOOP ( 'NONE', ( #7990, #18897, #23423, #18722 ) ) ;
#6992=CARTESIAN_POINT ( 'NONE',  ( 22.00000000000000000, -20.50000000000000000, -137.0552959530000123 ) ) ;
#7004=DIRECTION ( 'NONE',  ( -1.000000000000000000, 0.000000000000000000, -1.457985068979999943E-12 ) ) ;
#7018=DIRECTION ( 'NONE',  ( 0.000000000000000000, -1.000000000000000000, 0.000000000000000000 ) ) ;
#7025=ADVANCED_FACE ( 'NONE', ( #11070 ), #18572, .F. ) ;
#7026=VECTOR ( 'NONE', #3744, 1000.000000000000000 ) ;
#7033=ORIENTED_EDGE ( 'NONE', *, *, #7758, .T. ) ;
#7034=EDGE_CURVE ( 'NONE', #6268, #18451, #2171, .T. ) ;
#7041=VECTOR ( 'NONE', #970, 1000.000000000000000 ) ;
#7042=ORIENTED_EDGE ( 'NONE', *, *, #16058, .F. ) ;
#7053=VERTEX_POINT ( 'NONE', #4061 ) ;
#7054=CARTESIAN_POINT ( 'NONE',  ( -7.500000000000000000, 22.50000000000000000, -150.0552959529999839 ) ) ;
#7060=DIRECTION ( 'NONE',  ( 0.000000000000000000, 0.000000000000000000, 1.000000000000000000 ) ) ;
#7066=CARTESIAN_POINT ( 'NONE',  ( 17.50006728695150215, 22.10251055745073501, -150.0552959529999839 ) ) ;
#7067=ADVANCED_FACE ( 'NONE', ( #19902, #7395 ), #9517, .T. ) ;
#7068=CARTESIAN_POINT ( 'NONE',  ( -13.69054896997999826, -43.75739788393685359, -150.0552959529999839 ) ) ;
#7069=CARTESIAN_POINT ( 'NONE',  ( 3.000000000000000000, -3.500000000000000000, -145.5552959529999839 ) ) ;
#7075=CYLINDRICAL_SURFACE ( 'NONE', #22297, 2.000000000000001776 ) ;
#7077=FACE_OUTER_BOUND ( 'NONE', #4271, .T. ) ;
#7080=AXIS2_PLACEMENT_3D ( 'NONE', #18373, #10857, #18139 ) ;
#7088=CARTESIAN_POINT ( 'NONE',  ( -15.00000000000000000, -43.00000000000000000, -145.5552959529999839 ) ) ;
#7089=ORIENTED_EDGE ( 'NONE', *, *, #3711, .F. ) ;
#7096=ORIENTED_EDGE ( 'NONE', *, *, #5237, .T. ) ;
#7104=VERTEX_POINT ( 'NONE', #503 ) ;
#7106=DIRECTION ( 'NONE',  ( 1.000000000000000000, 0.000000000000000000, 0.000000000000000000 ) ) ;
#7111=LINE ( 'NONE', #12577, #19741 ) ;
#7127=VECTOR ( 'NONE', #19277, 1000.000000000000000 ) ;
#7129=CARTESIAN_POINT ( 'NONE',  ( -15.50000000000000000, 0.000000000000000000, -150.0552959529999839 ) ) ;
#7134=FACE_OUTER_BOUND ( 'NONE', #23306, .T. ) ;
#7135=DIRECTION ( 'NONE',  ( 2.257144641399999941E-12, 0.000000000000000000, -1.000000000000000000 ) ) ;
#7137=DIRECTION ( 'NONE',  ( 1.000000000000000000, 0.000000000000000000, 0.000000000000000000 ) ) ;
#7138=LINE ( 'NONE', #19883, #8023 ) ;
#7139=DIRECTION ( 'NONE',  ( 0.6459422414661276646, -0.7633862853691535388, 2.257453483404482811E-12 ) ) ;
#7143=DIRECTION ( 'NONE',  ( 0.000000000000000000, 0.000000000000000000, 1.000000000000000000 ) ) ;
#7151=ADVANCED_FACE ( 'NONE', ( #13208 ), #17015, .T. ) ;
#7152=ORIENTED_EDGE ( 'NONE', *, *, #2280, .F. ) ;
#7154=ORIENTED_EDGE ( 'NONE', *, *, #12164, .F. ) ;
#7156=AXIS2_PLACEMENT_3D ( 'NONE', #20189, #3885, #11118 ) ;
#7181=VECTOR ( 'NONE', #4287, 1000.000000000000000 ) ;
#7186=FACE_OUTER_BOUND ( 'NONE', #21980, .T. ) ;
#7194=VECTOR ( 'NONE', #2930, 1000.000000000000000 ) ;
#7203=CARTESIAN_POINT ( 'NONE',  ( 18.95053822279999878, -50.00000000000000000, -150.0552959529999839 ) ) ;
#7207=EDGE_CURVE ( 'NONE', #10920, #22797, #22724, .T. ) ;
#7208=ORIENTED_EDGE ( 'NONE', *, *, #9532, .T. ) ;
#7209=CARTESIAN_POINT ( 'NONE',  ( -4.576286989421689988, 23.28076054106537995, -150.0552959529999839 ) ) ;
#7213=DIRECTION ( 'NONE',  ( 1.000000000000000000, 0.000000000000000000, 0.000000000000000000 ) ) ;
#7223=AXIS2_PLACEMENT_3D ( 'NONE', #17717, #14616, #10788 ) ;
#7224=FACE_OUTER_BOUND ( 'NONE', #22650, .T. ) ;
#7226=CARTESIAN_POINT ( 'NONE',  ( -32.50000000000000000, 1.000000000000000000, -150.5552959529999839 ) ) ;
#7233=VERTEX_POINT ( 'NONE', #11418 ) ;
#7235=EDGE_CURVE ( 'NONE', #1424, #19480, #22503, .T. ) ;
#7245=DIRECTION ( 'NONE',  ( 1.000000000000000000, 0.000000000000000000, 2.273736754430000208E-12 ) ) ;
#7256=ORIENTED_EDGE ( 'NONE', *, *, #9804, .F. ) ;
#7257=DIRECTION ( 'NONE',  ( -0.000000000000000000, 1.000000000000000000, 0.000000000000000000 ) ) ;
#7258=DIRECTION ( 'NONE',  ( 0.000000000000000000, -1.000000000000000000, -2.273736754430000208E-12 ) ) ;
#7262=ADVANCED_FACE ( 'NONE', ( #17139 ), #22382, .F. ) ;
#7263=FACE_OUTER_BOUND ( 'NONE', #13171, .T. ) ;
#7267=PLANE ( 'NONE',  #9447 ) ;
#7275=LINE ( 'NONE', #14541, #9412 ) ;
#7278=ORIENTED_EDGE ( 'NONE', *, *, #13860, .T. ) ;
#7284=CARTESIAN_POINT ( 'NONE',  ( -32.00000000000000000, 1.000000000000000000, -149.5552959529999839 ) ) ;
#7285=AXIS2_PLACEMENT_3D ( 'NONE', #8020, #16960, #18635 ) ;
#7288=AXIS2_PLACEMENT_3D ( 'NONE', #9502, #12967, #6184 ) ;
#7296=CYLINDRICAL_SURFACE ( 'NONE', #15274, 2.999999999999999112 ) ;
#7298=DIRECTION ( 'NONE',  ( 1.000000000000000000, 0.000000000000000000, 0.000000000000000000 ) ) ;
#7310=DIRECTION ( 'NONE',  ( 0.000000000000000000, -3.386641135243274558E-17, -1.000000000000000000 ) ) ;
#7311=CARTESIAN_POINT ( 'NONE',  ( 15.50000000000000000, 33.50000000000000000, -150.0552959529999839 ) ) ;
#7312=CARTESIAN_POINT ( 'NONE',  ( 31.50000000000000000, 0.000000000000000000, -150.0552959529999839 ) ) ;
#7314=DIRECTION ( 'NONE',  ( -1.000000000000000000, 0.000000000000000000, 2.257144641399999941E-12 ) ) ;
#7318=AXIS2_PLACEMENT_3D ( 'NONE', #1316, #11994, #2971 ) ;
#7321=CARTESIAN_POINT ( 'NONE',  ( 31.00000000000000000, -39.80430157320000006, -150.0552959529999839 ) ) ;
#7325=ORIENTED_EDGE ( 'NONE', *, *, #21302, .T. ) ;
#7336=DIRECTION ( 'NONE',  ( -1.000000000000000000, 0.000000000000000000, 0.000000000000000000 ) ) ;
#7338=ORIENTED_EDGE ( 'NONE', *, *, #9640, .T. ) ;
#7343=CARTESIAN_POINT ( 'NONE',  ( 4.750000000000000888, -47.26539404904927721, -150.0552959529999839 ) ) ;
#7344=DIRECTION ( 'NONE',  ( 1.000000000000000000, 0.000000000000000000, 0.000000000000000000 ) ) ;
#7349=DIRECTION ( 'NONE',  ( -0.6459422414661292189, 0.7633862853691524286, 0.000000000000000000 ) ) ;
#7351=ORIENTED_EDGE ( 'NONE', *, *, #21266, .T. ) ;
#7354=CARTESIAN_POINT ( 'NONE',  ( -12.50000000000000000, 45.50000000000000000, -151.0552959529999839 ) ) ;
#7355=ADVANCED_FACE ( 'NONE', ( #9953 ), #6047, .F. ) ;
#7359=FACE_OUTER_BOUND ( 'NONE', #15769, .T. ) ;
#7360=FACE_OUTER_BOUND ( 'NONE', #21658, .T. ) ;
#7365=ADVANCED_FACE ( 'NONE', ( #15216 ), #14974, .T. ) ;
#7366=VERTEX_POINT ( 'NONE', #9710 ) ;
#7379=EDGE_LOOP ( 'NONE', ( #5208, #21850, #12497, #18957 ) ) ;
#7380=LINE ( 'NONE', #5120, #17148 ) ;
#7382=CARTESIAN_POINT ( 'NONE',  ( 7.500000000000002665, -3.892699081698711705, -150.0552959529999839 ) ) ;
#7391=ADVANCED_FACE ( 'NONE', ( #9829 ), #17108, .T. ) ;
#7393=CARTESIAN_POINT ( 'NONE',  ( -32.50000000000000000, -43.00000000050000182, -137.0552959530000123 ) ) ;
#7395=FACE_OUTER_BOUND ( 'NONE', #22104, .T. ) ;
#7396=DIRECTION ( 'NONE',  ( 1.000000000000000000, 0.000000000000000000, 0.000000000000000000 ) ) ;
#7397=VERTEX_POINT ( 'NONE', #10864 ) ;
#7400=CARTESIAN_POINT ( 'NONE',  ( 31.00000000000000000, -39.80430157320000006, -149.5552959529999839 ) ) ;
#7404=DIRECTION ( 'NONE',  ( 0.000000000000000000, 0.000000000000000000, 1.000000000000000000 ) ) ;
#7405=FACE_OUTER_BOUND ( 'NONE', #9854, .T. ) ;
#7406=CARTESIAN_POINT ( 'NONE',  ( 32.50000000000000000, -36.53620104889999709, -136.0552959530000123 ) ) ;
#7407=VERTEX_POINT ( 'NONE', #21605 ) ;
#7409=VERTEX_POINT ( 'NONE', #17913 ) ;
#7412=ADVANCED_FACE ( 'NONE', ( #19241 ), #12539, .T. ) ;
#7416=EDGE_CURVE ( 'NONE', #11512, #21536, #21578, .T. ) ;
#7418=PLANE ( 'NONE',  #7080 ) ;
#7422=CARTESIAN_POINT ( 'NONE',  ( 6.750000000000000000, -47.00000000000000000, -150.0552959529999839 ) ) ;
#7423=DIRECTION ( 'NONE',  ( -1.000000000000000000, 0.000000000000000000, 0.000000000000000000 ) ) ;
#7429=ORIENTED_EDGE ( 'NONE', *, *, #78, .T. ) ;
#7440=ADVANCED_FACE ( 'NONE', ( #7077 ), #22824, .F. ) ;
#7443=DIRECTION ( 'NONE',  ( 1.000000000000000000, 0.000000000000000000, 0.000000000000000000 ) ) ;
#7461=VECTOR ( 'NONE', #8312, 1000.000000000000000 ) ;
#7468=EDGE_CURVE ( 'NONE', #3293, #5505, #8848, .T. ) ;
#7469=CARTESIAN_POINT ( 'NONE',  ( 25.50000000000000000, 22.50000000000000000, -150.0552959529999839 ) ) ;
#7471=FACE_OUTER_BOUND ( 'NONE', #6009, .T. ) ;
#7478=CARTESIAN_POINT ( 'NONE',  ( 18.95053822279999878, 50.00000000000000000, -149.5552959529999839 ) ) ;
#7480=DIRECTION ( 'NONE',  ( 1.000000000000000000, 0.000000000000000000, 0.000000000000000000 ) ) ;
#7481=DIRECTION ( 'NONE',  ( -0.000000000000000000, 1.000000000000000000, 0.000000000000000000 ) ) ;
#7483=DIRECTION ( 'NONE',  ( 0.6459422414661292189, 0.7633862853691524286, 2.257144641400453113E-12 ) ) ;
#7492=DIRECTION ( 'NONE',  ( -1.000000000000000000, 0.000000000000000000, -2.245315044999999693E-12 ) ) ;
#7496=DIRECTION ( 'NONE',  ( -0.000000000000000000, 1.000000000000000000, 0.000000000000000000 ) ) ;
#7498=AXIS2_PLACEMENT_3D ( 'NONE', #11677, #16697, #412 ) ;
#7501=EDGE_LOOP ( 'NONE', ( #16046, #11848, #6566, #9929 ) ) ;
#7502=PLANE ( 'NONE',  #8198 ) ;
#7515=DIRECTION ( 'NONE',  ( -1.000000000000000000, 1.156482317317871725E-15, 0.000000000000000000 ) ) ;
#7516=DIRECTION ( 'NONE',  ( 0.000000000000000000, 0.000000000000000000, 1.000000000000000000 ) ) ;
#7518=ORIENTED_EDGE ( 'NONE', *, *, #5188, .F. ) ;
#7519=DIRECTION ( 'NONE',  ( 0.000000000000000000, 0.000000000000000000, 1.000000000000000000 ) ) ;
#7525=CARTESIAN_POINT ( 'NONE',  ( 13.13369214859999978, -51.00000000000000000, -136.0552959530000123 ) ) ;
#7529=CARTESIAN_POINT ( 'NONE',  ( 13.09808825513362862, 34.66051412330866555, -150.0552959529999839 ) ) ;
#7532=LINE ( 'NONE', #22416, #12841 ) ;
#7533=ORIENTED_EDGE ( 'NONE', *, *, #2855, .T. ) ;
#7535=ORIENTED_EDGE ( 'NONE', *, *, #4379, .T. ) ;
#7539=VECTOR ( 'NONE', #974, 1000.000000000000000 ) ;
#7540=VERTEX_POINT ( 'NONE', #23382 ) ;
#7545=VERTEX_POINT ( 'NONE', #23265 ) ;
#7550=ORIENTED_EDGE ( 'NONE', *, *, #784, .T. ) ;
#7554=DIRECTION ( 'NONE',  ( 1.000000000000000000, 0.000000000000000000, 0.000000000000000000 ) ) ;
#7555=CIRCLE ( 'NONE', #11726, 1.500000000000001332 ) ;
#7562=DIRECTION ( 'NONE',  ( 0.7633862853691523176, -0.6459422414661291079, 0.000000000000000000 ) ) ;
#7563=VERTEX_POINT ( 'NONE', #19691 ) ;
#7569=CARTESIAN_POINT ( 'NONE',  ( 4.500000000000000000, -3.500000000000000000, -140.0552959529999839 ) ) ;
#7573=ORIENTED_EDGE ( 'NONE', *, *, #8183, .F. ) ;
#7577=CARTESIAN_POINT ( 'NONE',  ( 13.95201674008764137, 21.48075934361423478, -150.0552959530000123 ) ) ;
#7582=CARTESIAN_POINT ( 'NONE',  ( -32.00000000000000000, -36.00000000000000000, -137.0552959530000123 ) ) ;
#7584=ORIENTED_EDGE ( 'NONE', *, *, #10838, .T. ) ;
#7592=ORIENTED_EDGE ( 'NONE', *, *, #20887, .T. ) ;
#7596=ORIENTED_EDGE ( 'NONE', *, *, #1533, .T. ) ;
#7600=CARTESIAN_POINT ( 'NONE',  ( 7.750000000000000000, 0.000000000000000000, -150.0552959529999839 ) ) ;
#7602=EDGE_CURVE ( 'NONE', #23428, #6865, #9661, .T. ) ;
#7604=LINE ( 'NONE', #18553, #13740 ) ;
#7605=DIRECTION ( 'NONE',  ( 0.000000000000000000, 0.000000000000000000, 1.000000000000000000 ) ) ;
#7607=CARTESIAN_POINT ( 'NONE',  ( 19.13369214879999802, 50.49999999980000354, -143.0552959529999839 ) ) ;
#7614=VECTOR ( 'NONE', #7143, 1000.000000000000000 ) ;
#7615=VECTOR ( 'NONE', #14963, 1000.000000000000000 ) ;
#7625=ADVANCED_FACE ( 'NONE', ( #20049 ), #9200, .F. ) ;
#7637=CARTESIAN_POINT ( 'NONE',  ( 32.50000000000000000, -39.92025131119999770, -149.5552959529999839 ) ) ;
#7640=EDGE_CURVE ( 'NONE', #3754, #10756, #7532, .T. ) ;
#7644=DIRECTION ( 'NONE',  ( 0.000000000000000000, 0.000000000000000000, 1.000000000000000000 ) ) ;
#7649=CARTESIAN_POINT ( 'NONE',  ( -32.50000000000000000, 0.000000000000000000, -150.0552959529999839 ) ) ;
#7651=FACE_OUTER_BOUND ( 'NONE', #19126, .T. ) ;
#7655=CARTESIAN_POINT ( 'NONE',  ( -13.86630785140000022, 50.50000000000000000, -136.0552959530000123 ) ) ;
#7656=VERTEX_POINT ( 'NONE', #7655 ) ;
#7662=AXIS2_PLACEMENT_3D ( 'NONE', #12873, #13221, #12995 ) ;
#7675=EDGE_CURVE ( 'NONE', #12039, #19224, #17239, .T. ) ;
#7677=EDGE_LOOP ( 'NONE', ( #19260, #13461, #8079, #17661 ) ) ;
#7678=VECTOR ( 'NONE', #4168, 1000.000000000000000 ) ;
#7690=CARTESIAN_POINT ( 'NONE',  ( -7.500000000000000000, 22.50000000000000000, -151.0552959529999839 ) ) ;
#7693=CARTESIAN_POINT ( 'NONE',  ( -12.50000000000000000, 48.50000000000000000, -150.5552959529999839 ) ) ;
#7700=EDGE_CURVE ( 'NONE', #954, #6667, #6693, .T. ) ;
#7717=CARTESIAN_POINT ( 'NONE',  ( 25.96278831570000278, 46.03148680980000051, -150.0552959529999839 ) ) ;
#7719=EDGE_LOOP ( 'NONE', ( #19392, #11053, #3580, #19640 ) ) ;
#7722=DIRECTION ( 'NONE',  ( 0.000000000000000000, 1.000000000000000000, 0.000000000000000000 ) ) ;
#7724=LINE ( 'NONE', #22251, #8688 ) ;
#7742=CARTESIAN_POINT ( 'NONE',  ( -1.500000000000000000, 44.50000000000000000, -150.0552959529999839 ) ) ;
#7743=CARTESIAN_POINT ( 'NONE',  ( -6.366307851450000221, 51.50000000000000000, -136.0552959530000123 ) ) ;
#7748=CARTESIAN_POINT ( 'NONE',  ( 31.32297112069999656, -40.18599471579999971, -150.0552959529999839 ) ) ;
#7754=FACE_BOUND ( 'NONE', #2355, .T. ) ;
#7756=LINE ( 'NONE', #20161, #3843 ) ;
#7758=EDGE_CURVE ( 'NONE', #16283, #6873, #16270, .T. ) ;
#7760=ORIENTED_EDGE ( 'NONE', *, *, #19619, .F. ) ;
#7764=CARTESIAN_POINT ( 'NONE',  ( 12.88080765318778731, 38.01462304345265153, -150.0552959529999839 ) ) ;
#7765=LINE ( 'NONE', #2546, #8248 ) ;
#7768=ADVANCED_FACE ( 'NONE', ( #3718 ), #18463, .F. ) ;
#7780=EDGE_CURVE ( 'NONE', #14361, #802, #508, .T. ) ;
#7781=AXIS2_PLACEMENT_3D ( 'NONE', #14035, #10338, #8545 ) ;
#7789=FACE_OUTER_BOUND ( 'NONE', #1327, .T. ) ;
#7798=ORIENTED_EDGE ( 'NONE', *, *, #7675, .F. ) ;
#7799=DIRECTION ( 'NONE',  ( 0.000000000000000000, 0.000000000000000000, -1.000000000000000000 ) ) ;
#7800=ORIENTED_EDGE ( 'NONE', *, *, #21402, .F. ) ;
#7802=PLANE ( 'NONE',  #20136 ) ;
#7806=DIRECTION ( 'NONE',  ( -1.000000000000000000, 0.000000000000000000, 0.000000000000000000 ) ) ;
#7809=CARTESIAN_POINT ( 'NONE',  ( 0.000000000000000000, 19.50000000000000000, -150.0552959529999839 ) ) ;
#7810=DIRECTION ( 'NONE',  ( 1.000000000000000000, 0.000000000000000000, 0.000000000000000000 ) ) ;
#7820=CARTESIAN_POINT ( 'NONE',  ( 1.133692148550000001, 50.50000000000000000, -142.8052959529999839 ) ) ;
#7823=DIRECTION ( 'NONE',  ( -0.000000000000000000, 1.000000000000000000, 0.000000000000000000 ) ) ;
#7828=CARTESIAN_POINT ( 'NONE',  ( -4.020716686303631882, 46.44926652720589999, -150.0552959530000123 ) ) ;
#7833=ADVANCED_FACE ( 'NONE', ( #5843 ), #21819, .F. ) ;
#7836=DIRECTION ( 'NONE',  ( -1.000000000000000000, 0.000000000000000000, 2.273736754430000208E-12 ) ) ;
#7838=ORIENTED_EDGE ( 'NONE', *, *, #1127, .T. ) ;
#7843=ORIENTED_EDGE ( 'NONE', *, *, #20945, .F. ) ;
#7846=DIRECTION ( 'NONE',  ( 0.000000000000000000, 0.000000000000000000, 1.000000000000000000 ) ) ;
#7851=FACE_OUTER_BOUND ( 'NONE', #21094, .T. ) ;
#7853=DIRECTION ( 'NONE',  ( 0.000000000000000000, 1.000000000000000000, 0.000000000000000000 ) ) ;
#7862=EDGE_CURVE ( 'NONE', #18719, #18280, #14662, .T. ) ;
#7867=ORIENTED_EDGE ( 'NONE', *, *, #8375, .T. ) ;
#7877=DIRECTION ( 'NONE',  ( -0.000000000000000000, 1.000000000000000000, 0.000000000000000000 ) ) ;
#7884=CARTESIAN_POINT ( 'NONE',  ( -12.50000000000000000, 22.50000000000000000, -151.0552959529999839 ) ) ;
#7890=VERTEX_POINT ( 'NONE', #18356 ) ;
#7904=ORIENTED_EDGE ( 'NONE', *, *, #14106, .F. ) ;
#7911=EDGE_CURVE ( 'NONE', #5505, #1160, #18812, .T. ) ;
#7924=DIRECTION ( 'NONE',  ( -2.259525899700000234E-12, 0.000000000000000000, 1.000000000000000000 ) ) ;
#7930=ADVANCED_FACE ( 'NONE', ( #13336 ), #2762, .T. ) ;
#7932=EDGE_CURVE ( 'NONE', #1705, #16883, #4767, .T. ) ;
#7935=ORIENTED_EDGE ( 'NONE', *, *, #15610, .T. ) ;
#7937=CARTESIAN_POINT ( 'NONE',  ( 19.13369214859999801, -51.00000000000000000, -136.0552959530000123 ) ) ;
#7942=ORIENTED_EDGE ( 'NONE', *, *, #2070, .F. ) ;
#7947=ORIENTED_EDGE ( 'NONE', *, *, #1439, .F. ) ;
#7949=VECTOR ( 'NONE', #15315, 1000.000000000000000 ) ;
#7952=VECTOR ( 'NONE', #19246, 1000.000000000000000 ) ;
#7953=LINE ( 'NONE', #20469, #7181 ) ;
#7956=ORIENTED_EDGE ( 'NONE', *, *, #17430, .F. ) ;
#7959=VERTEX_POINT ( 'NONE', #4412 ) ;
#7963=CARTESIAN_POINT ( 'NONE',  ( 2.656359840075251277, -1.100999472805462398, -150.0552959529999839 ) ) ;
#7971=VERTEX_POINT ( 'NONE', #13563 ) ;
#7979=DIRECTION ( 'NONE',  ( 1.000000000000000000, 0.000000000000000000, 0.000000000000000000 ) ) ;
#7983=ORIENTED_EDGE ( 'NONE', *, *, #11097, .F. ) ;
#7989=DIRECTION ( 'NONE',  ( 1.000000000000000000, 0.000000000000000000, 0.000000000000000000 ) ) ;
#7990=ORIENTED_EDGE ( 'NONE', *, *, #22956, .F. ) ;
#7992=EDGE_CURVE ( 'NONE', #16708, #20624, #20836, .T. ) ;
#7995=CARTESIAN_POINT ( 'NONE',  ( 19.27350934360000068, -50.38169314270000143, -149.5552959529999839 ) ) ;
#8009=LINE ( 'NONE', #20301, #1921 ) ;
#8012=AXIS2_PLACEMENT_3D ( 'NONE', #23506, #20294, #3524 ) ;
#8018=EDGE_CURVE ( 'NONE', #18803, #15247, #12070, .T. ) ;
#8020=CARTESIAN_POINT ( 'NONE',  ( 1.133692148550000001, -51.50000000000000000, -134.3952035990000127 ) ) ;
#8021=ORIENTED_EDGE ( 'NONE', *, *, #8899, .F. ) ;
#8022=CARTESIAN_POINT ( 'NONE',  ( 32.50000000000000000, -40.03620104880000241, -142.8052959529999839 ) ) ;
#8023=VECTOR ( 'NONE', #5362, 1000.000000000000000 ) ;
#8027=ORIENTED_EDGE ( 'NONE', *, *, #14919, .T. ) ;
#8035=ORIENTED_EDGE ( 'NONE', *, *, #14126, .F. ) ;
#8036=DIRECTION ( 'NONE',  ( 0.000000000000000000, -1.000000000000000000, 0.000000000000000000 ) ) ;
#8040=FACE_OUTER_BOUND ( 'NONE', #15731, .T. ) ;
#8041=EDGE_CURVE ( 'NONE', #20008, #6667, #12132, .T. ) ;
#8048=DIRECTION ( 'NONE',  ( 0.000000000000000000, 1.000000000000000000, 0.000000000000000000 ) ) ;
#8054=FACE_OUTER_BOUND ( 'NONE', #15965, .T. ) ;
#8058=VERTEX_POINT ( 'NONE', #19527 ) ;
#8060=EDGE_CURVE ( 'NONE', #5378, #19876, #4885, .T. ) ;
#8068=CARTESIAN_POINT ( 'NONE',  ( -1.000000000000000000, 20.50000000000000000, -150.5552959529999839 ) ) ;
#8069=EDGE_LOOP ( 'NONE', ( #12876, #6844, #1562, #4126, #16839, #1322, #4381 ) ) ;
#8075=ADVANCED_FACE ( 'NONE', ( #12607 ), #3111, .T. ) ;
#8079=ORIENTED_EDGE ( 'NONE', *, *, #22898, .T. ) ;
#8084=ORIENTED_EDGE ( 'NONE', *, *, #2105, .T. ) ;
#8087=DIRECTION ( 'NONE',  ( -1.000000000000000000, 0.000000000000000000, 0.000000000000000000 ) ) ;
#8091=DIRECTION ( 'NONE',  ( 0.000000000000000000, 1.000000000000000000, 0.000000000000000000 ) ) ;
#8094=DIRECTION ( 'NONE',  ( 1.000000000000000000, 0.000000000000000000, 0.000000000000000000 ) ) ;
#8110=CARTESIAN_POINT ( 'NONE',  ( -5.500000000000000000, 44.50000000000000000, -150.0552959529999839 ) ) ;
#8111=CARTESIAN_POINT ( 'NONE',  ( 4.084222279812038003, 13.38246373452152227, -150.0552959529999839 ) ) ;
#8113=CARTESIAN_POINT ( 'NONE',  ( -1.000000000000000000, 20.50000000000000000, -150.0552959529999839 ) ) ;
#8117=ORIENTED_EDGE ( 'NONE', *, *, #684, .F. ) ;
#8118=CARTESIAN_POINT ( 'NONE',  ( 8.750000000000000000, -38.23606797749999942, -150.5552959529999839 ) ) ;
#8124=ORIENTED_EDGE ( 'NONE', *, *, #4090, .F. ) ;
#8128=EDGE_CURVE ( 'NONE', #14773, #9439, #15715, .T. ) ;
#8130=CARTESIAN_POINT ( 'NONE',  ( -32.50000000000000000, -50.50000000000000000, -136.0552959530000123 ) ) ;
#8131=AXIS2_PLACEMENT_3D ( 'NONE', #8456, #6672, #21801 ) ;
#8138=ORIENTED_EDGE ( 'NONE', *, *, #21600, .T. ) ;
#8140=EDGE_LOOP ( 'NONE', ( #5791, #1782, #11006, #8613 ) ) ;
#8141=ORIENTED_EDGE ( 'NONE', *, *, #7780, .T. ) ;
#8144=VECTOR ( 'NONE', #4182, 1000.000000000000000 ) ;
#8148=EDGE_CURVE ( 'NONE', #21739, #11298, #8791, .T. ) ;
#8165=ORIENTED_EDGE ( 'NONE', *, *, #6685, .T. ) ;
#8167=LINE ( 'NONE', #19497, #15410 ) ;
#8168=ADVANCED_FACE ( 'NONE', ( #19882 ), #19992, .F. ) ;
#8169=ORIENTED_EDGE ( 'NONE', *, *, #150, .T. ) ;
#8172=ORIENTED_EDGE ( 'NONE', *, *, #11550, .T. ) ;
#8179=LINE ( 'NONE', #10077, #4163 ) ;
#8180=VECTOR ( 'NONE', #3081, 1000.000000000000000 ) ;
#8182=ORIENTED_EDGE ( 'NONE', *, *, #13587, .F. ) ;
#8183=EDGE_CURVE ( 'NONE', #2237, #3754, #1907, .T. ) ;
#8193=CARTESIAN_POINT ( 'NONE',  ( -31.00000000000000000, 1.000000000000000000, -150.5552959529999839 ) ) ;
#8198=AXIS2_PLACEMENT_3D ( 'NONE', #7393, #16664, #12979 ) ;
#8200=DIRECTION ( 'NONE',  ( -2.257242012349999735E-12, 0.000000000000000000, 1.000000000000000000 ) ) ;
#8202=CARTESIAN_POINT ( 'NONE',  ( -12.50000000000000000, 0.000000000000000000, -150.0552959529999839 ) ) ;
#8204=CARTESIAN_POINT ( 'NONE',  ( 26.50000000000000000, -20.50000000000000000, -150.0552959529999839 ) ) ;
#8205=CARTESIAN_POINT ( 'NONE',  ( -15.91979154561522947, -41.79923503140520324, -150.0552959529999839 ) ) ;
#8214=DIRECTION ( 'NONE',  ( 0.6459422414661292189, 0.7633862853691524286, 2.257144641400453113E-12 ) ) ;
#8218=CARTESIAN_POINT ( 'NONE',  ( 32.50000000000000000, 0.000000000000000000, -150.0552959529999839 ) ) ;
#8228=CARTESIAN_POINT ( 'NONE',  ( 0.5375835489636304754, 15.92407921618091393, -150.0552959529999839 ) ) ;
#8232=AXIS2_PLACEMENT_3D ( 'NONE', #8576, #21573, #12037 ) ;
#8234=VERTEX_POINT ( 'NONE', #12721 ) ;
#8238=ORIENTED_EDGE ( 'NONE', *, *, #5585, .T. ) ;
#8243=CARTESIAN_POINT ( 'NONE',  ( 19.13369214859999801, -51.50000000000000000, -136.0552959530000123 ) ) ;
#8244=ORIENTED_EDGE ( 'NONE', *, *, #17681, .F. ) ;
#8246=AXIS2_PLACEMENT_3D ( 'NONE', #5724, #12981, #5382 ) ;
#8248=VECTOR ( 'NONE', #11324, 1000.000000000000000 ) ;
#8261=PRESENTATION_STYLE_ASSIGNMENT (( #9928 ) ) ;
#8264=AXIS2_PLACEMENT_3D ( 'NONE', #7478, #11271, #18542 ) ;
#8271=DIRECTION ( 'NONE',  ( 2.257242012349999735E-12, 0.000000000000000000, -1.000000000000000000 ) ) ;
#8292=CARTESIAN_POINT ( 'NONE',  ( 24.28524365307784905, -23.42191803000494232, -150.0552959529999839 ) ) ;
#8293=ORIENTED_EDGE ( 'NONE', *, *, #16787, .F. ) ;
#8300=DIRECTION ( 'NONE',  ( 1.000000000000000000, 0.000000000000000000, 0.000000000000000000 ) ) ;
#8305=AXIS2_PLACEMENT_3D ( 'NONE', #3119, #10351, #17626 ) ;
#8312=DIRECTION ( 'NONE',  ( -1.000000000000000000, 0.000000000000000000, 0.000000000000000000 ) ) ;
#8313=VECTOR ( 'NONE', #1241, 1000.000000000000000 ) ;
#8324=CARTESIAN_POINT ( 'NONE',  ( -13.69030790613426873, -42.24283201952169975, -150.0552959529999839 ) ) ;
#8333=FACE_OUTER_BOUND ( 'NONE', #16591, .T. ) ;
#8336=ORIENTED_EDGE ( 'NONE', *, *, #15129, .T. ) ;
#8338=FACE_OUTER_BOUND ( 'NONE', #22776, .T. ) ;
#8339=FACE_OUTER_BOUND ( 'NONE', #8502, .T. ) ;
#8341=AXIS2_PLACEMENT_3D ( 'NONE', #4020, #9464, #13280 ) ;
#8349=EDGE_LOOP ( 'NONE', ( #18634, #20792, #19675, #6876 ) ) ;
#8351=EDGE_CURVE ( 'NONE', #213, #4867, #2838, .T. ) ;
#8352=CARTESIAN_POINT ( 'NONE',  ( 23.00000000000000000, 19.50000000000000000, -151.0552959529999839 ) ) ;
#8358=CARTESIAN_POINT ( 'NONE',  ( 4.798892695402127373, -33.70134726954550075, -150.0552959529999555 ) ) ;
#8359=ORIENTED_EDGE ( 'NONE', *, *, #4204, .T. ) ;
#8370=ORIENTED_EDGE ( 'NONE', *, *, #23141, .F. ) ;
#8375=EDGE_CURVE ( 'NONE', #11748, #21536, #18674, .T. ) ;
#8378=CARTESIAN_POINT ( 'NONE',  ( -18.00000000000001066, -42.60730091830129140, -150.0552959529999839 ) ) ;
#8379=AXIS2_PLACEMENT_3D ( 'NONE', #17000, #7605, #5593 ) ;
#8383=B_SPLINE_CURVE_WITH_KNOTS ( 'NONE', 3,
 ( #12347, #9250, #3320, #14267, #5218, #20560, #4369, #11494, #693, #16748 ),
 .UNSPECIFIED., .F., .F.,
 ( 4, 2, 2, 2, 4 ),
 ( 0.000000000000000000, 0.2499999999999999445, 0.4999999999999998890, 0.7499999999999998890, 1.000000000000000000 ),
 .UNSPECIFIED. ) ;
#8384=LINE ( 'NONE', #13861, #22638 ) ;
#8410=CARTESIAN_POINT ( 'NONE',  ( 22.50000000000000000, 39.50000000000000000, -150.0552959529999839 ) ) ;
#8418=CARTESIAN_POINT ( 'NONE',  ( 22.50000000000000000, 39.50000000000000000, -151.0552959529999839 ) ) ;
#8421=DIRECTION ( 'NONE',  ( 0.000000000000000000, -1.000000000000000000, 2.257144641399999941E-12 ) ) ;
#8422=EDGE_LOOP ( 'NONE', ( #16027, #2102, #17525, #14856 ) ) ;
#8426=ORIENTED_EDGE ( 'NONE', *, *, #10231, .F. ) ;
#8430=COLOUR_RGB ( '', 0.40784314, 0.44705882, 0.49803922) ;
#8431=DIRECTION ( 'NONE',  ( 0.7633862853691523176, 0.6459422414661291079, 0.000000000000000000 ) ) ;
#8432=CIRCLE ( 'NONE', #13754, 7.499999999999999112 ) ;
#8436=CARTESIAN_POINT ( 'NONE',  ( 23.50000000000000000, -20.50000000000000000, -135.0552959530000123 ) ) ;
#8445=DIRECTION ( 'NONE',  ( 2.257144641399999941E-12, 0.000000000000000000, 1.000000000000000000 ) ) ;
#8450=CARTESIAN_POINT ( 'NONE',  ( 32.00000000000000000, -40.03620104880000241, -136.0552959530000123 ) ) ;
#8453=CARTESIAN_POINT ( 'NONE',  ( -15.50000000000000000, 47.50000000000000000, -150.0552959529999839 ) ) ;
#8456=CARTESIAN_POINT ( 'NONE',  ( -31.75000000000000000, 19.50000000000000000, -151.0552959529999839 ) ) ;
#8457=ORIENTED_EDGE ( 'NONE', *, *, #12811, .T. ) ;
#8460=CARTESIAN_POINT ( 'NONE',  ( 3.038109793998242214, -3.109613115927613247, -150.0552959530000123 ) ) ;
#8468=DIRECTION ( 'NONE',  ( 0.7071067811865476838, -0.7071067811865475727, 0.000000000000000000 ) ) ;
#8474=CARTESIAN_POINT ( 'NONE',  ( -5.500000000000000000, 44.50000000000000000, -150.5552959529999839 ) ) ;
#8476=CARTESIAN_POINT ( 'NONE',  ( 19.27350934360000068, 50.38169314270000143, -150.0552959529999839 ) ) ;
#8492=CARTESIAN_POINT ( 'NONE',  ( -17.92191803000495298, -42.21475634692217938, -150.0552959530000123 ) ) ;
#8497=DIRECTION ( 'NONE',  ( 1.000000000000000000, 0.000000000000000000, 0.000000000000000000 ) ) ;
#8498=PLANE ( 'NONE',  #15056 ) ;
#8500=CARTESIAN_POINT ( 'NONE',  ( 32.50000000000000000, -39.92025131100000124, -149.5552959529999839 ) ) ;
#8502=EDGE_LOOP ( 'NONE', ( #5598, #19768, #20901, #105 ) ) ;
#8506=DIRECTION ( 'NONE',  ( -1.457881434619999915E-12, 1.723066134219999902E-12, 1.000000000000000000 ) ) ;
#8509=EDGE_CURVE ( 'NONE', #21875, #18822, #21168, .T. ) ;
#8510=VERTEX_POINT ( 'NONE', #8527 ) ;
#8520=CARTESIAN_POINT ( 'NONE',  ( 25.50006728695417024, 36.10251055749550630, -150.0552959529999839 ) ) ;
#8521=ORIENTED_EDGE ( 'NONE', *, *, #1533, .F. ) ;
#8525=CARTESIAN_POINT ( 'NONE',  ( 31.00000000000000000, -0.7500000000009999779, -149.5552959529999839 ) ) ;
#8527=CARTESIAN_POINT ( 'NONE',  ( -31.00000000000000000, -36.00000000000000000, -150.0552959529999839 ) ) ;
#8528=DIRECTION ( 'NONE',  ( -1.000000000000000000, 0.000000000000000000, 0.000000000000000000 ) ) ;
#8538=ORIENTED_EDGE ( 'NONE', *, *, #14270, .T. ) ;
#8539=LINE ( 'NONE', #9853, #9083 ) ;
#8540=FACE_OUTER_BOUND ( 'NONE', #4507, .T. ) ;
#8544=CARTESIAN_POINT ( 'NONE',  ( 8.750000000000000000, -40.23606797749999942, -151.0552959529999839 ) ) ;
#8545=DIRECTION ( 'NONE',  ( 0.000000000000000000, 1.000000000000000000, 0.000000000000000000 ) ) ;
#8550=CARTESIAN_POINT ( 'NONE',  ( -31.99999999949999818, 19.50000000000000000, -137.0552959530000123 ) ) ;
#8553=DIRECTION ( 'NONE',  ( 2.252420472359999842E-12, 0.000000000000000000, -1.000000000000000000 ) ) ;
#8569=VECTOR ( 'NONE', #10423, 1000.000000000000000 ) ;
#8576=CARTESIAN_POINT ( 'NONE',  ( 3.552713678799999608E-15, 50.00000000000000000, -149.5552959529999839 ) ) ;
#8578=ORIENTED_EDGE ( 'NONE', *, *, #21161, .F. ) ;
#8584=EDGE_LOOP ( 'NONE', ( #21252, #18679, #13870, #3306 ) ) ;
#8587=EDGE_LOOP ( 'NONE', ( #11016, #3372, #19710, #5986 ) ) ;
#8595=DIRECTION ( 'NONE',  ( -1.000000000000000000, 0.000000000000000000, 0.000000000000000000 ) ) ;
#8601=CARTESIAN_POINT ( 'NONE',  ( 23.50000000000000000, -20.50000000000000000, -137.0552959530000123 ) ) ;
#8602=VECTOR ( 'NONE', #5807, 1000.000000000000000 ) ;
#8604=CARTESIAN_POINT ( 'NONE',  ( 5.961890206001605463, -3.890386884071861395, -150.0552959530000408 ) ) ;
#8606=ORIENTED_EDGE ( 'NONE', *, *, #14919, .F. ) ;
#8607=LINE ( 'NONE', #15881, #10556 ) ;
#8608=EDGE_CURVE ( 'NONE', #7053, #2155, #22786, .T. ) ;
#8610=ORIENTED_EDGE ( 'NONE', *, *, #22090, .T. ) ;
#8613=ORIENTED_EDGE ( 'NONE', *, *, #21831, .F. ) ;
#8619=AXIS2_PLACEMENT_3D ( 'NONE', #4328, #13123, #5756 ) ;
#8623=ORIENTED_EDGE ( 'NONE', *, *, #9064, .T. ) ;
#8625=EDGE_CURVE ( 'NONE', #16505, #8645, #13974, .T. ) ;
#8626=PLANE ( 'NONE',  #15930 ) ;
#8630=EDGE_CURVE ( 'NONE', #11744, #19192, #1734, .T. ) ;
#8635=FACE_OUTER_BOUND ( 'NONE', #23193, .T. ) ;
#8645=VERTEX_POINT ( 'NONE', #23375 ) ;
#8648=ORIENTED_EDGE ( 'NONE', *, *, #22457, .F. ) ;
#8662=CARTESIAN_POINT ( 'NONE',  ( -7.500000000000000000, 0.000000000000000000, -150.0552959529999839 ) ) ;
#8673=AXIS2_PLACEMENT_3D ( 'NONE', #5715, #7496, #10582 ) ;
#8674=CARTESIAN_POINT ( 'NONE',  ( -3.500000000000000000, 40.00000000000000000, -150.0552959529999839 ) ) ;
#8677=DIRECTION ( 'NONE',  ( 0.000000000000000000, 2.257144641399999941E-12, 1.000000000000000000 ) ) ;
#8681=ORIENTED_EDGE ( 'NONE', *, *, #104, .T. ) ;
#8688=VECTOR ( 'NONE', #5943, 1000.000000000000000 ) ;
#8691=VECTOR ( 'NONE', #20520, 1000.000000000000000 ) ;
#8692=CARTESIAN_POINT ( 'NONE',  ( 8.750000000000000000, -42.23606797749999942, -151.0552959529999839 ) ) ;
#8695=CARTESIAN_POINT ( 'NONE',  ( 1.544832289344039822, 26.15117705467530840, -150.0552959529999839 ) ) ;
#8699=CYLINDRICAL_SURFACE ( 'NONE', #1602, 2.999999999999999112 ) ;
#8702=VECTOR ( 'NONE', #18923, 1000.000000000000000 ) ;
#8703=ORIENTED_EDGE ( 'NONE', *, *, #13616, .F. ) ;
#8708=VECTOR ( 'NONE', #8036, 1000.000000000000000 ) ;
#8711=CARTESIAN_POINT ( 'NONE',  ( 4.750000000000000000, -38.23606797749999942, -151.0552959529999839 ) ) ;
#8713=DIRECTION ( 'NONE',  ( 0.000000000000000000, -1.000000000000000000, 0.000000000000000000 ) ) ;
#8729=B_SPLINE_CURVE_WITH_KNOTS ( 'NONE', 3,
 ( #641, #4438, #6459, #11560, #8111, #763, #6107, #9891, #17169, #22643, #8228, #2897, #6336, #22891, #10127, #20989, #6223, #15501 ),
 .UNSPECIFIED., .F., .F.,
 ( 4, 2, 2, 2, 2, 2, 2, 2, 4 ),
 ( 0.000000000000000000, 0.1249999999999999167, 0.2499999999999998335, 0.3749999999999998335, 0.4999999999999998890, 0.6249999999999998890, 0.7499999999999998890, 0.8750000000000000000, 1.000000000000000000 ),
 .UNSPECIFIED. ) ;
#8737=LINE ( 'NONE', #9844, #15645 ) ;
#8738=CARTESIAN_POINT ( 'NONE',  ( -32.50000000000000000, 51.00000000000000000, -137.0552959530000123 ) ) ;
#8741=CARTESIAN_POINT ( 'NONE',  ( 25.31684607440000079, 45.26810052420000119, -136.0552959530000123 ) ) ;
#8744=PLANE ( 'NONE',  #11798 ) ;
#8747=DIRECTION ( 'NONE',  ( -3.781283367744424970E-15, 0.000000000000000000, 1.000000000000000000 ) ) ;
#8748=VERTEX_POINT ( 'NONE', #15998 ) ;
#8755=ADVANCED_FACE ( 'NONE', ( #13007 ), #14800, .F. ) ;
#8759=AXIS2_PLACEMENT_3D ( 'NONE', #9228, #16495, #18507 ) ;
#8760=CARTESIAN_POINT ( 'NONE',  ( -32.50000000000000000, 19.50000000000000000, -143.3052959529999839 ) ) ;
#8769=ORIENTED_EDGE ( 'NONE', *, *, #9840, .T. ) ;
#8781=LINE ( 'NONE', #7129, #12795 ) ;
#8783=ADVANCED_FACE ( 'NONE', ( #284 ), #16692, .T. ) ;
#8785=CARTESIAN_POINT ( 'NONE',  ( -32.50000000000000000, 21.50000000000000000, -150.0552959529999839 ) ) ;
#8786=EDGE_LOOP ( 'NONE', ( #8921, #16638 ) ) ;
#8791=LINE ( 'NONE', #16071, #21275 ) ;
#8794=( GEOMETRIC_REPRESENTATION_CONTEXT ( 3 ) GLOBAL_UNCERTAINTY_ASSIGNED_CONTEXT ( ( #1859 ) ) GLOBAL_UNIT_ASSIGNED_CONTEXT ( ( #20777, #4244, #20904 ) ) REPRESENTATION_CONTEXT ( 'NONE', 'WORKASPACE' ) );
#8815=LINE ( 'NONE', #19784, #14793 ) ;
#8827=EDGE_CURVE ( 'NONE', #10244, #12707, #16356, .T. ) ;
#8833=B_SPLINE_CURVE_WITH_KNOTS ( 'NONE', 3,
 ( #6484, #5160, #21367, #1147, #10496, #21478, #4817, #12061, #13743, #1496, #12406, #19331, #21008, #5057, #12299, #8492, #8378, #19683 ),
 .UNSPECIFIED., .F., .F.,
 ( 4, 2, 2, 2, 2, 2, 2, 2, 4 ),
 ( 0.000000000000000000, 0.1249999999999997224, 0.2499999999999994449, 0.3749999999999991673, 0.4999999999999988898, 0.6249999999999991118, 0.7499999999999994449, 0.8749999999999996669, 1.000000000000000000 ),
 .UNSPECIFIED. ) ;
#8835=DIRECTION ( 'NONE',  ( 0.000000000000000000, 0.000000000000000000, 1.000000000000000000 ) ) ;
#8839=CARTESIAN_POINT ( 'NONE',  ( 19.71905350739518070, 19.57650987475782500, -150.0552959530000123 ) ) ;
#8841=DIRECTION ( 'NONE',  ( 0.000000000000000000, -1.000000000000000000, 0.000000000000000000 ) ) ;
#8845=CARTESIAN_POINT ( 'NONE',  ( 8.750000000000000000, -38.23606797749999942, -150.0552959529999839 ) ) ;
#8848=LINE ( 'NONE', #5166, #14710 ) ;
#8861=FACE_OUTER_BOUND ( 'NONE', #6181, .T. ) ;
#8871=DIRECTION ( 'NONE',  ( 0.000000000000000000, -2.956752937091289955E-12, -1.000000000000000000 ) ) ;
#8873=ORIENTED_EDGE ( 'NONE', *, *, #12168, .F. ) ;
#8874=CARTESIAN_POINT ( 'NONE',  ( 20.50000000000000000, -20.50000000000000000, -137.0552959530000123 ) ) ;
#8882=VECTOR ( 'NONE', #7298, 1000.000000000000000 ) ;
#8884=CARTESIAN_POINT ( 'NONE',  ( 32.14594224169999848, -40.79958733389999992, -143.0552959529999839 ) ) ;
#8890=ORIENTED_EDGE ( 'NONE', *, *, #14483, .T. ) ;
#8898=DIRECTION ( 'NONE',  ( 0.000000000000000000, -1.000000000000000000, 2.257144641399999941E-12 ) ) ;
#8899=EDGE_CURVE ( 'NONE', #12137, #11748, #21765, .T. ) ;
#8905=FACE_OUTER_BOUND ( 'NONE', #3492, .T. ) ;
#8908=DIRECTION ( 'NONE',  ( -1.000000000000000000, 0.000000000000000000, 0.000000000000000000 ) ) ;
#8909=CARTESIAN_POINT ( 'NONE',  ( -32.50000000000000000, 10.25000000000000000, -137.0552959530000123 ) ) ;
#8921=ORIENTED_EDGE ( 'NONE', *, *, #15465, .T. ) ;
#8923=ORIENTED_EDGE ( 'NONE', *, *, #7992, .T. ) ;
#8924=CARTESIAN_POINT ( 'NONE',  ( 25.31684607480000082, -45.26810052400000473, -150.0552959529999839 ) ) ;
#8949=VECTOR ( 'NONE', #9261, 1000.000000000000000 ) ;
#8951=ORIENTED_EDGE ( 'NONE', *, *, #14495, .T. ) ;
#8953=B_SPLINE_CURVE_WITH_KNOTS ( 'NONE', 3,
 ( #10667, #21644, #14143, #12337, #10780, #17826, #10545, #1776, #23302, #8997 ),
 .UNSPECIFIED., .F., .F.,
 ( 4, 2, 2, 2, 4 ),
 ( 0.000000000000000000, 0.2500000000000000000, 0.5000000000000000000, 0.7500000000000000000, 1.000000000000000000 ),
 .UNSPECIFIED. ) ;
#8957=ADVANCED_FACE ( 'NONE', ( #12810 ), #14372, .F. ) ;
#8962=LINE ( 'NONE', #14806, #7026 ) ;
#8975=CARTESIAN_POINT ( 'NONE',  ( 31.32297112069999656, 40.18599471579999971, -149.5552959529999839 ) ) ;
#8982=AXIS2_PLACEMENT_3D ( 'NONE', #9479, #2693, #4030 ) ;
#8987=LINE ( 'NONE', #4004, #4599 ) ;
#8990=PLANE ( 'NONE',  #992 ) ;
#8993=CARTESIAN_POINT ( 'NONE',  ( -32.50000000000000000, -43.00000000050000182, -137.0552959530000123 ) ) ;
#8997=CARTESIAN_POINT ( 'NONE',  ( -5.500000000000000000, 44.50000000000000000, -150.0552959529999839 ) ) ;
#9003=VERTEX_POINT ( 'NONE', #23182 ) ;
#9007=VERTEX_POINT ( 'NONE', #6875 ) ;
#9008=EDGE_CURVE ( 'NONE', #13555, #15811, #8953, .T. ) ;
#9015=CARTESIAN_POINT ( 'NONE',  ( 32.00000000000000000, 32.96379895120000469, -137.0552959530000123 ) ) ;
#9025=VECTOR ( 'NONE', #15473, 1000.000000000000227 ) ;
#9027=CARTESIAN_POINT ( 'NONE',  ( -10.00000000000000000, 48.50000000000000000, -150.0552959529999839 ) ) ;
#9037=DIRECTION ( 'NONE',  ( -0.7633862853691523176, -0.6459422414661291079, 0.000000000000000000 ) ) ;
#9043=ORIENTED_EDGE ( 'NONE', *, *, #684, .T. ) ;
#9047=VECTOR ( 'NONE', #12940, 1000.000000000000000 ) ;
#9048=ADVANCED_FACE ( 'NONE', ( #22216 ), #18412, .T. ) ;
#9049=ORIENTED_EDGE ( 'NONE', *, *, #22956, .T. ) ;
#9052=CARTESIAN_POINT ( 'NONE',  ( -12.50000000000000000, 48.50000000000000000, -150.0552959529999839 ) ) ;
#9056=EDGE_CURVE ( 'NONE', #9183, #22593, #20548, .T. ) ;
#9062=DIRECTION ( 'NONE',  ( 0.000000000000000000, -2.231104189749999978E-12, 1.000000000000000000 ) ) ;
#9064=EDGE_CURVE ( 'NONE', #20852, #7545, #16628, .T. ) ;
#9067=LINE ( 'NONE', #7525, #4805 ) ;
#9070=CARTESIAN_POINT ( 'NONE',  ( 13.98502865237644777, 39.11890206003842252, -150.0552959529999839 ) ) ;
#9072=LINE ( 'NONE', #1626, #12046 ) ;
#9074=AXIS2_PLACEMENT_3D ( 'NONE', #20984, #759, #7989 ) ;
#9076=EDGE_CURVE ( 'NONE', #21875, #1062, #3904, .T. ) ;
#9083=VECTOR ( 'NONE', #8431, 1000.000000000000227 ) ;
#9100=ORIENTED_EDGE ( 'NONE', *, *, #3334, .F. ) ;
#9105=VECTOR ( 'NONE', #4248, 1000.000000000000000 ) ;
#9107=CYLINDRICAL_SURFACE ( 'NONE', #9459, 2.000000000000000000 ) ;
#9109=LINE ( 'NONE', #2110, #430 ) ;
#9111=CARTESIAN_POINT ( 'NONE',  ( 7.976419552961967696, -48.60121046038479875, -150.0552959529999839 ) ) ;
#9115=EDGE_LOOP ( 'NONE', ( #18892, #19916, #14462, #22836 ) ) ;
#9121=AXIS2_PLACEMENT_3D ( 'NONE', #15320, #13285, #18654 ) ;
#9122=EDGE_CURVE ( 'NONE', #3037, #8645, #11708, .T. ) ;
#9123=VERTEX_POINT ( 'NONE', #4359 ) ;
#9125=EDGE_CURVE ( 'NONE', #232, #11298, #4713, .T. ) ;
#9132=LINE ( 'NONE', #14624, #15166 ) ;
#9133=EDGE_CURVE ( 'NONE', #3527, #751, #17321, .T. ) ;
#9139=LINE ( 'NONE', #20105, #22400 ) ;
#9157=VECTOR ( 'NONE', #21616, 1000.000000000000000 ) ;
#9159=EDGE_LOOP ( 'NONE', ( #22928, #15291, #4634, #20133 ) ) ;
#9162=ORIENTED_EDGE ( 'NONE', *, *, #15268, .F. ) ;
#9173=VECTOR ( 'NONE', #7836, 1000.000000000000000 ) ;
#9174=DIRECTION ( 'NONE',  ( 0.000000000000000000, -1.000000000000000000, 1.723073263340000007E-12 ) ) ;
#9179=DIRECTION ( 'NONE',  ( -0.7633862853691522066, 0.6459422414661292189, -1.795096815436260566E-28 ) ) ;
#9180=DIRECTION ( 'NONE',  ( 1.000000000000000000, 0.000000000000000000, 0.000000000000000000 ) ) ;
#9183=VERTEX_POINT ( 'NONE', #17570 ) ;
#9185=AXIS2_PLACEMENT_3D ( 'NONE', #4739, #707, #8421 ) ;
#9190=EDGE_CURVE ( 'NONE', #11748, #15992, #22929, .T. ) ;
#9191=LINE ( 'NONE', #16464, #13639 ) ;
#9192=CARTESIAN_POINT ( 'NONE',  ( -3.500000000000000000, 44.50000000000000000, -150.0552959529999839 ) ) ;
#9195=DIRECTION ( 'NONE',  ( -0.6459422414661291079, 0.7633862853691523176, -2.245315045000450442E-12 ) ) ;
#9197=CARTESIAN_POINT ( 'NONE',  ( -2.500000000000000000, 34.00000000000000000, -151.0552959529999839 ) ) ;
#9200=PLANE ( 'NONE',  #15496 ) ;
#9209=LINE ( 'NONE', #75, #6138 ) ;
#9224=CARTESIAN_POINT ( 'NONE',  ( -13.86630785140000022, -51.50000000000000000, -136.0552959530000123 ) ) ;
#9228=CARTESIAN_POINT ( 'NONE',  ( 18.95053822279999878, 50.00000000000000000, -149.5552959529999839 ) ) ;
#9230=DIRECTION ( 'NONE',  ( 3.552713678800000397E-15, 7.105427357600000794E-15, 1.000000000000000000 ) ) ;
#9234=ORIENTED_EDGE ( 'NONE', *, *, #2250, .F. ) ;
#9237=ORIENTED_EDGE ( 'NONE', *, *, #18111, .F. ) ;
#9250=CARTESIAN_POINT ( 'NONE',  ( -3.234790887188633945, 46.50000000000002132, -150.0552959530000408 ) ) ;
#9254=FACE_OUTER_BOUND ( 'NONE', #11617, .T. ) ;
#9256=EDGE_CURVE ( 'NONE', #11512, #20386, #20610, .T. ) ;
#9261=DIRECTION ( 'NONE',  ( -1.000000000000000000, 0.000000000000000000, -2.273736754430000208E-12 ) ) ;
#9265=CARTESIAN_POINT ( 'NONE',  ( 32.50000000000000000, -40.03620104880000241, -142.8052959529999839 ) ) ;
#9272=ORIENTED_EDGE ( 'NONE', *, *, #21429, .F. ) ;
#9275=LINE ( 'NONE', #18103, #16649 ) ;
#9278=DIRECTION ( 'NONE',  ( 1.000000000000000000, 0.000000000000000000, 0.000000000000000000 ) ) ;
#9284=CARTESIAN_POINT ( 'NONE',  ( -1.000000000000000000, 20.50000000000000000, -151.0552959529999839 ) ) ;
#9291=LINE ( 'NONE', #22395, #1989 ) ;
#9294=CARTESIAN_POINT ( 'NONE',  ( -13.50000000000000000, -43.00000000000000000, -140.0552959529999839 ) ) ;
#9297=FACE_OUTER_BOUND ( 'NONE', #6991, .T. ) ;
#9302=EDGE_CURVE ( 'NONE', #11634, #8234, #12540, .T. ) ;
#9321=FACE_OUTER_BOUND ( 'NONE', #6016, .T. ) ;
#9324=ADVANCED_FACE ( 'NONE', ( #10752, #4954 ), #12423, .F. ) ;
#9328=VECTOR ( 'NONE', #13301, 1000.000000000000000 ) ;
#9338=CARTESIAN_POINT ( 'NONE',  ( 18.95053822279999878, -50.50000000000000000, -150.0552959529999839 ) ) ;
#9341=CARTESIAN_POINT ( 'NONE',  ( -12.37864083493721878, -44.51085694111268509, -150.0552959529999839 ) ) ;
#9344=ORIENTED_EDGE ( 'NONE', *, *, #6327, .F. ) ;
#9352=CARTESIAN_POINT ( 'NONE',  ( -32.50000000000000000, 50.00000000000000000, -151.0552959529999839 ) ) ;
#9354=ADVANCED_FACE ( 'NONE', ( #74 ), #3171, .F. ) ;
#9357=DIRECTION ( 'NONE',  ( 0.000000000000000000, -1.000000000000000000, 0.000000000000000000 ) ) ;
#9360=DIRECTION ( 'NONE',  ( -1.000000000000000000, 0.000000000000000000, 0.000000000000000000 ) ) ;
#9361=AXIS2_PLACEMENT_3D ( 'NONE', #11796, #22412, #18952 ) ;
#9372=DIRECTION ( 'NONE',  ( 0.000000000000000000, -1.000000000000000000, 0.000000000000000000 ) ) ;
#9374=ORIENTED_EDGE ( 'NONE', *, *, #23081, .T. ) ;
#9376=LINE ( 'NONE', #3820, #18266 ) ;
#9378=DIRECTION ( 'NONE',  ( 0.000000000000000000, 0.000000000000000000, 1.000000000000000000 ) ) ;
#9383=CARTESIAN_POINT ( 'NONE',  ( -32.50000000000000000, -36.00000000000000000, -143.3052959529999839 ) ) ;
#9387=ORIENTED_EDGE ( 'NONE', *, *, #1797, .T. ) ;
#9392=CARTESIAN_POINT ( 'NONE',  ( -32.50000000000000000, -14.25000000000000000, -150.0552959529999839 ) ) ;
#9395=CARTESIAN_POINT ( 'NONE',  ( 32.00000000000000000, -39.80430157320000006, -149.5552959529999839 ) ) ;
#9401=AXIS2_PLACEMENT_3D ( 'NONE', #14041, #7257, #5358 ) ;
#9410=VERTEX_POINT ( 'NONE', #8453 ) ;
#9412=VECTOR ( 'NONE', #21804, 1000.000000000000000 ) ;
#9419=LINE ( 'NONE', #1854, #18888 ) ;
#9423=ORIENTED_EDGE ( 'NONE', *, *, #2549, .F. ) ;
#9431=AXIS2_PLACEMENT_3D ( 'NONE', #11361, #13275, #7799 ) ;
#9436=DIRECTION ( 'NONE',  ( 0.000000000000000000, 2.259525899700000234E-12, 1.000000000000000000 ) ) ;
#9437=EDGE_CURVE ( 'NONE', #11594, #467, #12368, .T. ) ;
#9439=VERTEX_POINT ( 'NONE', #15721 ) ;
#9445=LINE ( 'NONE', #16724, #20783 ) ;
#9447=AXIS2_PLACEMENT_3D ( 'NONE', #21683, #11171, #18217 ) ;
#9448=VECTOR ( 'NONE', #17281, 1000.000000000000000 ) ;
#9450=VERTEX_POINT ( 'NONE', #14175 ) ;
#9453=ORIENTED_EDGE ( 'NONE', *, *, #7207, .T. ) ;
#9459=AXIS2_PLACEMENT_3D ( 'NONE', #3417, #12685, #19952 ) ;
#9463=AXIS2_PLACEMENT_3D ( 'NONE', #13839, #6224, #1247 ) ;
#9464=DIRECTION ( 'NONE',  ( 0.000000000000000000, -1.000000000000000000, 0.000000000000000000 ) ) ;
#9473=DIRECTION ( 'NONE',  ( -1.000000000000000000, 0.000000000000000000, 2.257144641399999941E-12 ) ) ;
#9475=CARTESIAN_POINT ( 'NONE',  ( 14.00000000000000000, 20.50000000000000000, -150.5552959529999839 ) ) ;
#9479=CARTESIAN_POINT ( 'NONE',  ( 13.13369214859999978, -51.50000000000000000, -137.0552959530000123 ) ) ;
#9485=DIRECTION ( 'NONE',  ( 1.000000000000000000, 0.000000000000000000, 0.000000000000000000 ) ) ;
#9492=EDGE_LOOP ( 'NONE', ( #16476, #6769, #8336, #3357 ) ) ;
#9494=DIRECTION ( 'NONE',  ( 0.000000000000000000, 0.000000000000000000, -1.000000000000000000 ) ) ;
#9499=CARTESIAN_POINT ( 'NONE',  ( 32.14594224169999848, -40.79958733389999992, -143.0552959529999839 ) ) ;
#9500=ORIENTED_EDGE ( 'NONE', *, *, #18197, .F. ) ;
#9502=CARTESIAN_POINT ( 'NONE',  ( -32.50000000000000000, 10.25000000000000000, -137.0552959530000123 ) ) ;
#9509=AXIS2_PLACEMENT_3D ( 'NONE', #15102, #12842, #715 ) ;
#9512=EDGE_LOOP ( 'NONE', ( #21216, #17283, #14104, #18298 ) ) ;
#9513=EDGE_CURVE ( 'NONE', #5292, #6470, #15605, .T. ) ;
#9517=PLANE ( 'NONE',  #16608 ) ;
#9521=LINE ( 'NONE', #8202, #5532 ) ;
#9522=EDGE_CURVE ( 'NONE', #2624, #2028, #23097, .T. ) ;
#9532=EDGE_CURVE ( 'NONE', #2149, #4983, #12140, .T. ) ;
#9533=PLANE ( 'NONE',  #4262 ) ;
#9535=LINE ( 'NONE', #15016, #11155 ) ;
#9543=DIRECTION ( 'NONE',  ( -0.6459422414661291079, 0.7633862853691523176, -2.245315045000450442E-12 ) ) ;
#9549=CARTESIAN_POINT ( 'NONE',  ( 1.133692148550000001, 50.50000000000000000, -137.0552959530000123 ) ) ;
#9553=ADVANCED_FACE ( 'NONE', ( #19288 ), #10234, .F. ) ;
#9558=DIRECTION ( 'NONE',  ( 0.000000000000000000, -2.252420471819999940E-12, 1.000000000000000000 ) ) ;
#9559=CIRCLE ( 'NONE', #6157, 1.500000000000001332 ) ;
#9562=CIRCLE ( 'NONE', #12613, 2.000000000000000000 ) ;
#9566=VERTEX_POINT ( 'NONE', #19533 ) ;
#9573=ADVANCED_FACE ( 'NONE', ( #3227 ), #7267, .T. ) ;
#9578=CARTESIAN_POINT ( 'NONE',  ( 13.13369214859999978, -51.50000000000000000, -137.0552959530000123 ) ) ;
#9579=ORIENTED_EDGE ( 'NONE', *, *, #22249, .T. ) ;
#9585=EDGE_LOOP ( 'NONE', ( #19606, #12689, #10995, #10903 ) ) ;
#9586=FACE_OUTER_BOUND ( 'NONE', #5827, .T. ) ;
#9588=CARTESIAN_POINT ( 'NONE',  ( 8.446000075252877437, 27.76013181716563594, -150.0552959529999555 ) ) ;
#9591=DIRECTION ( 'NONE',  ( 1.000000000000000000, 0.000000000000000000, 0.000000000000000000 ) ) ;
#9594=CARTESIAN_POINT ( 'NONE',  ( 32.50000000000000000, 39.80430157320000006, -149.8052959529999839 ) ) ;
#9607=VERTEX_POINT ( 'NONE', #16540 ) ;
#9609=ORIENTED_EDGE ( 'NONE', *, *, #21131, .F. ) ;
#9617=DIRECTION ( 'NONE',  ( 0.000000000000000000, -1.000000000000000000, 0.000000000000000000 ) ) ;
#9624=ADVANCED_FACE ( 'NONE', ( #21799 ), #14288, .F. ) ;
#9627=PLANE ( 'NONE',  #6650 ) ;
#9628=DIRECTION ( 'NONE',  ( 2.257144641399999941E-12, 0.000000000000000000, 1.000000000000000000 ) ) ;
#9632=EDGE_CURVE ( 'NONE', #6404, #12670, #19770, .T. ) ;
#9634=CARTESIAN_POINT ( 'NONE',  ( -14.60945070276051894, -41.53817725281877671, -150.0552959529999839 ) ) ;
#9635=CARTESIAN_POINT ( 'NONE',  ( 22.50000000000000000, 33.50000000000000000, -151.0552959529999839 ) ) ;
#9636=DIRECTION ( 'NONE',  ( 1.000000000000000000, 0.000000000000000000, 0.000000000000000000 ) ) ;
#9640=EDGE_CURVE ( 'NONE', #11584, #12574, #1694, .T. ) ;
#9642=CARTESIAN_POINT ( 'NONE',  ( 6.500000000000000000, 13.00000000000000000, -151.0552959529999839 ) ) ;
#9646=FACE_BOUND ( 'NONE', #4399, .T. ) ;
#9648=DIRECTION ( 'NONE',  ( 0.000000000000000000, -2.252420472359999842E-12, -1.000000000000000000 ) ) ;
#9653=ORIENTED_EDGE ( 'NONE', *, *, #14495, .F. ) ;
#9661=LINE ( 'NONE', #21954, #6366 ) ;
#9664=VERTEX_POINT ( 'NONE', #18906 ) ;
#9668=LINE ( 'NONE', #4571, #16501 ) ;
#9679=EDGE_CURVE ( 'NONE', #12200, #12791, #22387, .T. ) ;
#9686=AXIS2_PLACEMENT_3D ( 'NONE', #16933, #7877, #11563 ) ;
#9687=CARTESIAN_POINT ( 'NONE',  ( -4.500000000000000000, 34.00000000000000000, -150.0552959529999839 ) ) ;
#9690=ORIENTED_EDGE ( 'NONE', *, *, #21374, .T. ) ;
#9693=CARTESIAN_POINT ( 'NONE',  ( -14.60730091830126476, -46.00000000000000711, -150.0552959529999555 ) ) ;
#9695=EDGE_LOOP ( 'NONE', ( #13320, #11951, #14954, #22566 ) ) ;
#9700=DIRECTION ( 'NONE',  ( 0.000000000000000000, -1.000000000000000000, 0.000000000000000000 ) ) ;
#9703=ORIENTED_EDGE ( 'NONE', *, *, #22924, .F. ) ;
#9705=AXIS2_PLACEMENT_3D ( 'NONE', #18326, #10801, #5359 ) ;
#9708=ORIENTED_EDGE ( 'NONE', *, *, #14375, .T. ) ;
#9710=CARTESIAN_POINT ( 'NONE',  ( 1.133692148550000001, 51.50000000000000000, -136.0552959530000123 ) ) ;
#9715=ORIENTED_EDGE ( 'NONE', *, *, #8148, .F. ) ;
#9718=ORIENTED_EDGE ( 'NONE', *, *, #1721, .T. ) ;
#9726=ORIENTED_EDGE ( 'NONE', *, *, #19590, .T. ) ;
#9730=ORIENTED_EDGE ( 'NONE', *, *, #11688, .T. ) ;
#9738=CARTESIAN_POINT ( 'NONE',  ( 16.13369214829999976, -51.50000000000000000, -136.0552959530000123 ) ) ;
#9740=CARTESIAN_POINT ( 'NONE',  ( -10.00000000000000000, 19.50000000000000000, -150.0552959529999839 ) ) ;
#9743=DIRECTION ( 'NONE',  ( -1.000000000000000000, 0.000000000000000000, -2.273736754430000208E-12 ) ) ;
#9746=CARTESIAN_POINT ( 'NONE',  ( 0.000000000000000000, 0.000000000000000000, -150.0552959529999839 ) ) ;
#9763=CARTESIAN_POINT ( 'NONE',  ( 7.750000000000000000, -41.23606797749999942, -150.0552959529999839 ) ) ;
#9764=ORIENTED_EDGE ( 'NONE', *, *, #17234, .T. ) ;
#9766=AXIS2_PLACEMENT_3D ( 'NONE', #18806, #9628, #16902 ) ;
#9773=CARTESIAN_POINT ( 'NONE',  ( 7.930443943682751851, -33.22545875219810796, -150.0552959529999839 ) ) ;
#9782=EDGE_CURVE ( 'NONE', #565, #20697, #14989, .T. ) ;
#9785=DIRECTION ( 'NONE',  ( 0.000000000000000000, 0.000000000000000000, 1.000000000000000000 ) ) ;
#9799=LINE ( 'NONE', #20540, #19052 ) ;
#9804=EDGE_CURVE ( 'NONE', #9978, #7971, #7724, .T. ) ;
#9806=VECTOR ( 'NONE', #4871, 1000.000000000000000 ) ;
#9807=LINE ( 'NONE', #17201, #17053 ) ;
#9808=EDGE_CURVE ( 'NONE', #6526, #13263, #7953, .T. ) ;
#9821=ORIENTED_EDGE ( 'NONE', *, *, #21131, .T. ) ;
#9823=LINE ( 'NONE', #2372, #10585 ) ;
#9829=FACE_OUTER_BOUND ( 'NONE', #19239, .T. ) ;
#9831=ORIENTED_EDGE ( 'NONE', *, *, #16241, .F. ) ;
#9834=VECTOR ( 'NONE', #6388, 1000.000000000000000 ) ;
#9840=EDGE_CURVE ( 'NONE', #15915, #2624, #718, .T. ) ;
#9844=CARTESIAN_POINT ( 'NONE',  ( 1.133692148550000001, -51.00000000000000000, -137.0552959530000123 ) ) ;
#9851=FACE_OUTER_BOUND ( 'NONE', #7677, .T. ) ;
#9853=CARTESIAN_POINT ( 'NONE',  ( 25.94418247360000152, -46.04723021459999899, -149.5552959529999839 ) ) ;
#9854=EDGE_LOOP ( 'NONE', ( #16381, #4291, #8165, #4117, #4573, #20559, #5422 ) ) ;
#9855=CARTESIAN_POINT ( 'NONE',  ( 7.750000000000000000, -40.23606797749999942, -151.0552959529999839 ) ) ;
#9860=AXIS2_PLACEMENT_3D ( 'NONE', #1614, #21590, #8835 ) ;
#9861=CARTESIAN_POINT ( 'NONE',  ( 1.500000000000000000, -3.500000000000000000, -150.0552959529999839 ) ) ;
#9867=ORIENTED_EDGE ( 'NONE', *, *, #4844, .T. ) ;
#9884=DIRECTION ( 'NONE',  ( -1.000000000000000000, 0.000000000000000000, 0.000000000000000000 ) ) ;
#9891=CARTESIAN_POINT ( 'NONE',  ( 1.924189958818393276, 14.53742485369798842, -150.0552959530000123 ) ) ;
#9902=ORIENTED_EDGE ( 'NONE', *, *, #15587, .T. ) ;
#9908=LINE ( 'NONE', #15640, #18611 ) ;
#9909=CARTESIAN_POINT ( 'NONE',  ( 0.000000000000000000, -40.23606797749999942, -150.0552959529999839 ) ) ;
#9917=CARTESIAN_POINT ( 'NONE',  ( -13.86630785140000022, -50.50000000000000000, -137.0552959530000123 ) ) ;
#9920=CARTESIAN_POINT ( 'NONE',  ( 18.95053822279999878, -50.50000000000000000, -143.0552959529999839 ) ) ;
#9925=VECTOR ( 'NONE', #1102, 1000.000000000000000 ) ;
#9928=SURFACE_STYLE_USAGE ( .BOTH. , #916 ) ;
#9929=ORIENTED_EDGE ( 'NONE', *, *, #11917, .T. ) ;
#9930=CARTESIAN_POINT ( 'NONE',  ( 32.50000000000000000, 26.96379895119999759, -137.0552959530000123 ) ) ;
#9934=ORIENTED_EDGE ( 'NONE', *, *, #19440, .T. ) ;
#9935=LINE ( 'NONE', #15672, #17853 ) ;
#9939=LINE ( 'NONE', #4839, #21234 ) ;
#9940=ADVANCED_FACE ( 'NONE', ( #23190 ), #11750, .F. ) ;
#9945=AXIS2_PLACEMENT_3D ( 'NONE', #16512, #2367, #15076 ) ;
#9946=EDGE_CURVE ( 'NONE', #5050, #14322, #2658, .T. ) ;
#9948=EDGE_CURVE ( 'NONE', #18719, #22568, #8179, .T. ) ;
#9949=CARTESIAN_POINT ( 'NONE',  ( 25.11896946143725984, 38.01480899505094868, -150.0552959529999839 ) ) ;
#9950=ORIENTED_EDGE ( 'NONE', *, *, #17963, .T. ) ;
#9953=FACE_OUTER_BOUND ( 'NONE', #21098, .T. ) ;
#9955=EDGE_LOOP ( 'NONE', ( #21407, #9963, #14385, #18825 ) ) ;
#9956=CARTESIAN_POINT ( 'NONE',  ( 31.50000000000000000, 0.000000000000000000, -137.0552959530000123 ) ) ;
#9963=ORIENTED_EDGE ( 'NONE', *, *, #14649, .F. ) ;
#9966=DIRECTION ( 'NONE',  ( 0.000000000000000000, 0.000000000000000000, 1.000000000000000000 ) ) ;
#9974=DIRECTION ( 'NONE',  ( -0.7633862853691523176, 0.6459422414661291079, 0.000000000000000000 ) ) ;
#9978=VERTEX_POINT ( 'NONE', #1315 ) ;
#9979=CARTESIAN_POINT ( 'NONE',  ( 5.285243653077836612, -0.5780819699950525692, -150.0552959529999839 ) ) ;
#9982=LINE ( 'NONE', #10095, #8702 ) ;
#9984=CARTESIAN_POINT ( 'NONE',  ( 32.00000000000000000, 39.80430157320000006, -150.0552959529999839 ) ) ;
#9991=FACE_OUTER_BOUND ( 'NONE', #15571, .T. ) ;
#9995=PRODUCT_DEFINITION_FORMATION_WITH_SPECIFIED_SOURCE ( 'ANY', '', #4785, .NOT_KNOWN. ) ;
#9996=CARTESIAN_POINT ( 'NONE',  ( -15.00000000000000000, -43.00000000000000000, -140.0552959529999839 ) ) ;
#9997=EDGE_LOOP ( 'NONE', ( #8521, #5939, #18034, #19896 ) ) ;
#10026=ORIENTED_EDGE ( 'NONE', *, *, #20248, .T. ) ;
#10028=EDGE_CURVE ( 'NONE', #10724, #9007, #20087, .T. ) ;
#10041=LINE ( 'NONE', #9930, #12499 ) ;
#10058=AXIS2_PLACEMENT_3D ( 'NONE', #1443, #8445, #11894 ) ;
#10059=DIRECTION ( 'NONE',  ( -1.000000000000000000, 0.000000000000000000, 2.273736754430000208E-12 ) ) ;
#10068=DIRECTION ( 'NONE',  ( -0.7633862853691523176, 0.6459422414661291079, 0.000000000000000000 ) ) ;
#10069=CARTESIAN_POINT ( 'NONE',  ( 21.65635984007526105, -22.89900052719454493, -150.0552959529999839 ) ) ;
#10077=CARTESIAN_POINT ( 'NONE',  ( 19.59648046430000079, 50.76338628540000286, -150.0552959529999839 ) ) ;
#10079=VECTOR ( 'NONE', #19015, 1000.000000000000000 ) ;
#10092=DIRECTION ( 'NONE',  ( 0.000000000000000000, 0.000000000000000000, 1.000000000000000000 ) ) ;
#10093=EDGE_CURVE ( 'NONE', #12394, #2513, #17092, .T. ) ;
#10095=CARTESIAN_POINT ( 'NONE',  ( 31.50000000000000000, -40.03620104880000241, -143.0552959529999839 ) ) ;
#10109=EDGE_CURVE ( 'NONE', #18841, #4401, #20213, .T. ) ;
#10119=CARTESIAN_POINT ( 'NONE',  ( 4.109383212426824805, -2.038350857853872711, -150.0552959529999839 ) ) ;
#10122=PLANE ( 'NONE',  #18216 ) ;
#10126=LINE ( 'NONE', #8352, #1763 ) ;
#10127=CARTESIAN_POINT ( 'NONE',  ( -0.7600837004312114287, 18.55411937531333777, -150.0552959529999839 ) ) ;
#10131=AXIS2_PLACEMENT_3D ( 'NONE', #198, #16603, #7443 ) ;
#10132=CARTESIAN_POINT ( 'NONE',  ( 9.593637377583139170, -37.00248504027853613, -150.0552959529999839 ) ) ;
#10136=EDGE_CURVE ( 'NONE', #13352, #13163, #22794, .T. ) ;
#10138=ORIENTED_EDGE ( 'NONE', *, *, #20730, .T. ) ;
#10143=VERTEX_POINT ( 'NONE', #2366 ) ;
#10151=DIRECTION ( 'NONE',  ( 0.000000000000000000, 1.000000000000000000, 0.000000000000000000 ) ) ;
#10157=ORIENTED_EDGE ( 'NONE', *, *, #21023, .T. ) ;
#10160=ADVANCED_FACE ( 'NONE', ( #9586 ), #7802, .F. ) ;
#10164=ORIENTED_EDGE ( 'NONE', *, *, #5038, .F. ) ;
#10165=EDGE_CURVE ( 'NONE', #18702, #1936, #17574, .T. ) ;
#10173=FACE_OUTER_BOUND ( 'NONE', #2264, .T. ) ;
#10184=CARTESIAN_POINT ( 'NONE',  ( 24.33948587669790342, 34.09808825513669461, -150.0552959529999839 ) ) ;
#10197=ADVANCED_FACE ( 'NONE', ( #13990 ), #18999, .T. ) ;
#10200=VECTOR ( 'NONE', #9974, 1000.000000000000227 ) ;
#10214=ORIENTED_EDGE ( 'NONE', *, *, #2989, .T. ) ;
#10217=ADVANCED_FACE ( 'NONE', ( #10173 ), #17444, .T. ) ;
#10218=CARTESIAN_POINT ( 'NONE',  ( 19.13369214879999802, 50.49999999980000354, -150.0552959529999839 ) ) ;
#10221=CARTESIAN_POINT ( 'NONE',  ( 19.45666326950000169, -50.88169314249999786, -136.0552959530000123 ) ) ;
#10223=CARTESIAN_POINT ( 'NONE',  ( 1.133692148550000001, -50.50000000000000000, -137.0552959530000123 ) ) ;
#10224=CARTESIAN_POINT ( 'NONE',  ( 31.00000000000000000, 39.80430157320000006, -149.5552959529999839 ) ) ;
#10226=CARTESIAN_POINT ( 'NONE',  ( 24.28524365307783484, -17.57808196999505412, -150.0552959529999839 ) ) ;
#10229=AXIS2_PLACEMENT_3D ( 'NONE', #2030, #11259, #9357 ) ;
#10231=EDGE_CURVE ( 'NONE', #10837, #18382, #4929, .T. ) ;
#10234=PLANE ( 'NONE',  #8305 ) ;
#10237=FACE_OUTER_BOUND ( 'NONE', #22376, .T. ) ;
#10242=CARTESIAN_POINT ( 'NONE',  ( 6.000000000000000000, -3.301262168631092564, -150.0552959530000123 ) ) ;
#10244=VERTEX_POINT ( 'NONE', #13634 ) ;
#10246=EDGE_CURVE ( 'NONE', #19589, #4360, #9935, .T. ) ;
#10249=VECTOR ( 'NONE', #10068, 1000.000000000000227 ) ;
#10257=EDGE_CURVE ( 'NONE', #7545, #7540, #13512, .T. ) ;
#10258=CARTESIAN_POINT ( 'NONE',  ( 25.50000000000000000, 25.50000000000000000, -151.0552959529999839 ) ) ;
#10263=CARTESIAN_POINT ( 'NONE',  ( 3.763193976707701172, -36.41260098204946871, -150.0552959530000123 ) ) ;
#10269=CARTESIAN_POINT ( 'NONE',  ( -32.50000000000000000, 1.000000000000000000, -151.0552959529999839 ) ) ;
#10278=CARTESIAN_POINT ( 'NONE',  ( -32.50000000000000000, 1.000000000000000000, -150.0552959529999839 ) ) ;
#10280=CARTESIAN_POINT ( 'NONE',  ( -16.46164914215972885, -43.39061678754082862, -150.0552959530000123 ) ) ;
#10282=MECHANICAL_DESIGN_GEOMETRIC_PRESENTATION_REPRESENTATION('',(#11802),#20953);
#10287=EDGE_LOOP ( 'NONE', ( #17203, #2902, #18882, #8610 ) ) ;
#10288=DIRECTION ( 'NONE',  ( 0.000000000000000000, 0.000000000000000000, 1.000000000000000000 ) ) ;
#10306=EDGE_CURVE ( 'NONE', #11337, #8510, #3411, .T. ) ;
#10314=ORIENTED_EDGE ( 'NONE', *, *, #952, .F. ) ;
#10316=DIRECTION ( 'NONE',  ( -0.6459422414661291079, -0.7633862853691523176, -2.273736754430455399E-12 ) ) ;
#10317=ORIENTED_EDGE ( 'NONE', *, *, #6974, .F. ) ;
#10331=VECTOR ( 'NONE', #5342, 1000.000000000000000 ) ;
#10337=CARTESIAN_POINT ( 'NONE',  ( 19.91945158500000090, 51.14507942810000429, -150.0552959519999945 ) ) ;
#10338=DIRECTION ( 'NONE',  ( 1.000000000000000000, 0.000000000000000000, 0.000000000000000000 ) ) ;
#10342=DIRECTION ( 'NONE',  ( 1.000000000000000000, 0.000000000000000000, 0.000000000000000000 ) ) ;
#10344=DIRECTION ( 'NONE',  ( -1.000000000000000000, 0.000000000000000000, 0.000000000000000000 ) ) ;
#10345=DIRECTION ( 'NONE',  ( 0.000000000000000000, 0.000000000000000000, -1.000000000000000000 ) ) ;
#10348=ORIENTED_EDGE ( 'NONE', *, *, #15586, .T. ) ;
#10349=EDGE_CURVE ( 'NONE', #16889, #13555, #11001, .T. ) ;
#10351=DIRECTION ( 'NONE',  ( -0.000000000000000000, 1.000000000000000000, 0.000000000000000000 ) ) ;
#10366=DIRECTION ( 'NONE',  ( 0.000000000000000000, 0.000000000000000000, 1.000000000000000000 ) ) ;
#10384=ADVANCED_FACE ( 'NONE', ( #8861 ), #5303, .T. ) ;
#10385=ORIENTED_EDGE ( 'NONE', *, *, #10306, .T. ) ;
#10388=EDGE_CURVE ( 'NONE', #18640, #3680, #15754, .T. ) ;
#10400=ORIENTED_EDGE ( 'NONE', *, *, #6628, .T. ) ;
#10403=DIRECTION ( 'NONE',  ( 0.000000000000000000, -1.000000000000000000, -1.723073263340000007E-12 ) ) ;
#10406=EDGE_CURVE ( 'NONE', #21462, #9003, #5429, .T. ) ;
#10421=ORIENTED_EDGE ( 'NONE', *, *, #9190, .T. ) ;
#10422=DIRECTION ( 'NONE',  ( 0.000000000000000000, 0.000000000000000000, 1.000000000000000000 ) ) ;
#10423=DIRECTION ( 'NONE',  ( 0.000000000000000000, -1.000000000000000000, 0.000000000000000000 ) ) ;
#10432=EDGE_CURVE ( 'NONE', #6865, #4983, #14935, .T. ) ;
#10438=FACE_OUTER_BOUND ( 'NONE', #1417, .T. ) ;
#10441=DIRECTION ( 'NONE',  ( 1.000000000000000000, 0.000000000000000000, -2.257453483404482811E-12 ) ) ;
#10442=CIRCLE ( 'NONE', #10814, 2.000000000000000000 ) ;
#10456=VERTEX_POINT ( 'NONE', #22081 ) ;
#10460=CARTESIAN_POINT ( 'NONE',  ( 31.82297112100000192, -40.41789419119999849, -150.0552959529999839 ) ) ;
#10467=DIRECTION ( 'NONE',  ( -0.000000000000000000, 1.000000000000000000, 0.000000000000000000 ) ) ;
#10471=AXIS2_PLACEMENT_3D ( 'NONE', #12857, #12980, #16210 ) ;
#10473=VERTEX_POINT ( 'NONE', #5998 ) ;
#10474=DIRECTION ( 'NONE',  ( 0.000000000000000000, 1.000000000000000000, 0.000000000000000000 ) ) ;
#10485=ORIENTED_EDGE ( 'NONE', *, *, #11887, .T. ) ;
#10492=LINE ( 'NONE', #1488, #14828 ) ;
#10493=ORIENTED_EDGE ( 'NONE', *, *, #391, .F. ) ;
#10496=CARTESIAN_POINT ( 'NONE',  ( -12.60099947280546218, -41.15635984007524684, -150.0552959529999839 ) ) ;
#10507=CYLINDRICAL_SURFACE ( 'NONE', #3354, 7.500000000000006217 ) ;
#10512=CARTESIAN_POINT ( 'NONE',  ( 32.05742780190000474, 40.87448416769999682, -149.5552959529999839 ) ) ;
#10515=VECTOR ( 'NONE', #20258, 1000.000000000000000 ) ;
#10519=AXIS2_PLACEMENT_3D ( 'NONE', #2323, #15150, #20283 ) ;
#10522=ORIENTED_EDGE ( 'NONE', *, *, #21099, .T. ) ;
#10537=DIRECTION ( 'NONE',  ( 0.000000000000000000, 1.000000000000000000, 2.257144641399999941E-12 ) ) ;
#10540=ORIENTED_EDGE ( 'NONE', *, *, #1797, .F. ) ;
#10545=CARTESIAN_POINT ( 'NONE',  ( -5.246332636038733455, 43.48990303080123709, -150.0552959529999839 ) ) ;
#10548=ORIENTED_EDGE ( 'NONE', *, *, #11919, .T. ) ;
#10550=DIRECTION ( 'NONE',  ( 0.000000000000000000, 0.000000000000000000, 1.000000000000000000 ) ) ;
#10554=LINE ( 'NONE', #10909, #17044 ) ;
#10556=VECTOR ( 'NONE', #10288, 1000.000000000000000 ) ;
#10557=CARTESIAN_POINT ( 'NONE',  ( 20.50000000000000000, 19.50000000000000000, -151.0552959529999839 ) ) ;
#10558=ORIENTED_EDGE ( 'NONE', *, *, #18855, .F. ) ;
#10561=ADVANCED_FACE ( 'NONE', ( #17542 ), #19091, .F. ) ;
#10571=VECTOR ( 'NONE', #14282, 1000.000000000000000 ) ;
#10573=CARTESIAN_POINT ( 'NONE',  ( 0.8371776177479999248, 16.00000000000000000, -144.0552959529999839 ) ) ;
#10574=AXIS2_PLACEMENT_3D ( 'NONE', #7569, #18517, #2236 ) ;
#10582=DIRECTION ( 'NONE',  ( 1.000000000000000000, 0.000000000000000000, 0.000000000000000000 ) ) ;
#10585=VECTOR ( 'NONE', #14729, 1000.000000000000000 ) ;
#10590=DIRECTION ( 'NONE',  ( 0.000000000000000000, 0.000000000000000000, 1.000000000000000000 ) ) ;
#10592=CARTESIAN_POINT ( 'NONE',  ( 23.50000000000000000, -20.50000000000000000, -137.0552959530000123 ) ) ;
#10597=DIRECTION ( 'NONE',  ( -1.000000000000000000, 0.000000000000000000, 2.273736754430000208E-12 ) ) ;
#10601=DIRECTION ( 'NONE',  ( -2.257242012349999735E-12, 0.000000000000000000, 1.000000000000000000 ) ) ;
#10603=CARTESIAN_POINT ( 'NONE',  ( -32.50000000000000000, 21.50000000000000000, -151.0552959529999839 ) ) ;
#10612=VERTEX_POINT ( 'NONE', #783 ) ;
#10615=PLANE ( 'NONE',  #1154 ) ;
#10619=CARTESIAN_POINT ( 'NONE',  ( -14.80142434076114810, -44.50006722990159602, -150.0552959529999839 ) ) ;
#10622=CARTESIAN_POINT ( 'NONE',  ( -6.683153925719999222, -50.50000000000000000, -136.0552959530000123 ) ) ;
#10631=VECTOR ( 'NONE', #13631, 1000.000000000000000 ) ;
#10639=CARTESIAN_POINT ( 'NONE',  ( 18.95053822279999878, 50.00000000000000000, -150.5552959529999839 ) ) ;
#10647=VECTOR ( 'NONE', #9591, 1000.000000000000000 ) ;
#10649=EDGE_CURVE ( 'NONE', #22981, #12791, #9908, .T. ) ;
#10653=PLANE ( 'NONE',  #12882 ) ;
#10657=CARTESIAN_POINT ( 'NONE',  ( -32.50000000000000000, -43.00000000050000182, -137.0552959530000123 ) ) ;
#10659=AXIS2_PLACEMENT_3D ( 'NONE', #13528, #938, #19130 ) ;
#10666=ADVANCED_FACE ( 'NONE', ( #12054 ), #13487, .T. ) ;
#10667=CARTESIAN_POINT ( 'NONE',  ( -3.500000000000000000, 42.50000000000000000, -150.0552959529999839 ) ) ;
#10671=CARTESIAN_POINT ( 'NONE',  ( 13.13369214859999978, 51.50000000000000000, -136.0552959530000123 ) ) ;
#10683=EDGE_LOOP ( 'NONE', ( #12922, #10317, #5690, #18998 ) ) ;
#10699=CIRCLE ( 'NONE', #19845, 7.499999999999999112 ) ;
#10702=CARTESIAN_POINT ( 'NONE',  ( 5.285243653077851711, -6.421918030004944100, -150.0552959529999839 ) ) ;
#10705=ORIENTED_EDGE ( 'NONE', *, *, #18257, .T. ) ;
#10719=ORIENTED_EDGE ( 'NONE', *, *, #9125, .T. ) ;
#10724=VERTEX_POINT ( 'NONE', #10735 ) ;
#10731=DIRECTION ( 'NONE',  ( -0.7633862853691524286, -0.6459422414661292189, -2.187565684150435883E-17 ) ) ;
#10734=EDGE_CURVE ( 'NONE', #22797, #21113, #12292, .T. ) ;
#10735=CARTESIAN_POINT ( 'NONE',  ( -12.50000000000000000, 42.50000000000000000, -151.0552959529999839 ) ) ;
#10739=CARTESIAN_POINT ( 'NONE',  ( 18.98537695655051394, 19.88080765318867194, -150.0552959530000123 ) ) ;
#10748=CARTESIAN_POINT ( 'NONE',  ( 18.95053822279999878, -50.00000000000000000, -149.5552959529999839 ) ) ;
#10752=FACE_BOUND ( 'NONE', #14240, .T. ) ;
#10756=VERTEX_POINT ( 'NONE', #8711 ) ;
#10757=ADVANCED_FACE ( 'NONE', ( #1841 ), #21828, .T. ) ;
#10758=CARTESIAN_POINT ( 'NONE',  ( -5.660609041639971473, 24.90181682660303508, -150.0552959529999839 ) ) ;
#10761=ADVANCED_FACE ( 'NONE', ( #12647 ), #16229, .T. ) ;
#10765=AXIS2_PLACEMENT_3D ( 'NONE', #7088, #1750, #23508 ) ;
#10768=LINE ( 'NONE', #12090, #17061 ) ;
#10770=ORIENTED_EDGE ( 'NONE', *, *, #11550, .F. ) ;
#10771=FACE_OUTER_BOUND ( 'NONE', #10287, .T. ) ;
#10776=FACE_OUTER_BOUND ( 'NONE', #8349, .T. ) ;
#10780=CARTESIAN_POINT ( 'NONE',  ( -4.726769794318020246, 42.89852487308611018, -150.0552959529999839 ) ) ;
#10788=DIRECTION ( 'NONE',  ( 0.000000000000000000, 0.000000000000000000, -1.000000000000000000 ) ) ;
#10790=CARTESIAN_POINT ( 'NONE',  ( -32.50000000000000000, -36.00000000000000000, -149.5552959529999839 ) ) ;
#10799=ORIENTED_EDGE ( 'NONE', *, *, #6629, .F. ) ;
#10801=DIRECTION ( 'NONE',  ( 0.000000000000000000, 2.257144641399999941E-12, -1.000000000000000000 ) ) ;
#10803=B_SPLINE_CURVE_WITH_KNOTS ( 'NONE', 3,
 ( #3381, #17307, #10280, #17552, #1269, #14570, #59, #19809, #11093, #10619, #10977, #16355, #3736, #21946, #7068, #5281, #12654, #22060 ),
 .UNSPECIFIED., .F., .F.,
 ( 4, 2, 2, 2, 2, 2, 2, 2, 4 ),
 ( 0.000000000000000000, 0.1250000000000000000, 0.2500000000000000000, 0.3750000000000000000, 0.5000000000000000000, 0.6250000000000000000, 0.7500000000000000000, 0.8750000000000000000, 1.000000000000000000 ),
 .UNSPECIFIED. ) ;
#10808=ORIENTED_EDGE ( 'NONE', *, *, #15642, .T. ) ;
#10809=CARTESIAN_POINT ( 'NONE',  ( 19.77963439019999825, -51.26338628519999929, -149.5552959529999839 ) ) ;
#10814=AXIS2_PLACEMENT_3D ( 'NONE', #20829, #11417, #22262 ) ;
#10817=ORIENTED_EDGE ( 'NONE', *, *, #15497, .F. ) ;
#10837=VERTEX_POINT ( 'NONE', #9294 ) ;
#10838=EDGE_CURVE ( 'NONE', #6870, #4401, #16567, .T. ) ;
#10845=FACE_OUTER_BOUND ( 'NONE', #19303, .T. ) ;
#10846=ORIENTED_EDGE ( 'NONE', *, *, #7602, .F. ) ;
#10849=AXIS2_PLACEMENT_3D ( 'NONE', #8525, #21166, #12331 ) ;
#10857=DIRECTION ( 'NONE',  ( -0.000000000000000000, 1.000000000000000000, 0.000000000000000000 ) ) ;
#10861=CARTESIAN_POINT ( 'NONE',  ( 4.750000000000000000, -47.00000000000000000, -150.0552959529999839 ) ) ;
#10864=CARTESIAN_POINT ( 'NONE',  ( 31.50000000000000000, 20.96379895120000114, -136.0552959530000123 ) ) ;
#10868=UNCERTAINTY_MEASURE_WITH_UNIT (LENGTH_MEASURE( 1.000000000000000082E-05 ), #13599, 'distance_accuracy_value', 'NONE');
#10875=CARTESIAN_POINT ( 'NONE',  ( 22.50000000000000000, 33.50000000000000000, -150.5552959529999839 ) ) ;
#10883=ORIENTED_EDGE ( 'NONE', *, *, #10388, .F. ) ;
#10901=DIRECTION ( 'NONE',  ( -0.7633862853691524286, -0.6459422414661292189, 2.734434900580546249E-18 ) ) ;
#10903=ORIENTED_EDGE ( 'NONE', *, *, #16925, .T. ) ;
#10907=CARTESIAN_POINT ( 'NONE',  ( 31.50000000010000178, 40.03620104870000063, -149.5552959529999839 ) ) ;
#10909=CARTESIAN_POINT ( 'NONE',  ( 32.05742780199999942, -40.87448416760000214, -150.0552959529999839 ) ) ;
#10920=VERTEX_POINT ( 'NONE', #19973 ) ;
#10933=CARTESIAN_POINT ( 'NONE',  ( 19.04211518569999839, 51.50000000000000000, -149.5552959529999839 ) ) ;
#10937=CARTESIAN_POINT ( 'NONE',  ( 1.133692148550000001, -51.50000000000000000, -137.0552959530000123 ) ) ;
#10949=VECTOR ( 'NONE', #20237, 1000.000000000000000 ) ;
#10952=ORIENTED_EDGE ( 'NONE', *, *, #5041, .F. ) ;
#10954=EDGE_CURVE ( 'NONE', #20932, #802, #12589, .T. ) ;
#10964=CARTESIAN_POINT ( 'NONE',  ( 18.95053822279999878, 50.50000000000000000, -149.5552959529999839 ) ) ;
#10973=EDGE_CURVE ( 'NONE', #12372, #8058, #11034, .T. ) ;
#10975=CARTESIAN_POINT ( 'NONE',  ( -32.50000000000000000, -43.00000000050000182, -137.0552959530000123 ) ) ;
#10977=CARTESIAN_POINT ( 'NONE',  ( -14.60938321243984106, -44.46164914216203812, -150.0552959529999839 ) ) ;
#10979=ADVANCED_FACE ( 'NONE', ( #7359 ), #14617, .F. ) ;
#10980=LINE ( 'NONE', #22065, #18461 ) ;
#10981=EDGE_CURVE ( 'NONE', #1116, #3167, #11603, .T. ) ;
#10983=CARTESIAN_POINT ( 'NONE',  ( -4.500000000000000000, 40.00000000000000000, -150.5552959529999839 ) ) ;
#10991=VECTOR ( 'NONE', #4476, 1000.000000000000000 ) ;
#10995=ORIENTED_EDGE ( 'NONE', *, *, #20300, .F. ) ;
#11001=LINE ( 'NONE', #16140, #20505 ) ;
#11006=ORIENTED_EDGE ( 'NONE', *, *, #9076, .F. ) ;
#11008=EDGE_CURVE ( 'NONE', #3612, #19891, #12581, .T. ) ;
#11012=CARTESIAN_POINT ( 'NONE',  ( -32.50000000000000000, 12.00000000000000000, -144.0552959529999839 ) ) ;
#11016=ORIENTED_EDGE ( 'NONE', *, *, #5311, .T. ) ;
#11017=FACE_OUTER_BOUND ( 'NONE', #20476, .T. ) ;
#11020=ORIENTED_EDGE ( 'NONE', *, *, #10109, .F. ) ;
#11032=CYLINDRICAL_SURFACE ( 'NONE', #2761, 3.000000000000000000 ) ;
#11034=LINE ( 'NONE', #12820, #22419 ) ;
#11038=DIRECTION ( 'NONE',  ( 1.457928428160000110E-12, 1.723197716179999783E-12, -1.000000000000000000 ) ) ;
#11052=CARTESIAN_POINT ( 'NONE',  ( 19.34345092960000301, -49.66753540199999151, -149.5552959529999839 ) ) ;
#11053=ORIENTED_EDGE ( 'NONE', *, *, #13454, .T. ) ;
#11060=ORIENTED_EDGE ( 'NONE', *, *, #18981, .T. ) ;
#11061=ADVANCED_FACE ( 'NONE', ( #8040 ), #11254, .F. ) ;
#11066=B_SPLINE_CURVE_WITH_KNOTS ( 'NONE', 1,
 ( #9549, #11208 ),
 .UNSPECIFIED., .F., .F.,
 ( 2, 2 ),
 ( -6.000000000000000000, 6.000000000000000000 ),
 .UNSPECIFIED. ) ;
#11067=ORIENTED_EDGE ( 'NONE', *, *, #22118, .F. ) ;
#11070=FACE_OUTER_BOUND ( 'NONE', #20981, .T. ) ;
#11080=CARTESIAN_POINT ( 'NONE',  ( 32.50000000000000000, -27.03620104879999886, -137.0552959530000123 ) ) ;
#11081=EDGE_CURVE ( 'NONE', #16174, #7366, #13516, .T. ) ;
#11090=VECTOR ( 'NONE', #7806, 1000.000000000000000 ) ;
#11091=CARTESIAN_POINT ( 'NONE',  ( -7.500000000000000000, 48.50000000000000000, -150.0552959529999839 ) ) ;
#11092=LINE ( 'NONE', #18259, #18225 ) ;
#11093=CARTESIAN_POINT ( 'NONE',  ( -15.19857565924485421, -44.49993277009840398, -150.0552959529999839 ) ) ;
#11097=EDGE_CURVE ( 'NONE', #1062, #17719, #22225, .T. ) ;
#11098=CARTESIAN_POINT ( 'NONE',  ( 8.750000000000000000, -47.00000000000000000, -150.5552959529999839 ) ) ;
#11101=DIRECTION ( 'NONE',  ( 0.000000000000000000, 1.000000000000000000, 0.000000000000000000 ) ) ;
#11109=ORIENTED_EDGE ( 'NONE', *, *, #18269, .F. ) ;
#11111=DIRECTION ( 'NONE',  ( 0.6459422414661314393, 0.7633862853691505412, 0.000000000000000000 ) ) ;
#11118=DIRECTION ( 'NONE',  ( 1.000000000000000000, 0.000000000000000000, 0.000000000000000000 ) ) ;
#11123=FACE_OUTER_BOUND ( 'NONE', #7501, .T. ) ;
#11134=ADVANCED_FACE ( 'NONE', ( #4721 ), #11965, .F. ) ;
#11135=ORIENTED_EDGE ( 'NONE', *, *, #11097, .T. ) ;
#11138=ORIENTED_EDGE ( 'NONE', *, *, #15760, .F. ) ;
#11142=DIRECTION ( 'NONE',  ( 1.000000000000000000, 0.000000000000000000, 0.000000000000000000 ) ) ;
#11144=DIRECTION ( 'NONE',  ( 0.000000000000000000, -2.257144641399999941E-12, -1.000000000000000000 ) ) ;
#11148=LINE ( 'NONE', #20674, #6787 ) ;
#11149=ORIENTED_EDGE ( 'NONE', *, *, #11430, .F. ) ;
#11152=ORIENTED_EDGE ( 'NONE', *, *, #10257, .F. ) ;
#11153=CARTESIAN_POINT ( 'NONE',  ( 3.742764529247745386, -4.809518488836389771, -150.0552959529999839 ) ) ;
#11155=VECTOR ( 'NONE', #13460, 1000.000000000000000 ) ;
#11158=ORIENTED_EDGE ( 'NONE', *, *, #17277, .F. ) ;
#11161=ORIENTED_EDGE ( 'NONE', *, *, #5188, .T. ) ;
#11170=CARTESIAN_POINT ( 'NONE',  ( -12.50000000000000000, 42.50000000000000000, -150.0552959529999839 ) ) ;
#11171=DIRECTION ( 'NONE',  ( -1.000000000000000000, 0.000000000000000000, 0.000000000000000000 ) ) ;
#11183=CARTESIAN_POINT ( 'NONE',  ( 32.00000000000000000, 20.96379895120000114, -136.0552959530000123 ) ) ;
#11188=DIRECTION ( 'NONE',  ( -0.7071067811865475727, -0.7071067811865475727, 0.000000000000000000 ) ) ;
#11189=EDGE_CURVE ( 'NONE', #2513, #7104, #5187, .T. ) ;
#11194=DIRECTION ( 'NONE',  ( -0.000000000000000000, 1.000000000000000000, 0.000000000000000000 ) ) ;
#11196=LINE ( 'NONE', #22278, #19555 ) ;
#11197=ORIENTED_EDGE ( 'NONE', *, *, #15071, .T. ) ;
#11203=DIRECTION ( 'NONE',  ( 1.000000000000000000, 0.000000000000000000, 0.000000000000000000 ) ) ;
#11208=CARTESIAN_POINT ( 'NONE',  ( 13.13369214859999978, 50.50000000000000000, -137.0552959530000123 ) ) ;
#11209=CARTESIAN_POINT ( 'NONE',  ( -16.50000000000000000, -43.00000000000000000, -150.0552959529999839 ) ) ;
#11229=ADVANCED_FACE ( 'NONE', ( #18287 ), #17803, .F. ) ;
#11231=AXIS2_PLACEMENT_3D ( 'NONE', #9192, #14451, #170 ) ;
#11234=PLANE ( 'NONE',  #6501 ) ;
#11243=CARTESIAN_POINT ( 'NONE',  ( -13.15635984007524684, -45.39900052719453782, -150.0552959530000123 ) ) ;
#11254=PLANE ( 'NONE',  #9121 ) ;
#11255=LINE ( 'NONE', #13170, #9047 ) ;
#11256=ORIENTED_EDGE ( 'NONE', *, *, #10432, .T. ) ;
#11259=DIRECTION ( 'NONE',  ( 1.000000000000000000, 0.000000000000000000, 0.000000000000000000 ) ) ;
#11271=DIRECTION ( 'NONE',  ( 1.000000000000000000, 0.000000000000000000, 0.000000000000000000 ) ) ;
#11273=ORIENTED_EDGE ( 'NONE', *, *, #11810, .F. ) ;
#11276=DIRECTION ( 'NONE',  ( -1.000000000000000000, 0.000000000000000000, 0.000000000000000000 ) ) ;
#11278=VERTEX_POINT ( 'NONE', #1370 ) ;
#11286=ORIENTED_EDGE ( 'NONE', *, *, #21641, .T. ) ;
#11296=DIRECTION ( 'NONE',  ( -1.000000000000000000, 0.000000000000000000, 2.257144641399999941E-12 ) ) ;
#11298=VERTEX_POINT ( 'NONE', #8130 ) ;
#11308=CARTESIAN_POINT ( 'NONE',  ( 31.50000000000000000, 40.03620104880000241, -150.0552959529999839 ) ) ;
#11309=DIRECTION ( 'NONE',  ( -1.000000000000000000, 0.000000000000000000, 0.000000000000000000 ) ) ;
#11312=FACE_BOUND ( 'NONE', #12145, .T. ) ;
#11313=EDGE_CURVE ( 'NONE', #16877, #968, #21241, .T. ) ;
#11323=DIRECTION ( 'NONE',  ( 0.000000000000000000, -1.000000000000000000, 0.000000000000000000 ) ) ;
#11324=DIRECTION ( 'NONE',  ( 0.000000000000000000, 0.000000000000000000, 1.000000000000000000 ) ) ;
#11327=EDGE_LOOP ( 'NONE', ( #5892, #1035, #23152, #5659 ) ) ;
#11337=VERTEX_POINT ( 'NONE', #17421 ) ;
#11340=LINE ( 'NONE', #4228, #11759 ) ;
#11348=AXIS2_PLACEMENT_3D ( 'NONE', #11797, #19076, #764 ) ;
#11349=DIRECTION ( 'NONE',  ( -1.000000000000000000, 0.000000000000000000, 0.000000000000000000 ) ) ;
#11360=VERTEX_POINT ( 'NONE', #10278 ) ;
#11361=CARTESIAN_POINT ( 'NONE',  ( 8.250000000000000000, -42.23606797749999942, -150.0552959529999839 ) ) ;
#11363=ORIENTED_EDGE ( 'NONE', *, *, #3569, .T. ) ;
#11366=ADVANCED_FACE ( 'NONE', ( #6707 ), #17548, .T. ) ;
#11370=DIRECTION ( 'NONE',  ( 0.000000000000000000, -1.000000000000000000, 2.257144641399999941E-12 ) ) ;
#11371=CARTESIAN_POINT ( 'NONE',  ( 31.50000000000000000, 40.03620104880000241, -143.0552959529999839 ) ) ;
#11378=ORIENTED_EDGE ( 'NONE', *, *, #7992, .F. ) ;
#11396=LINE ( 'NONE', #22359, #10949 ) ;
#11400=ADVANCED_FACE ( 'NONE', ( #17188 ), #11819, .F. ) ;
#11408=ORIENTED_EDGE ( 'NONE', *, *, #22410, .T. ) ;
#11415=ORIENTED_EDGE ( 'NONE', *, *, #9125, .F. ) ;
#11416=CARTESIAN_POINT ( 'NONE',  ( -6.774730888589999722, -50.50000000000000000, -149.5552959529999839 ) ) ;
#11417=DIRECTION ( 'NONE',  ( -1.000000000000000000, 0.000000000000000000, 2.257144641399999941E-12 ) ) ;
#11418=CARTESIAN_POINT ( 'NONE',  ( 32.14594224149999491, 40.79958733410000349, -136.0552959519999945 ) ) ;
#11423=EDGE_CURVE ( 'NONE', #20008, #7366, #14447, .T. ) ;
#11424=DIRECTION ( 'NONE',  ( 0.000000000000000000, 0.000000000000000000, -1.000000000000000000 ) ) ;
#11427=CIRCLE ( 'NONE', #10659, 1.500000000000001332 ) ;
#11428=AXIS2_PLACEMENT_3D ( 'NONE', #5857, #5743, #3968 ) ;
#11429=DIRECTION ( 'NONE',  ( 0.000000000000000000, 0.000000000000000000, -1.000000000000000000 ) ) ;
#11430=EDGE_CURVE ( 'NONE', #4966, #14773, #14568, .T. ) ;
#11435=CARTESIAN_POINT ( 'NONE',  ( 15.50000000000000000, 39.50000000000000000, -151.0552959529999839 ) ) ;
#11444=EDGE_LOOP ( 'NONE', ( #21518, #12485, #850, #20925 ) ) ;
#11445=VECTOR ( 'NONE', #14534, 1000.000000000000000 ) ;
#11446=CARTESIAN_POINT ( 'NONE',  ( 22.50000000000000000, 39.50000000000000000, -150.5552959529999839 ) ) ;
#11450=CARTESIAN_POINT ( 'NONE',  ( -7.500000000000000000, 48.50000000000000000, -151.0552959529999839 ) ) ;
#11463=ORIENTED_EDGE ( 'NONE', *, *, #19567, .T. ) ;
#11471=DIRECTION ( 'NONE',  ( 2.256967945870000144E-12, 0.000000000000000000, 1.000000000000000000 ) ) ;
#11478=ORIENTED_EDGE ( 'NONE', *, *, #4894, .F. ) ;
#11483=CARTESIAN_POINT ( 'NONE',  ( 1.133692148550000001, -50.50000000000000000, -143.0552959529999839 ) ) ;
#11488=LINE ( 'NONE', #15197, #19364 ) ;
#11489=CARTESIAN_POINT ( 'NONE',  ( 12.15117705467117126, 25.45516771066687056, -150.0552959529999839 ) ) ;
#11494=CARTESIAN_POINT ( 'NONE',  ( -1.550733472792253709, 45.02071668630156154, -150.0552959530000123 ) ) ;
#11499=DIRECTION ( 'NONE',  ( 1.000000000000000000, 0.000000000000000000, 0.000000000000000000 ) ) ;
#11503=AXIS2_PLACEMENT_3D ( 'NONE', #1752, #3528, #20060 ) ;
#11504=CYLINDRICAL_SURFACE ( 'NONE', #5549, 1.500000000000001332 ) ;
#11509=FACE_OUTER_BOUND ( 'NONE', #12108, .T. ) ;
#11512=VERTEX_POINT ( 'NONE', #21474 ) ;
#11515=LINE ( 'NONE', #9499, #23200 ) ;
#11517=DIRECTION ( 'NONE',  ( -1.000000000000000000, 0.000000000000000000, 0.000000000000000000 ) ) ;
#11518=PLANE ( 'NONE',  #7288 ) ;
#11543=DIRECTION ( 'NONE',  ( -1.000000000000000000, 0.000000000000000000, 0.000000000000000000 ) ) ;
#11550=EDGE_CURVE ( 'NONE', #16851, #20008, #168, .T. ) ;
#11551=CARTESIAN_POINT ( 'NONE',  ( 1.133692148550000001, 51.00000000000000000, -137.0552959530000123 ) ) ;
#11553=FACE_OUTER_BOUND ( 'NONE', #9512, .T. ) ;
#11556=B_SPLINE_CURVE_WITH_KNOTS ( 'NONE', 3,
 ( #12960, #14747, #16884, #2389, #13309, #20578, #13423, #7828, #20462, #16996 ),
 .UNSPECIFIED., .F., .F.,
 ( 4, 2, 2, 2, 4 ),
 ( 0.000000000000000000, 0.2500000000000000000, 0.5000000000000000000, 0.7500000000000000000, 1.000000000000000000 ),
 .UNSPECIFIED. ) ;
#11557=EDGE_CURVE ( 'NONE', #7409, #4521, #12880, .T. ) ;
#11559=EDGE_CURVE ( 'NONE', #11681, #10612, #7756, .T. ) ;
#11560=CARTESIAN_POINT ( 'NONE',  ( 4.553999924767063057, 13.23986818282688560, -150.0552959530000123 ) ) ;
#11563=DIRECTION ( 'NONE',  ( 1.000000000000000000, 0.000000000000000000, 0.000000000000000000 ) ) ;
#11564=EDGE_CURVE ( 'NONE', #12200, #11512, #3853, .T. ) ;
#11568=ORIENTED_EDGE ( 'NONE', *, *, #4815, .T. ) ;
#11572=ORIENTED_EDGE ( 'NONE', *, *, #11641, .F. ) ;
#11574=DIRECTION ( 'NONE',  ( -0.6459422414661291079, -0.7633862853691523176, -2.245315045000450442E-12 ) ) ;
#11576=ORIENTED_EDGE ( 'NONE', *, *, #12218, .F. ) ;
#11584=VERTEX_POINT ( 'NONE', #11091 ) ;
#11593=CARTESIAN_POINT ( 'NONE',  ( -18.00000000000000000, -43.00000000000000000, -140.0552959529999839 ) ) ;
#11594=VERTEX_POINT ( 'NONE', #18724 ) ;
#11597=ORIENTED_EDGE ( 'NONE', *, *, #21398, .T. ) ;
#11603=LINE ( 'NONE', #11723, #22071 ) ;
#11606=CARTESIAN_POINT ( 'NONE',  ( 6.500000000000000000, 13.00000000000000000, -150.0552959529999839 ) ) ;
#11612=CARTESIAN_POINT ( 'NONE',  ( 24.90191174485078207, 38.33948587671270047, -150.0552959529999839 ) ) ;
#11613=ADVANCED_FACE ( 'NONE', ( #22059 ), #15139, .F. ) ;
#11617=EDGE_LOOP ( 'NONE', ( #13152, #23102, #6682, #1539 ) ) ;
#11621=DIRECTION ( 'NONE',  ( 0.7633862853691523176, 0.6459422414661291079, 0.000000000000000000 ) ) ;
#11628=CYLINDRICAL_SURFACE ( 'NONE', #19539, 7.500000000000007105 ) ;
#11631=DIRECTION ( 'NONE',  ( -1.457881434619999915E-12, -1.723066134219999902E-12, 1.000000000000000000 ) ) ;
#11632=ORIENTED_EDGE ( 'NONE', *, *, #12296, .T. ) ;
#11634=VERTEX_POINT ( 'NONE', #18475 ) ;
#11637=ORIENTED_EDGE ( 'NONE', *, *, #6179, .F. ) ;
#11640=AXIS2_PLACEMENT_3D ( 'NONE', #4941, #8497, #1502 ) ;
#11641=EDGE_CURVE ( 'NONE', #5292, #3235, #4206, .T. ) ;
#11643=CARTESIAN_POINT ( 'NONE',  ( 1.578081969995051459, -2.714756346922164720, -150.0552959530000123 ) ) ;
#11646=CARTESIAN_POINT ( 'NONE',  ( -32.50000000000000000, -51.50000000000000000, -136.0552959519999945 ) ) ;
#11648=DIRECTION ( 'NONE',  ( 2.259525899719999991E-12, 0.000000000000000000, -1.000000000000000000 ) ) ;
#11651=CARTESIAN_POINT ( 'NONE',  ( 18.95053822279999878, -51.50000000000000000, -150.0552959529999839 ) ) ;
#11656=VECTOR ( 'NONE', #6085, 1000.000000000000000 ) ;
#11658=CARTESIAN_POINT ( 'NONE',  ( -32.50000000000000000, -50.00000000000000000, -149.5552959529999839 ) ) ;
#11659=CARTESIAN_POINT ( 'NONE',  ( -1.500000000000000000, 44.50000000000000000, -150.5552959529999839 ) ) ;
#11661=VERTEX_POINT ( 'NONE', #15378 ) ;
#11672=AXIS2_PLACEMENT_3D ( 'NONE', #21845, #19930, #1628 ) ;
#11677=CARTESIAN_POINT ( 'NONE',  ( 0.8371776177479999248, 14.00000000000000000, -144.0552959529999839 ) ) ;
#11681=VERTEX_POINT ( 'NONE', #19066 ) ;
#11688=EDGE_CURVE ( 'NONE', #13163, #11906, #15491, .T. ) ;
#11690=DIRECTION ( 'NONE',  ( 0.000000000000000000, -1.100009706970682018E-14, -1.000000000000000000 ) ) ;
#11708=CIRCLE ( 'NONE', #10574, 1.500000000000000444 ) ;
#11710=FILL_AREA_STYLE_COLOUR ( '', #8430 ) ;
#11716=ORIENTED_EDGE ( 'NONE', *, *, #12811, .F. ) ;
#11723=CARTESIAN_POINT ( 'NONE',  ( -13.86630785140000022, -51.00000000000000000, -137.0552959530000123 ) ) ;
#11726=AXIS2_PLACEMENT_3D ( 'NONE', #19546, #14422, #10474 ) ;
#11734=ORIENTED_EDGE ( 'NONE', *, *, #3938, .F. ) ;
#11744=VERTEX_POINT ( 'NONE', #10269 ) ;
#11748=VERTEX_POINT ( 'NONE', #11805 ) ;
#11750=CYLINDRICAL_SURFACE ( 'NONE', #3793, 2.000000000000002220 ) ;
#11755=DIRECTION ( 'NONE',  ( 0.000000000000000000, 1.000000000000000000, 0.000000000000000000 ) ) ;
#11757=EDGE_LOOP ( 'NONE', ( #18405, #19142, #7278, #9821 ) ) ;
#11759=VECTOR ( 'NONE', #9436, 1000.000000000000000 ) ;
#11762=PLANE ( 'NONE',  #2906 ) ;
#11771=DIRECTION ( 'NONE',  ( 1.000000000000000000, 0.000000000000000000, 0.000000000000000000 ) ) ;
#11774=MANIFOLD_SOLID_BREP ( 'lock_assembly.1\\lock body.1\\PartBody', #442 ) ;
#11782=CARTESIAN_POINT ( 'NONE',  ( -13.86630785140000022, -50.50000000000000000, -137.0552959530000123 ) ) ;
#11785=EDGE_LOOP ( 'NONE', ( #9162, #23360, #9867, #4569 ) ) ;
#11787=CARTESIAN_POINT ( 'NONE',  ( -24.00000000000000000, 21.50000000000000000, -151.0552959529999839 ) ) ;
#11792=CARTESIAN_POINT ( 'NONE',  ( -31.00000000000000000, 1.000000000000000000, -149.5552959529999839 ) ) ;
#11796=CARTESIAN_POINT ( 'NONE',  ( -32.50000000000000000, -43.00000000050000182, -137.0552959530000123 ) ) ;
#11797=CARTESIAN_POINT ( 'NONE',  ( -31.00000000000000000, -50.00000000000000000, -149.5552959529999839 ) ) ;
#11798=AXIS2_PLACEMENT_3D ( 'NONE', #18160, #3531, #7213 ) ;
#11802=STYLED_ITEM ( 'NONE', ( #5043 ), #11774 ) ;
#11803=CARTESIAN_POINT ( 'NONE',  ( 6.446555752716397691, -33.00005219093733899, -150.0552959529999555 ) ) ;
#11805=CARTESIAN_POINT ( 'NONE',  ( 19.13369214879999802, -50.49999999980000354, -149.5552959529999839 ) ) ;
#11810=EDGE_CURVE ( 'NONE', #5668, #12787, #13722, .T. ) ;
#11817=ORIENTED_EDGE ( 'NONE', *, *, #2979, .F. ) ;
#11819=PLANE ( 'NONE',  #2690 ) ;
#11820=EDGE_CURVE ( 'NONE', #14446, #19224, #6814, .T. ) ;
#11827=ADVANCED_FACE ( 'NONE', ( #3365 ), #6938, .T. ) ;
#11829=DIRECTION ( 'NONE',  ( -2.256894259919999967E-12, 0.000000000000000000, 1.000000000000000000 ) ) ;
#11840=ORIENTED_EDGE ( 'NONE', *, *, #16494, .T. ) ;
#11848=ORIENTED_EDGE ( 'NONE', *, *, #2280, .T. ) ;
#11855=CARTESIAN_POINT ( 'NONE',  ( 25.49993271304583331, 36.89748944256449192, -150.0552959529999839 ) ) ;
#11859=EDGE_CURVE ( 'NONE', #2045, #14976, #160, .T. ) ;
#11873=VECTOR ( 'NONE', #520, 1000.000000000000000 ) ;
#11874=DIRECTION ( 'NONE',  ( 0.7071067811865474617, 0.7071067811865475727, 0.000000000000000000 ) ) ;
#11875=EDGE_LOOP ( 'NONE', ( #18800, #2385, #6695, #19434 ) ) ;
#11881=PLANE ( 'NONE',  #14408 ) ;
#11887=EDGE_CURVE ( 'NONE', #3797, #1160, #5263, .T. ) ;
#11889=ADVANCED_FACE ( 'NONE', ( #1479 ), #8699, .F. ) ;
#11892=ORIENTED_EDGE ( 'NONE', *, *, #11189, .T. ) ;
#11894=DIRECTION ( 'NONE',  ( 1.000000000000000000, 0.000000000000000000, -2.257453483404482811E-12 ) ) ;
#11895=CARTESIAN_POINT ( 'NONE',  ( 21.98914305888729714, -17.87864083493722944, -150.0552959529999839 ) ) ;
#11898=DIRECTION ( 'NONE',  ( 0.000000000000000000, -1.000000000000000000, 0.000000000000000000 ) ) ;
#11906=VERTEX_POINT ( 'NONE', #21822 ) ;
#11917=EDGE_CURVE ( 'NONE', #14539, #18280, #5506, .T. ) ;
#11919=EDGE_CURVE ( 'NONE', #13247, #7407, #18297, .T. ) ;
#11920=DIRECTION ( 'NONE',  ( 0.000000000000000000, 0.000000000000000000, 1.000000000000000000 ) ) ;
#11922=FACE_OUTER_BOUND ( 'NONE', #12622, .T. ) ;
#11929=ORIENTED_EDGE ( 'NONE', *, *, #1267, .F. ) ;
#11932=LINE ( 'NONE', #5048, #174 ) ;
#11940=CARTESIAN_POINT ( 'NONE',  ( -32.00000000000000000, 1.000000000000000000, -137.0552959530000123 ) ) ;
#11942=DIRECTION ( 'NONE',  ( 2.257144641399999941E-12, 0.000000000000000000, 1.000000000000000000 ) ) ;
#11949=PLANE ( 'NONE',  #15886 ) ;
#11951=ORIENTED_EDGE ( 'NONE', *, *, #21042, .T. ) ;
#11954=CARTESIAN_POINT ( 'NONE',  ( 19.77963439039999827, 51.26338628509999751, -150.0552959529999839 ) ) ;
#11960=ORIENTED_EDGE ( 'NONE', *, *, #18735, .T. ) ;
#11962=CARTESIAN_POINT ( 'NONE',  ( 31.00000000000000000, 0.000000000000000000, -151.0552959529999839 ) ) ;
#11965=PLANE ( 'NONE',  #3449 ) ;
#11974=VECTOR ( 'NONE', #19951, 1000.000000000000000 ) ;
#11983=ORIENTED_EDGE ( 'NONE', *, *, #9056, .T. ) ;
#11984=DIRECTION ( 'NONE',  ( 1.000000000000000000, 0.000000000000000000, 0.000000000000000000 ) ) ;
#11985=EDGE_CURVE ( 'NONE', #844, #11278, #15604, .T. ) ;
#11987=ORIENTED_EDGE ( 'NONE', *, *, #4158, .T. ) ;
#11989=EDGE_CURVE ( 'NONE', #2949, #4038, #6554, .T. ) ;
#11990=FACE_OUTER_BOUND ( 'NONE', #16309, .T. ) ;
#11992=DIRECTION ( 'NONE',  ( 0.000000000000000000, 0.000000000000000000, 1.000000000000000000 ) ) ;
#11994=DIRECTION ( 'NONE',  ( 0.000000000000000000, -1.000000000000000000, 0.000000000000000000 ) ) ;
#11999=EDGE_CURVE ( 'NONE', #10920, #1386, #21202, .T. ) ;
#12004=ADVANCED_FACE ( 'NONE', ( #9991 ), #22737, .F. ) ;
#12007=CARTESIAN_POINT ( 'NONE',  ( -7.500000000000000000, 25.50000000000000000, -150.0552959529999839 ) ) ;
#12021=CARTESIAN_POINT ( 'NONE',  ( 0.000000000000000000, 25.50000000000000000, -150.0552959529999839 ) ) ;
#12023=LINE ( 'NONE', #17507, #935 ) ;
#12031=DIRECTION ( 'NONE',  ( -1.000000000000000000, 0.000000000000000000, 0.000000000000000000 ) ) ;
#12037=DIRECTION ( 'NONE',  ( 0.000000000000000000, 1.000000000000000000, 2.257453483404482811E-12 ) ) ;
#12039=VERTEX_POINT ( 'NONE', #18213 ) ;
#12043=CARTESIAN_POINT ( 'NONE',  ( 9.167789811881178252, -37.80184220689855579, -150.0552959529999839 ) ) ;
#12044=FACE_OUTER_BOUND ( 'NONE', #23507, .T. ) ;
#12046=VECTOR ( 'NONE', #12773, 1000.000000000000000 ) ;
#12054=FACE_OUTER_BOUND ( 'NONE', #19387, .T. ) ;
#12061=CARTESIAN_POINT ( 'NONE',  ( -14.21475634692216339, -40.07808196999505412, -150.0552959529999839 ) ) ;
#12066=FACE_OUTER_BOUND ( 'NONE', #167, .T. ) ;
#12068=DIRECTION ( 'NONE',  ( 1.457985068979999943E-12, -1.723073263340000007E-12, -1.000000000000000000 ) ) ;
#12070=CIRCLE ( 'NONE', #4468, 2.000000000000000000 ) ;
#12090=CARTESIAN_POINT ( 'NONE',  ( 19.13369214859999801, -51.00000000000000000, -150.0552959529999839 ) ) ;
#12091=AXIS2_PLACEMENT_3D ( 'NONE', #7717, #7483, #5934 ) ;
#12093=EDGE_LOOP ( 'NONE', ( #22018, #5180, #6515, #19670 ) ) ;
#12103=ORIENTED_EDGE ( 'NONE', *, *, #5041, .T. ) ;
#12108=EDGE_LOOP ( 'NONE', ( #14093, #8538, #9387, #23213, #21240, #17187, #671 ) ) ;
#12110=AXIS2_PLACEMENT_3D ( 'NONE', #2701, #22926, #15190 ) ;
#12112=ORIENTED_EDGE ( 'NONE', *, *, #2362, .F. ) ;
#12118=CARTESIAN_POINT ( 'NONE',  ( 18.95053822279999878, 50.00000000000000000, -151.0552959529999839 ) ) ;
#12121=CARTESIAN_POINT ( 'NONE',  ( 7.421918030004944988, -2.714756346922159835, -150.0552959530000123 ) ) ;
#12125=LINE ( 'NONE', #12603, #3789 ) ;
#12128=DIRECTION ( 'NONE',  ( 1.000000000000000000, 0.000000000000000000, -2.245315046049999660E-12 ) ) ;
#12130=EDGE_CURVE ( 'NONE', #2045, #17877, #7380, .T. ) ;
#12132=LINE ( 'NONE', #15949, #1844 ) ;
#12133=LINE ( 'NONE', #6313, #20967 ) ;
#12135=CARTESIAN_POINT ( 'NONE',  ( -13.86630785140000022, 51.50000000000000000, -136.0552959530000123 ) ) ;
#12137=VERTEX_POINT ( 'NONE', #10809 ) ;
#12140=LINE ( 'NONE', #12021, #6802 ) ;
#12145=EDGE_LOOP ( 'NONE', ( #15843, #18168 ) ) ;
#12160=LINE ( 'NONE', #13592, #22769 ) ;
#12161=VERTEX_POINT ( 'NONE', #16310 ) ;
#12164=EDGE_CURVE ( 'NONE', #18803, #21084, #16432, .T. ) ;
#12166=DIRECTION ( 'NONE',  ( 0.7633862853691523176, 0.6459422414661291079, 0.000000000000000000 ) ) ;
#12168=EDGE_CURVE ( 'NONE', #1863, #8058, #20, .T. ) ;
#12171=CARTESIAN_POINT ( 'NONE',  ( -3.500000000000000000, 44.50000000000000000, -151.0552959529999839 ) ) ;
#12182=CARTESIAN_POINT ( 'NONE',  ( 17.88080765318374077, 24.01462304344178023, -150.0552959529999839 ) ) ;
#12183=PLANE ( 'NONE',  #20384 ) ;
#12198=DIRECTION ( 'NONE',  ( 1.000000000000000000, 0.000000000000000000, 0.000000000000000000 ) ) ;
#12200=VERTEX_POINT ( 'NONE', #5709 ) ;
#12204=EDGE_LOOP ( 'NONE', ( #14658, #15535, #5871, #11273 ) ) ;
#12205=DIRECTION ( 'NONE',  ( 0.000000000000000000, 0.000000000000000000, 1.000000000000000000 ) ) ;
#12211=CARTESIAN_POINT ( 'NONE',  ( 1.133692148550000001, -51.50000000000000000, -136.0552959530000123 ) ) ;
#12212=LINE ( 'NONE', #19491, #2642 ) ;
#12215=ORIENTED_EDGE ( 'NONE', *, *, #12272, .T. ) ;
#12218=EDGE_CURVE ( 'NONE', #18451, #7409, #7604, .T. ) ;
#12223=DIRECTION ( 'NONE',  ( 0.7633862853691524286, 0.6459422414661292189, -5.800915303671161101E-15 ) ) ;
#12225=FACE_BOUND ( 'NONE', #1751, .T. ) ;
#12234=AXIS2_PLACEMENT_3D ( 'NONE', #8993, #21285, #21762 ) ;
#12236=CIRCLE ( 'NONE', #13001, 1.500000000000001332 ) ;
#12237=AXIS2_PLACEMENT_3D ( 'NONE', #20328, #11144, #11370 ) ;
#12264=CARTESIAN_POINT ( 'NONE',  ( 13.13369214859999978, -51.50000000000000000, -136.0552959530000123 ) ) ;
#12270=VERTEX_POINT ( 'NONE', #21496 ) ;
#12272=EDGE_CURVE ( 'NONE', #3235, #9183, #8737, .T. ) ;
#12281=ORIENTED_EDGE ( 'NONE', *, *, #15129, .F. ) ;
#12283=SURFACE_STYLE_USAGE ( .BOTH. , #17293 ) ;
#12290=EDGE_CURVE ( 'NONE', #13032, #21821, #22930, .T. ) ;
#12292=LINE ( 'NONE', #12525, #21291 ) ;
#12294=ORIENTED_EDGE ( 'NONE', *, *, #4659, .F. ) ;
#12296=EDGE_CURVE ( 'NONE', #12161, #14060, #3172, .T. ) ;
#12299=CARTESIAN_POINT ( 'NONE',  ( -17.62135916506278122, -41.48914305888730780, -150.0552959530000123 ) ) ;
#12302=LINE ( 'NONE', #5162, #21891 ) ;
#12309=CARTESIAN_POINT ( 'NONE',  ( 25.96278831640000107, -46.03148680910000223, -136.0552959530000123 ) ) ;
#12311=ORIENTED_EDGE ( 'NONE', *, *, #15053, .F. ) ;
#12312=CARTESIAN_POINT ( 'NONE',  ( 4.500000000000000000, -3.500000000000000000, -140.0552959529999839 ) ) ;
#12317=CARTESIAN_POINT ( 'NONE',  ( -6.719401811558778803, 19.57621958799323636, -150.0552959530000123 ) ) ;
#12318=CARTESIAN_POINT ( 'NONE',  ( 32.50000000000000000, 40.03620104880000241, -150.0552959529999839 ) ) ;
#12328=FACE_OUTER_BOUND ( 'NONE', #15434, .T. ) ;
#12331=DIRECTION ( 'NONE',  ( 1.000000000000000000, 0.000000000000000000, 2.257453483404482811E-12 ) ) ;
#12337=CARTESIAN_POINT ( 'NONE',  ( -4.510008323426233368, 42.75347665030082567, -150.0552959530000123 ) ) ;
#12339=ORIENTED_EDGE ( 'NONE', *, *, #14375, .F. ) ;
#12347=CARTESIAN_POINT ( 'NONE',  ( -3.500000000000000000, 46.50000000000000000, -150.0552959529999839 ) ) ;
#12358=EDGE_CURVE ( 'NONE', #6962, #20386, #4995, .T. ) ;
#12359=CARTESIAN_POINT ( 'NONE',  ( -7.500000000000000000, 45.50000000000000000, -150.0552959529999839 ) ) ;
#12365=ORIENTED_EDGE ( 'NONE', *, *, #12944, .F. ) ;
#12366=CARTESIAN_POINT ( 'NONE',  ( 32.50000000000000000, 0.000000000000000000, -149.5552959529999839 ) ) ;
#12368=LINE ( 'NONE', #10460, #19745 ) ;
#12372=VERTEX_POINT ( 'NONE', #186 ) ;
#12373=ADVANCED_FACE ( 'NONE', ( #14341 ), #21852, .F. ) ;
#12388=CARTESIAN_POINT ( 'NONE',  ( 4.554119375321583618, 27.76008370043824769, -150.0552959529999839 ) ) ;
#12394=VERTEX_POINT ( 'NONE', #3753 ) ;
#12395=VECTOR ( 'NONE', #6194, 1000.000000000000000 ) ;
#12406=CARTESIAN_POINT ( 'NONE',  ( -15.78524365307784549, -40.07808196999505412, -150.0552959529999839 ) ) ;
#12420=EDGE_CURVE ( 'NONE', #14107, #23105, #9209, .T. ) ;
#12423=PLANE ( 'NONE',  #5340 ) ;
#12428=AXIS2_PLACEMENT_3D ( 'NONE', #10748, #5526, #17459 ) ;
#12430=CARTESIAN_POINT ( 'NONE',  ( -7.102348325422107145, 25.49999999999999645, -150.0552959530000123 ) ) ;
#12431=EDGE_CURVE ( 'NONE', #20852, #21170, #4570, .T. ) ;
#12437=DIRECTION ( 'NONE',  ( 1.000000000000000000, 0.000000000000000000, 0.000000000000000000 ) ) ;
#12440=CARTESIAN_POINT ( 'NONE',  ( -7.500000000000000000, 45.50000000000000000, -151.0552959529999839 ) ) ;
#12446=ORIENTED_EDGE ( 'NONE', *, *, #18269, .T. ) ;
#12461=LINE ( 'NONE', #23422, #10331 ) ;
#12471=PLANE ( 'NONE',  #1024 ) ;
#12485=ORIENTED_EDGE ( 'NONE', *, *, #10093, .F. ) ;
#12491=DIRECTION ( 'NONE',  ( 0.000000000000000000, 0.000000000000000000, 1.000000000000000000 ) ) ;
#12496=FACE_OUTER_BOUND ( 'NONE', #15440, .T. ) ;
#12497=ORIENTED_EDGE ( 'NONE', *, *, #21266, .F. ) ;
#12499=VECTOR ( 'NONE', #918, 1000.000000000000000 ) ;
#12502=VECTOR ( 'NONE', #20001, 1000.000000000000000 ) ;
#12525=CARTESIAN_POINT ( 'NONE',  ( 18.95053822279999878, -50.99999999949999818, -150.0552959529999839 ) ) ;
#12530=CYLINDRICAL_SURFACE ( 'NONE', #11231, 2.000000000000002220 ) ;
#12531=CARTESIAN_POINT ( 'NONE',  ( -32.50000000000000000, -17.50000000000000000, -151.0552959529999839 ) ) ;
#12539=PLANE ( 'NONE',  #12824 ) ;
#12540=CIRCLE ( 'NONE', #2313, 3.000000000000000000 ) ;
#12541=ORIENTED_EDGE ( 'NONE', *, *, #7034, .T. ) ;
#12544=ORIENTED_EDGE ( 'NONE', *, *, #3569, .F. ) ;
#12550=DIRECTION ( 'NONE',  ( 0.000000000000000000, 0.000000000000000000, 1.000000000000000000 ) ) ;
#12551=ADVANCED_FACE ( 'NONE', ( #19913 ), #20031, .T. ) ;
#12559=ORIENTED_EDGE ( 'NONE', *, *, #6340, .F. ) ;
#12562=DIRECTION ( 'NONE',  ( 0.6459422414661292189, -0.7633862853691524286, 2.257144641400451094E-12 ) ) ;
#12566=EDGE_CURVE ( 'NONE', #3293, #3797, #18011, .T. ) ;
#12574=VERTEX_POINT ( 'NONE', #9052 ) ;
#12577=CARTESIAN_POINT ( 'NONE',  ( -10.00000000000000000, 25.50000000000000000, -150.0552959529999839 ) ) ;
#12579=ORIENTED_EDGE ( 'NONE', *, *, #10136, .F. ) ;
#12581=B_SPLINE_CURVE_WITH_KNOTS ( 'NONE', 1,
 ( #22456, #6266 ),
 .UNSPECIFIED., .F., .F.,
 ( 2, 2 ),
 ( -12.63369214860000156, 6.000000000000000000 ),
 .UNSPECIFIED. ) ;
#12588=ADVANCED_FACE ( 'NONE', ( #162 ), #7296, .F. ) ;
#12589=LINE ( 'NONE', #20091, #22054 ) ;
#12603=CARTESIAN_POINT ( 'NONE',  ( -32.50000000000000000, 21.50000000000000000, -150.5552959529999839 ) ) ;
#12604=EDGE_LOOP ( 'NONE', ( #9690, #5129, #20517, #11987 ) ) ;
#12605=LINE ( 'NONE', #19879, #16568 ) ;
#12607=FACE_OUTER_BOUND ( 'NONE', #17561, .T. ) ;
#12610=VECTOR ( 'NONE', #20934, 1000.000000000000000 ) ;
#12613=AXIS2_PLACEMENT_3D ( 'NONE', #5240, #12491, #23449 ) ;
#12615=CARTESIAN_POINT ( 'NONE',  ( 8.750000000000000000, -40.23606797749999942, -150.0552959529999839 ) ) ;
#12621=DIRECTION ( 'NONE',  ( 0.7633862853691524286, -0.6459422414661292189, 2.187565684170436280E-17 ) ) ;
#12622=EDGE_LOOP ( 'NONE', ( #6390, #7798, #9272, #15138 ) ) ;
#12623=ADVANCED_FACE ( 'NONE', ( #4418 ), #9533, .T. ) ;
#12647=FACE_OUTER_BOUND ( 'NONE', #21967, .T. ) ;
#12653=CARTESIAN_POINT ( 'NONE',  ( 17.88103053855265401, 20.98519100495539291, -150.0552959529999839 ) ) ;
#12654=CARTESIAN_POINT ( 'NONE',  ( -13.50000000000000355, -43.19908942272522268, -150.0552959529999839 ) ) ;
#12660=CYLINDRICAL_SURFACE ( 'NONE', #16223, 0.4999999999999936717 ) ;
#12664=ORIENTED_EDGE ( 'NONE', *, *, #20248, .F. ) ;
#12670=VERTEX_POINT ( 'NONE', #20267 ) ;
#12675=DIRECTION ( 'NONE',  ( 0.000000000000000000, 0.000000000000000000, 1.000000000000000000 ) ) ;
#12685=DIRECTION ( 'NONE',  ( -1.000000000000000000, 0.000000000000000000, 2.257144641399999941E-12 ) ) ;
#12686=VERTEX_POINT ( 'NONE', #13105 ) ;
#12688=DIRECTION ( 'NONE',  ( 1.000000000000000000, 0.000000000000000000, 0.000000000000000000 ) ) ;
#12689=ORIENTED_EDGE ( 'NONE', *, *, #11313, .F. ) ;
#12691=FACE_BOUND ( 'NONE', #16946, .T. ) ;
#12698=ORIENTED_EDGE ( 'NONE', *, *, #770, .T. ) ;
#12699=EDGE_CURVE ( 'NONE', #4966, #21958, #20986, .T. ) ;
#12700=EDGE_LOOP ( 'NONE', ( #23180, #13394, #12879, #754 ) ) ;
#12707=VERTEX_POINT ( 'NONE', #7748 ) ;
#12708=LINE ( 'NONE', #20097, #2631 ) ;
#12721=CARTESIAN_POINT ( 'NONE',  ( 1.500000000000000000, -3.500000000000000000, -140.0552959529999839 ) ) ;
#12723=CARTESIAN_POINT ( 'NONE',  ( 26.50000000000000000, -20.50000000000000000, -143.5552959529999839 ) ) ;
#12724=ORIENTED_EDGE ( 'NONE', *, *, #13398, .F. ) ;
#12728=CARTESIAN_POINT ( 'NONE',  ( 3.714756346922168273, -6.421918030004948541, -150.0552959529999839 ) ) ;
#12741=ORIENTED_EDGE ( 'NONE', *, *, #7758, .F. ) ;
#12748=CIRCLE ( 'NONE', #13117, 3.000000000000000000 ) ;
#12754=CARTESIAN_POINT ( 'NONE',  ( 19.59648046430000079, 50.76338628540000286, -149.5552959529999839 ) ) ;
#12758=DIRECTION ( 'NONE',  ( 0.000000000000000000, 0.000000000000000000, 1.000000000000000000 ) ) ;
#12773=DIRECTION ( 'NONE',  ( 0.000000000000000000, 0.000000000000000000, 1.000000000000000000 ) ) ;
#12779=ORIENTED_EDGE ( 'NONE', *, *, #13398, .T. ) ;
#12785=DIRECTION ( 'NONE',  ( 0.000000000000000000, 2.259525899719999991E-12, 1.000000000000000000 ) ) ;
#12787=VERTEX_POINT ( 'NONE', #15833 ) ;
#12788=DIRECTION ( 'NONE',  ( 1.000000000000000000, 0.000000000000000000, 0.000000000000000000 ) ) ;
#12791=VERTEX_POINT ( 'NONE', #13932 ) ;
#12795=VECTOR ( 'NONE', #17722, 1000.000000000000000 ) ;
#12796=CARTESIAN_POINT ( 'NONE',  ( 4.500000000000000000, -3.500000000000000000, -140.0552959529999839 ) ) ;
#12799=CARTESIAN_POINT ( 'NONE',  ( 8.750000000000000000, -39.23606797749999942, -150.0552959529999839 ) ) ;
#12801=CARTESIAN_POINT ( 'NONE',  ( 4.800813058665234223, -47.52045733082537993, -150.0552959530000123 ) ) ;
#12810=FACE_OUTER_BOUND ( 'NONE', #23297, .T. ) ;
#12811=EDGE_CURVE ( 'NONE', #15840, #22265, #4777, .T. ) ;
#12814=ORIENTED_EDGE ( 'NONE', *, *, #5311, .F. ) ;
#12820=CARTESIAN_POINT ( 'NONE',  ( 32.00000000000000000, 39.80430157320000006, -149.5552959529999839 ) ) ;
#12824=AXIS2_PLACEMENT_3D ( 'NONE', #3515, #1053, #18146 ) ;
#12828=CARTESIAN_POINT ( 'NONE',  ( 3.190307906134843829, -4.257167980435450083, -150.0552959529999271 ) ) ;
#12829=EDGE_CURVE ( 'NONE', #567, #19467, #10699, .T. ) ;
#12834=FACE_BOUND ( 'NONE', #18673, .T. ) ;
#12837=LINE ( 'NONE', #12723, #16293 ) ;
#12839=ORIENTED_EDGE ( 'NONE', *, *, #11859, .T. ) ;
#12841=VECTOR ( 'NONE', #14808, 1000.000000000000000 ) ;
#12842=DIRECTION ( 'NONE',  ( 1.000000000000000000, 0.000000000000000000, 0.000000000000000000 ) ) ;
#12843=CARTESIAN_POINT ( 'NONE',  ( 4.892699081698736130, -6.500000000000000000, -150.0552959529999839 ) ) ;
#12851=ORIENTED_EDGE ( 'NONE', *, *, #11557, .T. ) ;
#12856=VECTOR ( 'NONE', #20556, 1000.000000000000000 ) ;
#12857=CARTESIAN_POINT ( 'NONE',  ( -31.00000000000000000, -50.00000000000000000, -149.5552959529999839 ) ) ;
#12859=AXIS2_PLACEMENT_3D ( 'NONE', #15098, #709, #11276 ) ;
#12861=CARTESIAN_POINT ( 'NONE',  ( -3.500000000000000000, 34.00000000000000000, -150.0552959529999839 ) ) ;
#12869=EDGE_CURVE ( 'NONE', #16889, #7959, #9562, .T. ) ;
#12871=DIRECTION ( 'NONE',  ( -0.7633862853691523176, 0.6459422414661291079, 0.000000000000000000 ) ) ;
#12873=CARTESIAN_POINT ( 'NONE',  ( 32.50000000000000000, -21.03620104879999886, -137.0552959530000123 ) ) ;
#12876=ORIENTED_EDGE ( 'NONE', *, *, #14483, .F. ) ;
#12879=ORIENTED_EDGE ( 'NONE', *, *, #21562, .T. ) ;
#12880=LINE ( 'NONE', #281, #1585 ) ;
#12882=AXIS2_PLACEMENT_3D ( 'NONE', #17933, #1650, #23403 ) ;
#12883=FACE_OUTER_BOUND ( 'NONE', #22215, .T. ) ;
#12884=CARTESIAN_POINT ( 'NONE',  ( 19.91945158500000090, 51.14507942810000429, -149.5552959529999839 ) ) ;
#12893=FACE_OUTER_BOUND ( 'NONE', #22184, .T. ) ;
#12896=CIRCLE ( 'NONE', #5679, 0.5000000000000004441 ) ;
#12904=LINE ( 'NONE', #14692, #3945 ) ;
#12908=DIRECTION ( 'NONE',  ( 0.000000000000000000, 1.000000000000000000, 0.000000000000000000 ) ) ;
#12918=ADVANCED_FACE ( 'NONE', ( #16655 ), #11518, .F. ) ;
#12922=ORIENTED_EDGE ( 'NONE', *, *, #17106, .F. ) ;
#12928=EDGE_LOOP ( 'NONE', ( #21110, #816, #19270, #22563 ) ) ;
#12937=CARTESIAN_POINT ( 'NONE',  ( 11.07581004119133539, 26.46257514629612118, -150.0552959530000123 ) ) ;
#12940=DIRECTION ( 'NONE',  ( 0.000000000000000000, 0.000000000000000000, 1.000000000000000000 ) ) ;
#12942=CYLINDRICAL_SURFACE ( 'NONE', #1505, 1.500000000000000444 ) ;
#12943=EDGE_CURVE ( 'NONE', #8645, #3037, #3117, .T. ) ;
#12944=EDGE_CURVE ( 'NONE', #903, #17493, #16774, .T. ) ;
#12960=CARTESIAN_POINT ( 'NONE',  ( -5.500000000000000000, 44.50000000000000000, -150.0552959529999839 ) ) ;
#12967=DIRECTION ( 'NONE',  ( -2.257144641399999941E-12, 0.000000000000000000, -1.000000000000000000 ) ) ;
#12971=AXIS2_PLACEMENT_3D ( 'NONE', #16455, #11429, #20721 ) ;
#12972=ORIENTED_EDGE ( 'NONE', *, *, #9437, .T. ) ;
#12976=ORIENTED_EDGE ( 'NONE', *, *, #605, .F. ) ;
#12979=DIRECTION ( 'NONE',  ( -1.000000000000000000, 0.000000000000000000, 2.257144641399999941E-12 ) ) ;
#12980=DIRECTION ( 'NONE',  ( 0.000000000000000000, -1.000000000000000000, 0.000000000000000000 ) ) ;
#12981=DIRECTION ( 'NONE',  ( 0.000000000000000000, 1.000000000000000000, 0.000000000000000000 ) ) ;
#12982=CARTESIAN_POINT ( 'NONE',  ( 32.50000000000000000, 32.96379895120000469, -136.5552959530000123 ) ) ;
#12984=DIRECTION ( 'NONE',  ( -2.252420472359999842E-12, 0.000000000000000000, 1.000000000000000000 ) ) ;
#12995=DIRECTION ( 'NONE',  ( 0.000000000000000000, 0.000000000000000000, -1.000000000000000000 ) ) ;
#13001=AXIS2_PLACEMENT_3D ( 'NONE', #15482, #20844, #2648 ) ;
#13004=DIRECTION ( 'NONE',  ( 0.000000000000000000, -1.000000000000000000, 0.000000000000000000 ) ) ;
#13007=FACE_OUTER_BOUND ( 'NONE', #16276, .T. ) ;
#13008=ORIENTED_EDGE ( 'NONE', *, *, #21868, .T. ) ;
#13011=CARTESIAN_POINT ( 'NONE',  ( 13.09818317338255156, 38.33939095839281208, -150.0552959529999839 ) ) ;
#13015=EDGE_CURVE ( 'NONE', #16420, #21462, #367, .T. ) ;
#13030=EDGE_CURVE ( 'NONE', #3680, #3138, #5712, .T. ) ;
#13032=VERTEX_POINT ( 'NONE', #20245 ) ;
#13038=CARTESIAN_POINT ( 'NONE',  ( -32.50000000000000000, -50.00000000000000000, -143.3052959529999839 ) ) ;
#13043=CARTESIAN_POINT ( 'NONE',  ( 8.351115582531676296, -48.22632467507040133, -150.0552959529999839 ) ) ;
#13056=ADVANCED_FACE ( 'NONE', ( #9851 ), #15579, .T. ) ;
#13060=DIRECTION ( 'NONE',  ( 0.000000000000000000, -1.000000000000000000, 0.000000000000000000 ) ) ;
#13061=ORIENTED_EDGE ( 'NONE', *, *, #7468, .F. ) ;
#13078=ORIENTED_EDGE ( 'NONE', *, *, #15724, .F. ) ;
#13099=CARTESIAN_POINT ( 'NONE',  ( -32.50000000000000000, -36.00000000000000000, -149.5552959529999839 ) ) ;
#13100=FACE_OUTER_BOUND ( 'NONE', #14992, .T. ) ;
#13105=CARTESIAN_POINT ( 'NONE',  ( 19.13369214859999801, 50.50000000000000000, -136.0552959530000123 ) ) ;
#13109=ORIENTED_EDGE ( 'NONE', *, *, #11557, .F. ) ;
#13117=AXIS2_PLACEMENT_3D ( 'NONE', #12796, #16267, #7554 ) ;
#13123=DIRECTION ( 'NONE',  ( 2.257144641399999941E-12, 0.000000000000000000, -1.000000000000000000 ) ) ;
#13126=CARTESIAN_POINT ( 'NONE',  ( 4.020454867573966418, -37.28105831637246581, -150.0552959530000123 ) ) ;
#13130=EDGE_LOOP ( 'NONE', ( #14979, #7573, #19557, #17532, #17754, #3763, #22896, #21004 ) ) ;
#13146=CARTESIAN_POINT ( 'NONE',  ( -2.500000000000000000, 34.00000000000000000, -150.0552959529999839 ) ) ;
#13151=PLANE ( 'NONE',  #19036 ) ;
#13152=ORIENTED_EDGE ( 'NONE', *, *, #11564, .F. ) ;
#13157=CARTESIAN_POINT ( 'NONE',  ( -31.50000000000000000, 10.25000000000000000, -149.5552959529999839 ) ) ;
#13163=VERTEX_POINT ( 'NONE', #1071 ) ;
#13164=DIRECTION ( 'NONE',  ( 0.000000000000000000, 0.000000000000000000, -1.000000000000000000 ) ) ;
#13165=DIRECTION ( 'NONE',  ( -0.7633862853691523176, 0.6459422414661291079, 0.000000000000000000 ) ) ;
#13170=CARTESIAN_POINT ( 'NONE',  ( -32.50000000000000000, 50.00000000000000000, -150.5552959529999839 ) ) ;
#13171=EDGE_LOOP ( 'NONE', ( #1167, #23393, #12839, #1457 ) ) ;
#13174=CARTESIAN_POINT ( 'NONE',  ( 31.50000000000000000, -40.03620104880000241, -149.5552959529999839 ) ) ;
#13188=ORIENTED_EDGE ( 'NONE', *, *, #14649, .T. ) ;
#13191=ORIENTED_EDGE ( 'NONE', *, *, #20608, .T. ) ;
#13198=AXIS2_PLACEMENT_3D ( 'NONE', #22234, #11499, #18778 ) ;
#13203=ORIENTED_EDGE ( 'NONE', *, *, #10649, .T. ) ;
#13204=ORIENTED_EDGE ( 'NONE', *, *, #11688, .F. ) ;
#13208=FACE_OUTER_BOUND ( 'NONE', #9159, .T. ) ;
#13210=EDGE_LOOP ( 'NONE', ( #5325, #20381, #5262, #1768 ) ) ;
#13213=AXIS2_PLACEMENT_3D ( 'NONE', #2066, #2301, #9174 ) ;
#13221=DIRECTION ( 'NONE',  ( 0.000000000000000000, -1.000000000000000000, 0.000000000000000000 ) ) ;
#13225=FACE_BOUND ( 'NONE', #14080, .T. ) ;
#13228=AXIS2_PLACEMENT_3D ( 'NONE', #3233, #10467, #3008 ) ;
#13229=VECTOR ( 'NONE', #8094, 1000.000000000000000 ) ;
#13232=ORIENTED_EDGE ( 'NONE', *, *, #9437, .F. ) ;
#13233=DIRECTION ( 'NONE',  ( 0.000000000000000000, 0.000000000000000000, 1.000000000000000000 ) ) ;
#13239=PLANE ( 'NONE',  #8619 ) ;
#13247=VERTEX_POINT ( 'NONE', #15331 ) ;
#13256=VERTEX_POINT ( 'NONE', #10671 ) ;
#13261=CARTESIAN_POINT ( 'NONE',  ( 22.00000000000000000, -20.50000000000000000, -136.0552959530000123 ) ) ;
#13263=VERTEX_POINT ( 'NONE', #21771 ) ;
#13264=AXIS2_PLACEMENT_3D ( 'NONE', #21413, #15699, #8300 ) ;
#13268=LINE ( 'NONE', #4007, #4103 ) ;
#13274=VERTEX_POINT ( 'NONE', #3437 ) ;
#13275=DIRECTION ( 'NONE',  ( 0.000000000000000000, -1.000000000000000000, 0.000000000000000000 ) ) ;
#13280=DIRECTION ( 'NONE',  ( 1.000000000000000000, 0.000000000000000000, 0.000000000000000000 ) ) ;
#13285=DIRECTION ( 'NONE',  ( -0.7633862853691524286, -0.6459422414661292189, 5.745404152441153618E-15 ) ) ;
#13301=DIRECTION ( 'NONE',  ( 0.000000000000000000, 1.000000000000000000, -2.245315044999999693E-12 ) ) ;
#13302=VECTOR ( 'NONE', #14987, 1000.000000000000000 ) ;
#13309=CARTESIAN_POINT ( 'NONE',  ( -5.101475126953193495, 45.72676979428539568, -150.0552959529999839 ) ) ;
#13316=ORIENTED_EDGE ( 'NONE', *, *, #15724, .T. ) ;
#13320=ORIENTED_EDGE ( 'NONE', *, *, #21398, .F. ) ;
#13328=ORIENTED_EDGE ( 'NONE', *, *, #7700, .T. ) ;
#13331=DIRECTION ( 'NONE',  ( 0.000000000000000000, 0.000000000000000000, -1.000000000000000000 ) ) ;
#13334=LINE ( 'NONE', #617, #21189 ) ;
#13336=FACE_OUTER_BOUND ( 'NONE', #22493, .T. ) ;
#13346=DIRECTION ( 'NONE',  ( 0.000000000000000000, 0.000000000000000000, 1.000000000000000000 ) ) ;
#13348=ADVANCED_FACE ( 'NONE', ( #15925, #23192 ), #21414, .T. ) ;
#13351=EDGE_CURVE ( 'NONE', #5909, #22853, #12461, .T. ) ;
#13352=VERTEX_POINT ( 'NONE', #18309 ) ;
#13356=AXIS2_PLACEMENT_3D ( 'NONE', #2074, #4314, #9180 ) ;
#13363=FACE_OUTER_BOUND ( 'NONE', #692, .T. ) ;
#13365=CARTESIAN_POINT ( 'NONE',  ( 6.148946002022614543, -33.04517854815976108, -150.0552959529999839 ) ) ;
#13367=CARTESIAN_POINT ( 'NONE',  ( -7.500000000000000000, 42.50000000000000000, -151.0552959529999839 ) ) ;
#13377=ADVANCED_FACE ( 'NONE', ( #15198 ), #11032, .T. ) ;
#13381=EDGE_LOOP ( 'NONE', ( #2850, #22874 ) ) ;
#13390=DIRECTION ( 'NONE',  ( 0.000000000000000000, 0.000000000000000000, 1.000000000000000000 ) ) ;
#13392=ORIENTED_EDGE ( 'NONE', *, *, #23355, .F. ) ;
#13393=CARTESIAN_POINT ( 'NONE',  ( -32.50000000000000000, 50.50000000000000000, -149.5552959529999839 ) ) ;
#13394=ORIENTED_EDGE ( 'NONE', *, *, #22820, .T. ) ;
#13398=EDGE_CURVE ( 'NONE', #21024, #16708, #2477, .T. ) ;
#13403=ADVANCED_FACE ( 'NONE', ( #688 ), #22223, .F. ) ;
#13421=CARTESIAN_POINT ( 'NONE',  ( 20.50000000000000000, 25.50000000000000000, -150.5552959529999839 ) ) ;
#13423=CARTESIAN_POINT ( 'NONE',  ( -4.510096969224879793, 46.24633263602949995, -150.0552959529999839 ) ) ;
#13430=DIRECTION ( 'NONE',  ( 1.000000000000000000, 0.000000000000000000, 0.000000000000000000 ) ) ;
#13436=DIRECTION ( 'NONE',  ( -2.257144641399999941E-12, 0.000000000000000000, -1.000000000000000000 ) ) ;
#13438=EDGE_CURVE ( 'NONE', #10143, #3905, #4129, .T. ) ;
#13441=CARTESIAN_POINT ( 'NONE',  ( 6.010856941112696639, -0.8786408349372250015, -150.0552959529999839 ) ) ;
#13446=CARTESIAN_POINT ( 'NONE',  ( 31.49999999989999822, 32.96379895120000469, -136.0552959530000123 ) ) ;
#13448=EDGE_CURVE ( 'NONE', #3522, #1160, #17182, .T. ) ;
#13449=CARTESIAN_POINT ( 'NONE',  ( -14.08011361694696539, -41.79914019397068614, -150.0552959529999839 ) ) ;
#13450=LINE ( 'NONE', #13564, #20588 ) ;
#13454=EDGE_CURVE ( 'NONE', #17813, #14322, #18802, .T. ) ;
#13460=DIRECTION ( 'NONE',  ( 0.000000000000000000, 1.000000000000000000, 0.000000000000000000 ) ) ;
#13461=ORIENTED_EDGE ( 'NONE', *, *, #1180, .T. ) ;
#13477=ORIENTED_EDGE ( 'NONE', *, *, #12296, .F. ) ;
#13484=DIRECTION ( 'NONE',  ( -1.000000000000000000, 0.000000000000000000, 0.000000000000000000 ) ) ;
#13485=CARTESIAN_POINT ( 'NONE',  ( 32.50000000000000000, -21.03620104879999886, -136.0552959530000123 ) ) ;
#13487=PLANE ( 'NONE',  #21672 ) ;
#13494=DIRECTION ( 'NONE',  ( 2.257252162960000001E-12, 0.000000000000000000, 1.000000000000000000 ) ) ;
#13496=CARTESIAN_POINT ( 'NONE',  ( 3.299235031439282650, -4.419791545611266415, -150.0552959529999555 ) ) ;
#13500=EDGE_LOOP ( 'NONE', ( #11637, #10385, #10558, #16101 ) ) ;
#13503=AXIS2_PLACEMENT_3D ( 'NONE', #8601, #11942, #6597 ) ;
#13512=LINE ( 'NONE', #15542, #10991 ) ;
#13516=LINE ( 'NONE', #20440, #7615 ) ;
#13520=LINE ( 'NONE', #20793, #23522 ) ;
#13524=CARTESIAN_POINT ( 'NONE',  ( 25.11919234682703461, 34.98537695657089586, -150.0552959529999839 ) ) ;
#13528=CARTESIAN_POINT ( 'NONE',  ( 23.50000000000000000, -20.50000000000000000, -137.0552959530000123 ) ) ;
#13531=EDGE_CURVE ( 'NONE', #5806, #21392, #22919, .T. ) ;
#13535=CARTESIAN_POINT ( 'NONE',  ( 23.89269908169873702, -23.49999999999999645, -150.0552959529999839 ) ) ;
#13536=VERTEX_POINT ( 'NONE', #17445 ) ;
#13541=EDGE_LOOP ( 'NONE', ( #17338, #1553, #14675, #4497 ) ) ;
#13543=ORIENTED_EDGE ( 'NONE', *, *, #5693, .T. ) ;
#13555=VERTEX_POINT ( 'NONE', #19483 ) ;
#13556=FACE_OUTER_BOUND ( 'NONE', #1840, .T. ) ;
#13557=CARTESIAN_POINT ( 'NONE',  ( -12.50000000000000000, 19.50000000000000000, -150.5552959529999839 ) ) ;
#13560=ORIENTED_EDGE ( 'NONE', *, *, #18092, .F. ) ;
#13563=CARTESIAN_POINT ( 'NONE',  ( 31.50000000000000000, 20.96379895120000114, -137.0552959530000123 ) ) ;
#13564=CARTESIAN_POINT ( 'NONE',  ( 0.000000000000000000, 47.50000000000000000, -150.0552959529999839 ) ) ;
#13565=LINE ( 'NONE', #8450, #7539 ) ;
#13572=LINE ( 'NONE', #19058, #20240 ) ;
#13579=EDGE_LOOP ( 'NONE', ( #14145, #11415, #12544, #17928 ) ) ;
#13584=DIRECTION ( 'NONE',  ( -1.000000000000000000, 0.000000000000000000, 0.000000000000000000 ) ) ;
#13587=EDGE_CURVE ( 'NONE', #3235, #4355, #14238, .T. ) ;
#13592=CARTESIAN_POINT ( 'NONE',  ( 31.50000000000000000, 32.96379895120000469, -143.0552959529999839 ) ) ;
#13596=CARTESIAN_POINT ( 'NONE',  ( 8.750000000000000000, -38.23606797749999942, -150.0552959529999839 ) ) ;
#13599=( LENGTH_UNIT ( ) NAMED_UNIT ( * ) SI_UNIT ( .MILLI., .METRE. ) );
#13603=DIRECTION ( 'NONE',  ( 1.000000000000000000, 0.000000000000000000, 0.000000000000000000 ) ) ;
#13616=EDGE_CURVE ( 'NONE', #9607, #1863, #16808, .T. ) ;
#13621=AXIS2_PLACEMENT_3D ( 'NONE', #8909, #18788, #6057 ) ;
#13623=DIRECTION ( 'NONE',  ( 1.000000000000000000, 0.000000000000000000, 0.000000000000000000 ) ) ;
#13624=AXIS2_PLACEMENT_3D ( 'NONE', #1970, #11203, #5748 ) ;
#13631=DIRECTION ( 'NONE',  ( 0.000000000000000000, 2.256988247090000272E-12, 1.000000000000000000 ) ) ;
#13632=ORIENTED_EDGE ( 'NONE', *, *, #18857, .T. ) ;
#13634=CARTESIAN_POINT ( 'NONE',  ( 31.96891336339999867, -40.94938100019999894, -150.0552959529999839 ) ) ;
#13636=DIRECTION ( 'NONE',  ( 2.257144641399999941E-12, 0.000000000000000000, 1.000000000000000000 ) ) ;
#13639=VECTOR ( 'NONE', #21945, 1000.000000000000000 ) ;
#13640=EDGE_CURVE ( 'NONE', #4521, #844, #18824, .T. ) ;
#13644=CARTESIAN_POINT ( 'NONE',  ( 6.500000000000000000, 28.00000000000000000, -150.5552959529999839 ) ) ;
#13646=AXIS2_PLACEMENT_3D ( 'NONE', #4508, #11517, #6182 ) ;
#13648=VECTOR ( 'NONE', #15283, 1000.000000000000000 ) ;
#13649=CARTESIAN_POINT ( 'NONE',  ( 24.90181682661750173, 34.66060904161302147, -150.0552959529999839 ) ) ;
#13650=VERTEX_POINT ( 'NONE', #20729 ) ;
#13655=AXIS2_PLACEMENT_3D ( 'NONE', #169, #282, #5629 ) ;
#13661=VECTOR ( 'NONE', #4405, 1000.000000000000000 ) ;
#13669=CARTESIAN_POINT ( 'NONE',  ( -2.500000000000000000, 40.00000000000000000, -150.5552959529999839 ) ) ;
#13676=DIRECTION ( 'NONE',  ( 0.000000000000000000, 0.000000000000000000, 1.000000000000000000 ) ) ;
#13684=FACE_OUTER_BOUND ( 'NONE', #13210, .T. ) ;
#13695=ORIENTED_EDGE ( 'NONE', *, *, #4090, .T. ) ;
#13706=CARTESIAN_POINT ( 'NONE',  ( 4.301424340778726929, -1.999932770097490042, -150.0552959529999839 ) ) ;
#13708=ORIENTED_EDGE ( 'NONE', *, *, #22327, .T. ) ;
#13711=CARTESIAN_POINT ( 'NONE',  ( -5.500000000000000000, 44.50000000000000000, -151.0552959529999839 ) ) ;
#13718=DIRECTION ( 'NONE',  ( -2.023844055306273103E-15, -1.000000000000000000, 0.000000000000000000 ) ) ;
#13722=CIRCLE ( 'NONE', #14478, 2.000000000000000000 ) ;
#13723=CARTESIAN_POINT ( 'NONE',  ( 7.053444247323598759, -32.99994780906266811, -150.0552959530000123 ) ) ;
#13725=DIRECTION ( 'NONE',  ( 0.000000000000000000, 0.000000000000000000, -1.000000000000000000 ) ) ;
#13740=VECTOR ( 'NONE', #2273, 1000.000000000000000 ) ;
#13743=CARTESIAN_POINT ( 'NONE',  ( -14.60730091830128252, -40.00000000000000711, -150.0552959530000123 ) ) ;
#13745=DIRECTION ( 'NONE',  ( 0.000000000000000000, -1.000000000000000000, 0.000000000000000000 ) ) ;
#13749=ADVANCED_FACE ( 'NONE', ( #11312, #22282, #15137, #7754, #20623, #5973, #13225, #18721, #2429, #9646, #6099, #5020 ), #19540, .T. ) ;
#13751=ORIENTED_EDGE ( 'NONE', *, *, #7911, .F. ) ;
#13754=AXIS2_PLACEMENT_3D ( 'NONE', #22654, #6349, #13603 ) ;
#13758=( NAMED_UNIT ( * ) PLANE_ANGLE_UNIT ( ) SI_UNIT ( $, .RADIAN. ) );
#13762=ADVANCED_FACE ( 'NONE', ( #8338 ), #3007, .T. ) ;
#13765=VERTEX_POINT ( 'NONE', #12264 ) ;
#13768=CARTESIAN_POINT ( 'NONE',  ( -31.00000000000000000, -36.00000000000000000, -149.5552959529999839 ) ) ;
#13779=LINE ( 'NONE', #19237, #4911 ) ;
#13782=DIRECTION ( 'NONE',  ( -0.7633862853691523176, 0.6459422414661291079, 0.000000000000000000 ) ) ;
#13802=DIRECTION ( 'NONE',  ( 2.257144641399999941E-12, 0.000000000000000000, -1.000000000000000000 ) ) ;
#13805=DIRECTION ( 'NONE',  ( 0.000000000000000000, -2.252420472359999842E-12, -1.000000000000000000 ) ) ;
#13814=CARTESIAN_POINT ( 'NONE',  ( 32.50000000000000000, 20.96379895120000114, -136.5552959530000123 ) ) ;
#13816=CARTESIAN_POINT ( 'NONE',  ( 21.10099947280545507, -18.65635984007526105, -150.0552959529999839 ) ) ;
#13817=CARTESIAN_POINT ( 'NONE',  ( -16.46189020600415631, -42.60961311590466494, -150.0552959530000408 ) ) ;
#13824=CARTESIAN_POINT ( 'NONE',  ( 6.500000000000000000, 20.50000000000000000, -151.0552959529999839 ) ) ;
#13826=FACE_OUTER_BOUND ( 'NONE', #5860, .T. ) ;
#13830=CARTESIAN_POINT ( 'NONE',  ( 6.000000000000000000, -3.500000000000000000, -150.0552959529999839 ) ) ;
#13831=ORIENTED_EDGE ( 'NONE', *, *, #7235, .F. ) ;
#13834=LINE ( 'NONE', #21097, #8313 ) ;
#13835=ORIENTED_EDGE ( 'NONE', *, *, #15497, .T. ) ;
#13839=CARTESIAN_POINT ( 'NONE',  ( 6.750000000000000000, -36.00000000000000000, -151.0552959529999839 ) ) ;
#13841=CARTESIAN_POINT ( 'NONE',  ( -0.009371101363106103949, 24.25767361204312067, -150.0552959529999839 ) ) ;
#13842=CARTESIAN_POINT ( 'NONE',  ( 3.736991614091279335, -36.11279581097431901, -150.0552959529999839 ) ) ;
#13843=EDGE_CURVE ( 'NONE', #384, #21164, #5127, .T. ) ;
#13854=DIRECTION ( 'NONE',  ( 0.7633862853691523176, 0.6459422414661291079, 0.000000000000000000 ) ) ;
#13860=EDGE_CURVE ( 'NONE', #17719, #903, #879, .T. ) ;
#13861=CARTESIAN_POINT ( 'NONE',  ( -32.50000000000000000, -43.00000000000000000, -137.0552959530000123 ) ) ;
#13865=EDGE_LOOP ( 'NONE', ( #4514, #16989, #17802, #15806 ) ) ;
#13866=LINE ( 'NONE', #8022, #5254 ) ;
#13870=ORIENTED_EDGE ( 'NONE', *, *, #8128, .T. ) ;
#13873=CARTESIAN_POINT ( 'NONE',  ( -31.50000000000000000, -43.00000000000000000, -137.0552959530000123 ) ) ;
#13883=ORIENTED_EDGE ( 'NONE', *, *, #22820, .F. ) ;
#13888=VECTOR ( 'NONE', #18955, 1000.000000000000227 ) ;
#13894=DIRECTION ( 'NONE',  ( -1.000000000000000000, 0.000000000000000000, 2.257144641399999941E-12 ) ) ;
#13895=ORIENTED_EDGE ( 'NONE', *, *, #14733, .T. ) ;
#13897=ORIENTED_EDGE ( 'NONE', *, *, #5038, .T. ) ;
#13898=CARTESIAN_POINT ( 'NONE',  ( 0.000000000000000000, 21.50000000000000000, -150.0552959529999839 ) ) ;
#13910=DIRECTION ( 'NONE',  ( 0.000000000000000000, 1.000000000000000000, 0.000000000000000000 ) ) ;
#13917=CARTESIAN_POINT ( 'NONE',  ( 4.107300918301270976, -0.5000000000000004441, -150.0552959529999839 ) ) ;
#13924=FACE_OUTER_BOUND ( 'NONE', #13541, .T. ) ;
#13930=CARTESIAN_POINT ( 'NONE',  ( 15.50000000000000000, 39.50000000000000000, -150.5552959529999839 ) ) ;
#13932=CARTESIAN_POINT ( 'NONE',  ( -31.00000000000000000, -50.50000000000000000, -149.5552959529999839 ) ) ;
#13934=PLANE ( 'NONE',  #8131 ) ;
#13938=VECTOR ( 'NONE', #9360, 1000.000000000000000 ) ;
#13941=ADVANCED_FACE ( 'NONE', ( #19776 ), #20126, .F. ) ;
#13949=ORIENTED_EDGE ( 'NONE', *, *, #21861, .T. ) ;
#13951=CARTESIAN_POINT ( 'NONE',  ( 6.007013984441634591, 28.00000000000000000, -150.0552959529999839 ) ) ;
#13953=DIRECTION ( 'NONE',  ( 0.000000000000000000, 1.000000000000000000, -2.273736754430000208E-12 ) ) ;
#13968=DIRECTION ( 'NONE',  ( 1.000000000000000000, 0.000000000000000000, -2.257453483404482811E-12 ) ) ;
#13974=LINE ( 'NONE', #7069, #17857 ) ;
#13977=DIRECTION ( 'NONE',  ( 0.000000000000000000, 1.000000000000000000, -2.273736754430000208E-12 ) ) ;
#13978=DIRECTION ( 'NONE',  ( -0.000000000000000000, 1.000000000000000000, 0.000000000000000000 ) ) ;
#13985=EDGE_LOOP ( 'NONE', ( #2465, #4082, #5642, #5929 ) ) ;
#13988=ORIENTED_EDGE ( 'NONE', *, *, #9522, .F. ) ;
#13990=FACE_OUTER_BOUND ( 'NONE', #1803, .T. ) ;
#14009=CARTESIAN_POINT ( 'NONE',  ( 7.750000000000000000, -42.23606797749999942, -150.5552959529999839 ) ) ;
#14015=CARTESIAN_POINT ( 'NONE',  ( -32.50000000000000000, 51.50000000000000000, -137.0552959530000123 ) ) ;
#14023=AXIS2_PLACEMENT_3D ( 'NONE', #19899, #14300, #5251 ) ;
#14030=CARTESIAN_POINT ( 'NONE',  ( 19.77963439019999825, 51.26338628519999929, -143.0552959529999839 ) ) ;
#14033=CARTESIAN_POINT ( 'NONE',  ( -32.50000000000000000, 16.00000000000000000, -144.0552959529999839 ) ) ;
#14035=CARTESIAN_POINT ( 'NONE',  ( -25.86630785139999844, -51.50000000000000000, -134.7421712960000377 ) ) ;
#14039=CARTESIAN_POINT ( 'NONE',  ( -12.50000000000000000, 25.50000000000000000, -150.0552959529999839 ) ) ;
#14041=CARTESIAN_POINT ( 'NONE',  ( -15.50000000000000000, 21.50000000000000000, -151.0552959529999839 ) ) ;
#14050=VECTOR ( 'NONE', #16082, 1000.000000000000000 ) ;
#14060=VERTEX_POINT ( 'NONE', #4053 ) ;
#14066=VECTOR ( 'NONE', #8506, 1000.000000000000000 ) ;
#14073=DIRECTION ( 'NONE',  ( 0.000000000000000000, 1.000000000000000000, 0.000000000000000000 ) ) ;
#14077=CARTESIAN_POINT ( 'NONE',  ( -0.7601318171633636434, 22.44600007524262963, -150.0552959530000123 ) ) ;
#14080=EDGE_LOOP ( 'NONE', ( #21853, #16753, #13988, #20473 ) ) ;
#14093=ORIENTED_EDGE ( 'NONE', *, *, #20168, .F. ) ;
#14104=ORIENTED_EDGE ( 'NONE', *, *, #12420, .F. ) ;
#14106=EDGE_CURVE ( 'NONE', #20428, #14361, #3941, .T. ) ;
#14107=VERTEX_POINT ( 'NONE', #9855 ) ;
#14111=DIRECTION ( 'NONE',  ( 0.000000000000000000, 1.000000000000000000, 0.000000000000000000 ) ) ;
#14126=EDGE_CURVE ( 'NONE', #4350, #9123, #20703, .T. ) ;
#14128=CARTESIAN_POINT ( 'NONE',  ( -32.50000000000000000, 50.00000000000000000, -151.0552959529999839 ) ) ;
#14130=ORIENTED_EDGE ( 'NONE', *, *, #19590, .F. ) ;
#14134=ORIENTED_EDGE ( 'NONE', *, *, #2979, .T. ) ;
#14136=DIRECTION ( 'NONE',  ( 0.000000000000000000, 1.000000000000000000, 0.000000000000000000 ) ) ;
#14139=PLANE ( 'NONE',  #12234 ) ;
#14143=CARTESIAN_POINT ( 'NONE',  ( -4.020805332102288077, 42.55092418646378860, -150.0552959530000123 ) ) ;
#14145=ORIENTED_EDGE ( 'NONE', *, *, #8148, .T. ) ;
#14147=ORIENTED_EDGE ( 'NONE', *, *, #2143, .F. ) ;
#14154=DIRECTION ( 'NONE',  ( 1.457985068979999943E-12, 1.723073263340000007E-12, -1.000000000000000000 ) ) ;
#14175=CARTESIAN_POINT ( 'NONE',  ( 26.50000000000000000, -20.50000000000000000, -150.0552959529999839 ) ) ;
#14181=PLANE ( 'NONE',  #13228 ) ;
#14183=CARTESIAN_POINT ( 'NONE',  ( -0.7500000000009999779, -50.00000000000000000, -149.5552959529999839 ) ) ;
#14184=EDGE_LOOP ( 'NONE', ( #6161, #18175, #5394, #17398 ) ) ;
#14186=EDGE_CURVE ( 'NONE', #258, #350, #16894, .T. ) ;
#14189=CYLINDRICAL_SURFACE ( 'NONE', #8232, 1.500000000000001332 ) ;
#14198=ORIENTED_EDGE ( 'NONE', *, *, #21706, .T. ) ;
#14211=CARTESIAN_POINT ( 'NONE',  ( 20.50000000000000000, 19.50000000000000000, -150.5552959529999839 ) ) ;
#14212=CARTESIAN_POINT ( 'NONE',  ( 20.50000000000000000, 19.50000000000000000, -150.0552959529999839 ) ) ;
#14213=DIRECTION ( 'NONE',  ( 1.000000000000000000, 0.000000000000000000, -2.257144641399999941E-12 ) ) ;
#14225=CARTESIAN_POINT ( 'NONE',  ( 6.500000000000000000, 20.50000000000000000, -150.0552959529999839 ) ) ;
#14229=ORIENTED_EDGE ( 'NONE', *, *, #6146, .T. ) ;
#14233=LINE ( 'NONE', #15342, #14847 ) ;
#14238=LINE ( 'NONE', #16021, #15696 ) ;
#14240=EDGE_LOOP ( 'NONE', ( #11161, #15060 ) ) ;
#14253=ORIENTED_EDGE ( 'NONE', *, *, #19463, .F. ) ;
#14266=ORIENTED_EDGE ( 'NONE', *, *, #9640, .F. ) ;
#14267=CARTESIAN_POINT ( 'NONE',  ( -2.489991676560021627, 46.24652334969350420, -150.0552959530000408 ) ) ;
#14270=EDGE_CURVE ( 'NONE', #21310, #322, #15583, .T. ) ;
#14278=DIRECTION ( 'NONE',  ( 0.000000000000000000, -1.000000000000000000, 0.000000000000000000 ) ) ;
#14280=DIRECTION ( 'NONE',  ( 0.000000000000000000, -1.000000000000000000, 0.000000000000000000 ) ) ;
#14282=DIRECTION ( 'NONE',  ( 0.000000000000000000, -1.000000000000000000, 0.000000000000000000 ) ) ;
#14283=AXIS2_PLACEMENT_3D ( 'NONE', #18671, #7823, #9485 ) ;
#14284=AXIS2_PLACEMENT_3D ( 'NONE', #15524, #13745, #2345 ) ;
#14287=CARTESIAN_POINT ( 'NONE',  ( 25.50000000000000000, 19.50000000000000000, -150.5552959529999839 ) ) ;
#14288=PLANE ( 'NONE',  #4908 ) ;
#14291=CARTESIAN_POINT ( 'NONE',  ( 19.04211518520000013, 51.50000000000000000, -149.5552959529999839 ) ) ;
#14300=DIRECTION ( 'NONE',  ( 0.000000000000000000, 0.000000000000000000, 1.000000000000000000 ) ) ;
#14304=ORIENTED_EDGE ( 'NONE', *, *, #18111, .T. ) ;
#14309=EDGE_CURVE ( 'NONE', #22853, #12372, #6648, .T. ) ;
#14312=ORIENTED_EDGE ( 'NONE', *, *, #21099, .F. ) ;
#14313=AXIS2_PLACEMENT_3D ( 'NONE', #7312, #18375, #2087 ) ;
#14315=CARTESIAN_POINT ( 'NONE',  ( 31.64594224149999846, -40.56768785850000825, -149.5552959529999839 ) ) ;
#14321=ADVANCED_FACE ( 'NONE', ( #8540 ), #11881, .T. ) ;
#14322=VERTEX_POINT ( 'NONE', #15703 ) ;
#14329=AXIS2_PLACEMENT_3D ( 'NONE', #4236, #556, #22091 ) ;
#14331=VECTOR ( 'NONE', #9743, 1000.000000000000000 ) ;
#14335=DIRECTION ( 'NONE',  ( 0.000000000000000000, 1.000000000000000000, 0.000000000000000000 ) ) ;
#14337=EDGE_LOOP ( 'NONE', ( #1434, #6539, #3143, #2333, #14134, #9344, #11840, #14304, #11929, #3965, #20827, #6168, #12976, #8182, #11572 ) ) ;
#14341=FACE_OUTER_BOUND ( 'NONE', #1164, .T. ) ;
#14346=ORIENTED_EDGE ( 'NONE', *, *, #8827, .T. ) ;
#14347=CARTESIAN_POINT ( 'NONE',  ( -5.098183173407200286, 20.66060904161428269, -150.0552959529999839 ) ) ;
#14355=ADVANCED_FACE ( 'NONE', ( #18312 ), #21778, .T. ) ;
#14361=VERTEX_POINT ( 'NONE', #10790 ) ;
#14364=VECTOR ( 'NONE', #11648, 1000.000000000000000 ) ;
#14367=DIRECTION ( 'NONE',  ( 0.000000000000000000, 1.000000000000000000, 0.000000000000000000 ) ) ;
#14371=DIRECTION ( 'NONE',  ( -1.000000000000000000, 0.000000000000000000, 0.000000000000000000 ) ) ;
#14372=PLANE ( 'NONE',  #20919 ) ;
#14375=EDGE_CURVE ( 'NONE', #16830, #12039, #120, .T. ) ;
#14378=ADVANCED_FACE ( 'NONE', ( #7360 ), #21417, .T. ) ;
#14380=ORIENTED_EDGE ( 'NONE', *, *, #7416, .T. ) ;
#14383=CIRCLE ( 'NONE', #19322, 1.500000000000001332 ) ;
#14385=ORIENTED_EDGE ( 'NONE', *, *, #10838, .F. ) ;
#14393=ORIENTED_EDGE ( 'NONE', *, *, #2786, .T. ) ;
#14401=AXIS2_PLACEMENT_3D ( 'NONE', #8500, #21932, #3721 ) ;
#14408=AXIS2_PLACEMENT_3D ( 'NONE', #15931, #23196, #11755 ) ;
#14411=EDGE_CURVE ( 'NONE', #19876, #6873, #6883, .T. ) ;
#14416=ORIENTED_EDGE ( 'NONE', *, *, #1639, .T. ) ;
#14419=ORIENTED_EDGE ( 'NONE', *, *, #11641, .T. ) ;
#14422=DIRECTION ( 'NONE',  ( -1.000000000000000000, 0.000000000000000000, 0.000000000000000000 ) ) ;
#14431=LINE ( 'NONE', #17757, #2720 ) ;
#14445=CARTESIAN_POINT ( 'NONE',  ( -2.500000000000000000, 34.00000000000000000, -150.5552959529999839 ) ) ;
#14446=VERTEX_POINT ( 'NONE', #1786 ) ;
#14447=LINE ( 'NONE', #19569, #22434 ) ;
#14451=DIRECTION ( 'NONE',  ( 0.000000000000000000, 0.000000000000000000, 1.000000000000000000 ) ) ;
#14453=PLANE ( 'NONE',  #18830 ) ;
#14462=ORIENTED_EDGE ( 'NONE', *, *, #10734, .F. ) ;
#14468=ORIENTED_EDGE ( 'NONE', *, *, #7235, .T. ) ;
#14472=CARTESIAN_POINT ( 'NONE',  ( -4.880807653193565798, 20.98537695657093138, -150.0552959529999839 ) ) ;
#14477=ORIENTED_EDGE ( 'NONE', *, *, #770, .F. ) ;
#14478=AXIS2_PLACEMENT_3D ( 'NONE', #12171, #13725, #15633 ) ;
#14483=EDGE_CURVE ( 'NONE', #11594, #10244, #10554, .T. ) ;
#14489=DIRECTION ( 'NONE',  ( -0.000000000000000000, 1.000000000000000000, 0.000000000000000000 ) ) ;
#14492=AXIS2_PLACEMENT_3D ( 'NONE', #21399, #21635, #1300 ) ;
#14493=FACE_OUTER_BOUND ( 'NONE', #20646, .T. ) ;
#14495=EDGE_CURVE ( 'NONE', #13536, #1424, #11148, .T. ) ;
#14497=CARTESIAN_POINT ( 'NONE',  ( 25.50000000000000000, 19.50000000000000000, -151.0552959529999839 ) ) ;
#14498=ORIENTED_EDGE ( 'NONE', *, *, #10349, .T. ) ;
#14500=EDGE_CURVE ( 'NONE', #6268, #4735, #11255, .T. ) ;
#14501=DIRECTION ( 'NONE',  ( -0.6459422414661291079, 0.7633862853691523176, -2.273736754430455399E-12 ) ) ;
#14511=DIRECTION ( 'NONE',  ( 0.7633862853691523176, 0.6459422414661291079, 0.000000000000000000 ) ) ;
#14518=CARTESIAN_POINT ( 'NONE',  ( 25.96278831570000278, -46.03148680980000051, -150.0552959529999839 ) ) ;
#14520=ADVANCED_FACE ( 'NONE', ( #575 ), #336, .F. ) ;
#14525=LINE ( 'NONE', #16067, #18091 ) ;
#14526=LINE ( 'NONE', #5586, #3448 ) ;
#14528=CARTESIAN_POINT ( 'NONE',  ( 32.50000000000000000, 40.03620104880000241, -143.0552959529999839 ) ) ;
#14534=DIRECTION ( 'NONE',  ( 0.000000000000000000, 1.000000000000000000, 0.000000000000000000 ) ) ;
#14539=VERTEX_POINT ( 'NONE', #4257 ) ;
#14541=CARTESIAN_POINT ( 'NONE',  ( -13.86630785140000022, -51.00000000000000000, -136.0552959530000123 ) ) ;
#14547=DIRECTION ( 'NONE',  ( 0.000000000000000000, -1.000000000000000000, 0.000000000000000000 ) ) ;
#14558=DIRECTION ( 'NONE',  ( 1.000000000000000000, 0.000000000000000000, 0.000000000000000000 ) ) ;
#14566=DIRECTION ( 'NONE',  ( -1.000000000000000000, 0.000000000000000000, 0.000000000000000000 ) ) ;
#14568=LINE ( 'NONE', #14211, #22829 ) ;
#14570=CARTESIAN_POINT ( 'NONE',  ( -15.91988638306137815, -44.20085980601010789, -150.0552959529999839 ) ) ;
#14572=EDGE_CURVE ( 'NONE', #20428, #14060, #18769, .T. ) ;
#14574=CARTESIAN_POINT ( 'NONE',  ( 15.10199673422965816, 39.50000000000000000, -150.0552959529999839 ) ) ;
#14587=EDGE_LOOP ( 'NONE', ( #18866, #6021, #17772, #17060 ) ) ;
#14588=CARTESIAN_POINT ( 'NONE',  ( -4.881030538584610667, 24.01480899504991484, -150.0552959529999839 ) ) ;
#14596=LINE ( 'NONE', #13038, #11974 ) ;
#14616=DIRECTION ( 'NONE',  ( 0.000000000000000000, -1.000000000000000000, 0.000000000000000000 ) ) ;
#14617=PLANE ( 'NONE',  #14848 ) ;
#14618=EDGE_CURVE ( 'NONE', #15247, #4592, #20920, .T. ) ;
#14620=EDGE_LOOP ( 'NONE', ( #22219, #734, #19627, #2771 ) ) ;
#14624=CARTESIAN_POINT ( 'NONE',  ( 13.13369214859999978, 50.99999999970000175, -136.0552959530000123 ) ) ;
#14631=ORIENTED_EDGE ( 'NONE', *, *, #17675, .T. ) ;
#14632=CARTESIAN_POINT ( 'NONE',  ( 18.95053822279999878, -50.00000000000000000, -151.0552959529999839 ) ) ;
#14637=CARTESIAN_POINT ( 'NONE',  ( -31.00000000000000000, 1.000000000000000000, -149.5552959529999839 ) ) ;
#14639=EDGE_CURVE ( 'NONE', #968, #20332, #2205, .T. ) ;
#14642=CARTESIAN_POINT ( 'NONE',  ( -4.500000000000000000, 40.00000000000000000, -150.0552959529999839 ) ) ;
#14649=EDGE_CURVE ( 'NONE', #4401, #20657, #18489, .T. ) ;
#14651=VERTEX_POINT ( 'NONE', #13367 ) ;
#14656=FACE_OUTER_BOUND ( 'NONE', #19160, .T. ) ;
#14658=ORIENTED_EDGE ( 'NONE', *, *, #22090, .F. ) ;
#14662=LINE ( 'NONE', #22045, #5628 ) ;
#14665=CARTESIAN_POINT ( 'NONE',  ( 25.31684607440000079, 45.26810052429999587, -149.5552959529999839 ) ) ;
#14666=CARTESIAN_POINT ( 'NONE',  ( 19.16617820230000291, 49.81753540199999719, -149.5552959529999839 ) ) ;
#14667=PLANE ( 'NONE',  #5012 ) ;
#14673=AXIS2_PLACEMENT_3D ( 'NONE', #10224, #17496, #22975 ) ;
#14675=ORIENTED_EDGE ( 'NONE', *, *, #9948, .F. ) ;
#14683=CARTESIAN_POINT ( 'NONE',  ( -3.500000000000000000, 42.50000000000000000, -151.0552959529999839 ) ) ;
#14684=CARTESIAN_POINT ( 'NONE',  ( -32.50000000000000000, -43.00000000050000182, -137.0552959530000123 ) ) ;
#14687=PRODUCT_DEFINITION_CONTEXT ( 'detailed design', #21353, 'design' ) ;
#14692=CARTESIAN_POINT ( 'NONE',  ( -31.50000000000000000, -36.00000000000000000, -143.3052959529999839 ) ) ;
#14703=AXIS2_PLACEMENT_3D ( 'NONE', #14518, #3101, #4997 ) ;
#14708=ORIENTED_EDGE ( 'NONE', *, *, #354, .T. ) ;
#14709=CARTESIAN_POINT ( 'NONE',  ( 31.00000000000000000, -39.80430157320000006, -150.5552959529999839 ) ) ;
#14710=VECTOR ( 'NONE', #13782, 1000.000000000000227 ) ;
#14720=ORIENTED_EDGE ( 'NONE', *, *, #11423, .F. ) ;
#14722=CARTESIAN_POINT ( 'NONE',  ( -32.50000000000000000, 21.50000000000000000, -151.0552959529999839 ) ) ;
#14723=CARTESIAN_POINT ( 'NONE',  ( 7.480639893028359744, 27.95196862336024779, -150.0552959529999839 ) ) ;
#14729=DIRECTION ( 'NONE',  ( 0.000000000000000000, -2.256894259950000208E-12, 1.000000000000000000 ) ) ;
#14732=DIRECTION ( 'NONE',  ( 1.000000000000000000, 0.000000000000000000, 0.000000000000000000 ) ) ;
#14733=EDGE_CURVE ( 'NONE', #19891, #7656, #6569, .T. ) ;
#14737=CYLINDRICAL_SURFACE ( 'NONE', #3623, 0.5000000000000079936 ) ;
#14743=EDGE_CURVE ( 'NONE', #13536, #13650, #2891, .T. ) ;
#14747=CARTESIAN_POINT ( 'NONE',  ( -5.499999999999999112, 44.76520911280726267, -150.0552959530000123 ) ) ;
#14751=EDGE_CURVE ( 'NONE', #15247, #18803, #5295, .T. ) ;
#14762=ADVANCED_FACE ( 'NONE', ( #15492 ), #10122, .F. ) ;
#14766=CARTESIAN_POINT ( 'NONE',  ( -32.50000000000000000, 47.50000000000000000, -151.0552959529999839 ) ) ;
#14768=VECTOR ( 'NONE', #2024, 1000.000000000000000 ) ;
#14770=CIRCLE ( 'NONE', #17038, 1.500000000000001332 ) ;
#14772=LINE ( 'NONE', #12982, #15941 ) ;
#14773=VERTEX_POINT ( 'NONE', #14858 ) ;
#14777=EDGE_CURVE ( 'NONE', #4867, #10143, #18598, .T. ) ;
#14790=ORIENTED_EDGE ( 'NONE', *, *, #17932, .T. ) ;
#14792=B_SPLINE_CURVE_WITH_KNOTS ( 'NONE', 1,
 ( #188, #17181 ),
 .UNSPECIFIED., .F., .F.,
 ( 2, 2 ),
 ( -15.50174796760000007, 0.2824781943659999683 ),
 .UNSPECIFIED. ) ;
#14793=VECTOR ( 'NONE', #16091, 1000.000000000000000 ) ;
#14798=DIRECTION ( 'NONE',  ( -2.257144641399999941E-12, 0.000000000000000000, -1.000000000000000000 ) ) ;
#14800=CYLINDRICAL_SURFACE ( 'NONE', #22755, 2.000000000000001776 ) ;
#14801=ORIENTED_EDGE ( 'NONE', *, *, #4844, .F. ) ;
#14804=CARTESIAN_POINT ( 'NONE',  ( 19.27350934360000068, 50.38169314270000143, -143.0552959529999839 ) ) ;
#14805=FACE_OUTER_BOUND ( 'NONE', #11444, .T. ) ;
#14806=CARTESIAN_POINT ( 'NONE',  ( 0.000000000000000000, 34.00000000000000000, -150.0552959529999839 ) ) ;
#14808=DIRECTION ( 'NONE',  ( 0.000000000000000000, 1.000000000000000000, 0.000000000000000000 ) ) ;
#14825=CARTESIAN_POINT ( 'NONE',  ( -31.00000000000000000, -50.00000000000000000, -149.5552959529999839 ) ) ;
#14828=VECTOR ( 'NONE', #8713, 1000.000000000000000 ) ;
#14831=VECTOR ( 'NONE', #9543, 1000.000000000000227 ) ;
#14836=ORIENTED_EDGE ( 'NONE', *, *, #15352, .T. ) ;
#14837=LINE ( 'NONE', #20312, #5630 ) ;
#14844=CARTESIAN_POINT ( 'NONE',  ( -16.84364015992473540, -45.39900052719455203, -150.0552959529999839 ) ) ;
#14847=VECTOR ( 'NONE', #6403, 1000.000000000000000 ) ;
#14848=AXIS2_PLACEMENT_3D ( 'NONE', #3794, #18879, #9700 ) ;
#14852=CARTESIAN_POINT ( 'NONE',  ( 13.99999999999999822, 20.99298601556613519, -150.0552959529999839 ) ) ;
#14856=ORIENTED_EDGE ( 'NONE', *, *, #980, .T. ) ;
#14857=LINE ( 'NONE', #22114, #2245 ) ;
#14858=CARTESIAN_POINT ( 'NONE',  ( 20.50000000000000000, 19.50000000000000000, -150.0552959529999839 ) ) ;
#14860=ORIENTED_EDGE ( 'NONE', *, *, #20297, .F. ) ;
#14869=EDGE_CURVE ( 'NONE', #7407, #14322, #18318, .T. ) ;
#14870=CARTESIAN_POINT ( 'NONE',  ( 0.000000000000000000, 50.00000000000000000, -150.0552959529999839 ) ) ;
#14874=DIRECTION ( 'NONE',  ( 0.000000000000000000, -1.000000000000000000, 0.000000000000000000 ) ) ;
#14884=DIRECTION ( 'NONE',  ( 0.000000000000000000, 2.256988247090000272E-12, 1.000000000000000000 ) ) ;
#14885=CARTESIAN_POINT ( 'NONE',  ( -6.683153925719999222, -50.50000000000000000, -136.0552959530000123 ) ) ;
#14886=ORIENTED_EDGE ( 'NONE', *, *, #8351, .F. ) ;
#14887=ADVANCED_FACE ( 'NONE', ( #16869 ), #4141, .F. ) ;
#14890=CARTESIAN_POINT ( 'NONE',  ( -31.00000000000000000, -50.00000000000000000, -150.5552959529999839 ) ) ;
#14896=VECTOR ( 'NONE', #20295, 1000.000000000000000 ) ;
#14903=EDGE_CURVE ( 'NONE', #10456, #13256, #9132, .T. ) ;
#14919=EDGE_CURVE ( 'NONE', #11360, #18084, #13779, .T. ) ;
#14925=CARTESIAN_POINT ( 'NONE',  ( 4.750000000000000000, -38.23606797749999942, -150.0552959529999839 ) ) ;
#14934=ORIENTED_EDGE ( 'NONE', *, *, #4379, .F. ) ;
#14935=LINE ( 'NONE', #2452, #1904 ) ;
#14944=DIRECTION ( 'NONE',  ( 0.000000000000000000, 2.257144641399999941E-12, -1.000000000000000000 ) ) ;
#14949=CARTESIAN_POINT ( 'NONE',  ( 5.740346993226800087, -48.74619218629713657, -150.0552959529999839 ) ) ;
#14950=ORIENTED_EDGE ( 'NONE', *, *, #14500, .F. ) ;
#14954=ORIENTED_EDGE ( 'NONE', *, *, #9946, .T. ) ;
#14955=CARTESIAN_POINT ( 'NONE',  ( -17.99999999999999645, -43.39269908169872991, -150.0552959530000123 ) ) ;
#14959=CARTESIAN_POINT ( 'NONE',  ( 0.000000000000000000, -42.23606797749999942, -150.0552959529999839 ) ) ;
#14961=DIRECTION ( 'NONE',  ( 1.000000000000000000, 0.000000000000000000, 0.000000000000000000 ) ) ;
#14963=DIRECTION ( 'NONE',  ( 0.000000000000000000, 1.000000000000000000, 2.245315043809999812E-12 ) ) ;
#14974=PLANE ( 'NONE',  #13198 ) ;
#14976=VERTEX_POINT ( 'NONE', #4370 ) ;
#14979=ORIENTED_EDGE ( 'NONE', *, *, #7640, .F. ) ;
#14987=DIRECTION ( 'NONE',  ( 1.457928428160000110E-12, -1.723197716179999783E-12, -1.000000000000000000 ) ) ;
#14989=LINE ( 'NONE', #6067, #5277 ) ;
#14990=CARTESIAN_POINT ( 'NONE',  ( 4.500000000000000000, -3.500000000000000000, -140.0552959529999839 ) ) ;
#14992=EDGE_LOOP ( 'NONE', ( #3635, #21059, #12814, #10548 ) ) ;
#14994=CIRCLE ( 'NONE', #23358, 2.999999999999999112 ) ;
#15015=PLANE ( 'NONE',  #7662 ) ;
#15016=CARTESIAN_POINT ( 'NONE',  ( 8.750000000000000000, -39.23606797749999942, -150.0552959529999839 ) ) ;
#15023=VECTOR ( 'NONE', #5439, 1000.000000000000000 ) ;
#15037=ADVANCED_FACE ( 'NONE', ( #17693 ), #17809, .F. ) ;
#15045=ORIENTED_EDGE ( 'NONE', *, *, #21016, .T. ) ;
#15053=EDGE_CURVE ( 'NONE', #19299, #14651, #21159, .T. ) ;
#15056=AXIS2_PLACEMENT_3D ( 'NONE', #6717, #13978, #21249 ) ;
#15058=EDGE_CURVE ( 'NONE', #10920, #22442, #10768, .T. ) ;
#15060=ORIENTED_EDGE ( 'NONE', *, *, #16241, .T. ) ;
#15064=ADVANCED_FACE ( 'NONE', ( #1181 ), #10653, .T. ) ;
#15069=CARTESIAN_POINT ( 'NONE',  ( -12.60099947280544797, -44.84364015992472474, -150.0552959529999555 ) ) ;
#15071=EDGE_CURVE ( 'NONE', #16883, #18382, #12212, .T. ) ;
#15076=DIRECTION ( 'NONE',  ( 0.6459422414661339928, 0.7633862853691482098, 0.000000000000000000 ) ) ;
#15084=ORIENTED_EDGE ( 'NONE', *, *, #21376, .F. ) ;
#15088=DIRECTION ( 'NONE',  ( 0.000000000000000000, -2.256894259950000208E-12, 1.000000000000000000 ) ) ;
#15096=ADVANCED_FACE ( 'NONE', ( #23168 ), #8626, .F. ) ;
#15098=CARTESIAN_POINT ( 'NONE',  ( -6.683153925719999222, -50.50000000000000000, -150.0552959529999839 ) ) ;
#15102=CARTESIAN_POINT ( 'NONE',  ( -32.50000000000000000, 51.50000000000000000, -142.8052959529999839 ) ) ;
#15106=CARTESIAN_POINT ( 'NONE',  ( 32.00000000000000000, -33.03620104880000241, -136.0552959530000123 ) ) ;
#15107=VECTOR ( 'NONE', #18700, 1000.000000000000000 ) ;
#15108=EDGE_LOOP ( 'NONE', ( #20260, #5515 ) ) ;
#15111=PLANE ( 'NONE',  #1860 ) ;
#15112=ORIENTED_EDGE ( 'NONE', *, *, #2189, .T. ) ;
#15114=SHAPE_REPRESENTATION ( 'Main Base', ( #5025 ), #8794 ) ;
#15116=CARTESIAN_POINT ( 'NONE',  ( 18.95053822279999878, -50.00000000000000000, -151.0552959529999839 ) ) ;
#15124=CARTESIAN_POINT ( 'NONE',  ( -13.53835085784080761, -42.60938321240698201, -150.0552959529999839 ) ) ;
#15129=EDGE_CURVE ( 'NONE', #6192, #903, #2002, .T. ) ;
#15137=FACE_BOUND ( 'NONE', #7719, .T. ) ;
#15138=ORIENTED_EDGE ( 'NONE', *, *, #21566, .T. ) ;
#15139=CYLINDRICAL_SURFACE ( 'NONE', #11428, 0.5000000000000079936 ) ;
#15150=DIRECTION ( 'NONE',  ( 0.000000000000000000, -2.257144641399999941E-12, -1.000000000000000000 ) ) ;
#15151=CARTESIAN_POINT ( 'NONE',  ( -3.500000000000000000, 40.00000000000000000, -151.0552959529999839 ) ) ;
#15159=VECTOR ( 'NONE', #14547, 1000.000000000000000 ) ;
#15163=DIRECTION ( 'NONE',  ( 0.000000000000000000, -2.256894259950000208E-12, 1.000000000000000000 ) ) ;
#15166=VECTOR ( 'NONE', #5920, 1000.000000000000000 ) ;
#15181=VECTOR ( 'NONE', #18858, 1000.000000000000000 ) ;
#15182=VECTOR ( 'NONE', #7492, 1000.000000000000000 ) ;
#15184=ORIENTED_EDGE ( 'NONE', *, *, #5183, .T. ) ;
#15186=EDGE_CURVE ( 'NONE', #8234, #11634, #12748, .T. ) ;
#15187=ORIENTED_EDGE ( 'NONE', *, *, #12943, .F. ) ;
#15190=DIRECTION ( 'NONE',  ( 1.000000000000000000, 0.000000000000000000, 0.000000000000000000 ) ) ;
#15197=CARTESIAN_POINT ( 'NONE',  ( 25.38675467179999856, 45.20894709569999748, -149.5552959529999839 ) ) ;
#15198=FACE_OUTER_BOUND ( 'NONE', #16316, .T. ) ;
#15199=CARTESIAN_POINT ( 'NONE',  ( -32.50000000000000000, 51.50000000000000000, -149.5552959529999839 ) ) ;
#15206=EDGE_LOOP ( 'NONE', ( #17680, #15393, #20100, #8169 ) ) ;
#15210=EDGE_CURVE ( 'NONE', #802, #9566, #14596, .T. ) ;
#15216=FACE_OUTER_BOUND ( 'NONE', #8422, .T. ) ;
#15217=LINE ( 'NONE', #7820, #20202 ) ;
#15227=CARTESIAN_POINT ( 'NONE',  ( -31.50000000000000000, -50.00000000000000000, -149.5552959529999839 ) ) ;
#15240=VECTOR ( 'NONE', #1833, 1000.000000000000000 ) ;
#15242=ORIENTED_EDGE ( 'NONE', *, *, #21919, .T. ) ;
#15243=LINE ( 'NONE', #8193, #12395 ) ;
#15247=VERTEX_POINT ( 'NONE', #11012 ) ;
#15250=CARTESIAN_POINT ( 'NONE',  ( -16.20085980602537035, -42.08011361693860408, -150.0552959529999839 ) ) ;
#15253=AXIS2_PLACEMENT_3D ( 'NONE', #6011, #15856, #4918 ) ;
#15259=CARTESIAN_POINT ( 'NONE',  ( 23.50000000000000000, -20.50000000000000000, -143.5552959529999839 ) ) ;
#15268=EDGE_CURVE ( 'NONE', #4135, #19589, #2223, .T. ) ;
#15274=AXIS2_PLACEMENT_3D ( 'NONE', #7054, #7404, #7515 ) ;
#15283=DIRECTION ( 'NONE',  ( 0.000000000000000000, -1.000000000000000000, 0.000000000000000000 ) ) ;
#15287=CARTESIAN_POINT ( 'NONE',  ( 19.77963439019999825, -51.26338628519999929, -136.0552959519999945 ) ) ;
#15291=ORIENTED_EDGE ( 'NONE', *, *, #22038, .T. ) ;
#15305=ORIENTED_EDGE ( 'NONE', *, *, #20945, .T. ) ;
#15315=DIRECTION ( 'NONE',  ( 0.000000000000000000, 0.000000000000000000, 1.000000000000000000 ) ) ;
#15320=CARTESIAN_POINT ( 'NONE',  ( 31.00000000000000000, -39.80430157320000006, -151.0552959529999839 ) ) ;
#15322=EDGE_LOOP ( 'NONE', ( #7584, #11020, #21763, #11408 ) ) ;
#15327=EDGE_CURVE ( 'NONE', #7397, #7104, #6488, .T. ) ;
#15331=CARTESIAN_POINT ( 'NONE',  ( 6.500000000000000000, 28.00000000000000000, -151.0552959529999839 ) ) ;
#15332=DIRECTION ( 'NONE',  ( 0.000000000000000000, -1.000000000000000000, 0.000000000000000000 ) ) ;
#15334=CARTESIAN_POINT ( 'NONE',  ( 24.97526911139999939, 44.90215078659999648, -151.0552959529999839 ) ) ;
#15335=CARTESIAN_POINT ( 'NONE',  ( 20.87864083493722234, -22.01085694111270641, -150.0552959530000123 ) ) ;
#15340=ORIENTED_EDGE ( 'NONE', *, *, #529, .F. ) ;
#15342=CARTESIAN_POINT ( 'NONE',  ( 31.50000000000000000, 0.000000000000000000, -137.0552959530000123 ) ) ;
#15345=EDGE_CURVE ( 'NONE', #4350, #3167, #1404, .T. ) ;
#15348=CARTESIAN_POINT ( 'NONE',  ( 31.00000000000000000, 39.80430157320000006, -150.0552959529999839 ) ) ;
#15351=CARTESIAN_POINT ( 'NONE',  ( -25.86630785139999844, -50.50000000000000000, -143.0552959529999839 ) ) ;
#15352=EDGE_CURVE ( 'NONE', #20386, #22853, #602, .T. ) ;
#15356=CARTESIAN_POINT ( 'NONE',  ( 6.899000527194538712, -1.656359840075253942, -150.0552959529999839 ) ) ;
#15377=ORIENTED_EDGE ( 'NONE', *, *, #21374, .F. ) ;
#15378=CARTESIAN_POINT ( 'NONE',  ( 18.95053822279999878, -50.50000000000000000, -149.5552959529999839 ) ) ;
#15389=ORIENTED_EDGE ( 'NONE', *, *, #17375, .T. ) ;
#15391=ADVANCED_FACE ( 'NONE', ( #18859 ), #6360, .F. ) ;
#15393=ORIENTED_EDGE ( 'NONE', *, *, #3537, .F. ) ;
#15398=ORIENTED_EDGE ( 'NONE', *, *, #12164, .T. ) ;
#15401=CIRCLE ( 'NONE', #22637, 2.000000000000000000 ) ;
#15402=ORIENTED_EDGE ( 'NONE', *, *, #18049, .T. ) ;
#15410=VECTOR ( 'NONE', #10316, 1000.000000000000227 ) ;
#15412=VECTOR ( 'NONE', #3163, 1000.000000000000000 ) ;
#15429=DIRECTION ( 'NONE',  ( 0.000000000000000000, 1.000000000000000000, 2.257144641399999941E-12 ) ) ;
#15434=EDGE_LOOP ( 'NONE', ( #1027, #23312, #11060, #12724 ) ) ;
#15440=EDGE_LOOP ( 'NONE', ( #5002, #13835, #22833, #3438 ) ) ;
#15443=EDGE_LOOP ( 'NONE', ( #12294, #15540, #4063, #10348 ) ) ;
#15463=ORIENTED_EDGE ( 'NONE', *, *, #5466, .F. ) ;
#15465=EDGE_CURVE ( 'NONE', #8748, #22265, #23019, .T. ) ;
#15469=ORIENTED_EDGE ( 'NONE', *, *, #8827, .F. ) ;
#15472=CARTESIAN_POINT ( 'NONE',  ( 26.42191803000494588, -19.71475634692216161, -150.0552959530000123 ) ) ;
#15473=DIRECTION ( 'NONE',  ( -0.6459422414661291079, -0.7633862853691523176, -2.273736754430455399E-12 ) ) ;
#15474=LINE ( 'NONE', #17622, #17920 ) ;
#15477=ORIENTED_EDGE ( 'NONE', *, *, #13860, .F. ) ;
#15481=DIRECTION ( 'NONE',  ( 0.000000000000000000, 0.000000000000000000, 1.000000000000000000 ) ) ;
#15482=CARTESIAN_POINT ( 'NONE',  ( 31.00000000000000000, -39.80430157320000006, -149.5552959529999839 ) ) ;
#15491=LINE ( 'NONE', #6568, #16754 ) ;
#15492=FACE_OUTER_BOUND ( 'NONE', #563, .T. ) ;
#15494=ORIENTED_EDGE ( 'NONE', *, *, #8183, .T. ) ;
#15496=AXIS2_PLACEMENT_3D ( 'NONE', #14684, #5637, #5985 ) ;
#15497=EDGE_CURVE ( 'NONE', #21310, #16420, #12302, .T. ) ;
#15501=CARTESIAN_POINT ( 'NONE',  ( -1.000000000000000000, 20.50000000000000000, -150.0552959529999839 ) ) ;
#15504=LINE ( 'NONE', #22764, #13888 ) ;
#15506=CARTESIAN_POINT ( 'NONE',  ( 9.660841442678691493, -35.21298433615703516, -150.0552959529999839 ) ) ;
#15508=EDGE_CURVE ( 'NONE', #1217, #1116, #6833, .T. ) ;
#15518=VECTOR ( 'NONE', #6603, 1000.000000000000000 ) ;
#15519=EDGE_LOOP ( 'NONE', ( #16249, #22498, #1317, #11597 ) ) ;
#15524=CARTESIAN_POINT ( 'NONE',  ( 31.00000000000000000, -39.80430157320000006, -149.5552959529999839 ) ) ;
#15527=CARTESIAN_POINT ( 'NONE',  ( 4.890616787569204149, -4.961649142147357416, -150.0552959529999839 ) ) ;
#15529=VECTOR ( 'NONE', #9636, 1000.000000000000000 ) ;
#15534=SURFACE_STYLE_FILL_AREA ( #22324 ) ;
#15535=ORIENTED_EDGE ( 'NONE', *, *, #12869, .T. ) ;
#15540=ORIENTED_EDGE ( 'NONE', *, *, #9513, .F. ) ;
#15542=CARTESIAN_POINT ( 'NONE',  ( -12.00000000000000000, -43.00000000000000000, -145.5552959529999839 ) ) ;
#15547=CIRCLE ( 'NONE', #16322, 0.5000000000000004441 ) ;
#15555=VECTOR ( 'NONE', #1461, 1000.000000000000000 ) ;
#15556=CARTESIAN_POINT ( 'NONE',  ( 8.250000000000000000, -40.23606797749999942, -151.0552959529999839 ) ) ;
#15562=CARTESIAN_POINT ( 'NONE',  ( -6.683153925719999222, -50.50000000000000000, -149.5552959529999839 ) ) ;
#15564=ORIENTED_EDGE ( 'NONE', *, *, #17873, .F. ) ;
#15566=CARTESIAN_POINT ( 'NONE',  ( 25.01085694111271351, -23.12135916506276700, -150.0552959529999839 ) ) ;
#15569=VECTOR ( 'NONE', #17615, 1000.000000000000227 ) ;
#15571=EDGE_LOOP ( 'NONE', ( #7535, #13203, #4275, #2765 ) ) ;
#15579=PLANE ( 'NONE',  #7318 ) ;
#15583=LINE ( 'NONE', #14030, #17816 ) ;
#15586=EDGE_CURVE ( 'NONE', #22593, #20530, #4702, .T. ) ;
#15587=EDGE_CURVE ( 'NONE', #7890, #17719, #19209, .T. ) ;
#15589=VECTOR ( 'NONE', #11574, 1000.000000000000227 ) ;
#15598=CARTESIAN_POINT ( 'NONE',  ( 19.91945158500000090, 51.14507942810000429, -149.8052959529999839 ) ) ;
#15600=CARTESIAN_POINT ( 'NONE',  ( -15.75716798047311862, -41.69030790613991400, -150.0552959529999555 ) ) ;
#15604=LINE ( 'NONE', #19414, #16778 ) ;
#15605=LINE ( 'NONE', #1452, #18214 ) ;
#15607=DIRECTION ( 'NONE',  ( 0.000000000000000000, 0.000000000000000000, 1.000000000000000000 ) ) ;
#15610=EDGE_CURVE ( 'NONE', #9566, #20428, #8384, .T. ) ;
#15614=CARTESIAN_POINT ( 'NONE',  ( 3.742832019563417045, -2.190307906135578797, -150.0552959529999839 ) ) ;
#15618=DIRECTION ( 'NONE',  ( 0.000000000000000000, -1.000000000000000000, 0.000000000000000000 ) ) ;
#15620=FACE_OUTER_BOUND ( 'NONE', #1390, .T. ) ;
#15625=CARTESIAN_POINT ( 'NONE',  ( 32.50000000000000000, 39.80430157340000363, -150.0552959529999839 ) ) ;
#15628=CARTESIAN_POINT ( 'NONE',  ( 6.500000000000000000, 28.00000000000000000, -150.0552959529999839 ) ) ;
#15630=CARTESIAN_POINT ( 'NONE',  ( 3.775218130398811045, -35.50714246577857836, -150.0552959529999555 ) ) ;
#15632=ORIENTED_EDGE ( 'NONE', *, *, #3210, .T. ) ;
#15633=DIRECTION ( 'NONE',  ( 1.000000000000000000, 0.000000000000000000, 0.000000000000000000 ) ) ;
#15639=ORIENTED_EDGE ( 'NONE', *, *, #19756, .F. ) ;
#15640=CARTESIAN_POINT ( 'NONE',  ( -31.00000000000000000, -51.00000000000000000, -149.5552959529999839 ) ) ;
#15642=EDGE_CURVE ( 'NONE', #467, #23250, #10980, .T. ) ;
#15645=VECTOR ( 'NONE', #14111, 1000.000000000000000 ) ;
#15647=ADVANCED_FACE ( 'NONE', ( #7186 ), #14453, .T. ) ;
#15650=CARTESIAN_POINT ( 'NONE',  ( 31.82297112100000192, -40.41789419119999849, -136.0552959530000123 ) ) ;
#15658=LINE ( 'NONE', #19103, #21612 ) ;
#15659=AXIS2_PLACEMENT_3D ( 'NONE', #9578, #22211, #20205 ) ;
#15663=ORIENTED_EDGE ( 'NONE', *, *, #17430, .T. ) ;
#15667=CARTESIAN_POINT ( 'NONE',  ( 19.13369214879999802, -50.49999999980000354, -143.0552959529999839 ) ) ;
#15672=CARTESIAN_POINT ( 'NONE',  ( -32.50000000000000000, 10.25000000050000004, -137.0552959530000123 ) ) ;
#15682=CARTESIAN_POINT ( 'NONE',  ( 23.28059818845795803, 33.57621958799324347, -150.0552959530000123 ) ) ;
#15685=CARTESIAN_POINT ( 'NONE',  ( 25.00000000000000000, -20.50000000000000000, -136.0552959530000123 ) ) ;
#15688=CARTESIAN_POINT ( 'NONE',  ( 31.50000000000000000, -33.03620104880000241, -137.0552959530000123 ) ) ;
#15696=VECTOR ( 'NONE', #21502, 1000.000000000000000 ) ;
#15698=ORIENTED_EDGE ( 'NONE', *, *, #14751, .T. ) ;
#15699=DIRECTION ( 'NONE',  ( 0.000000000000000000, 0.000000000000000000, 1.000000000000000000 ) ) ;
#15703=CARTESIAN_POINT ( 'NONE',  ( 14.00000000000000000, 20.50000000000000000, -150.0552959529999839 ) ) ;
#15714=CARTESIAN_POINT ( 'NONE',  ( 20.50000000000000000, -20.50000000000000000, -150.0552959529999839 ) ) ;
#15715=LINE ( 'NONE', #22977, #381 ) ;
#15721=CARTESIAN_POINT ( 'NONE',  ( 25.50000000000000000, 19.50000000000000000, -150.0552959529999839 ) ) ;
#15724=EDGE_CURVE ( 'NONE', #4735, #1301, #20280, .T. ) ;
#15731=EDGE_LOOP ( 'NONE', ( #7033, #10026, #4153, #23386 ) ) ;
#15742=CARTESIAN_POINT ( 'NONE',  ( 8.920566648557704426, -33.90725470905313443, -150.0552959529999839 ) ) ;
#15754=B_SPLINE_CURVE_WITH_KNOTS ( 'NONE', 3,
 ( #3643, #12430, #18156, #16376, #10758, #21856, #14588, #7209, #23157, #6851, #21387, #14472, #14347, #1518, #5073, #12317, #19592, #3285 ),
 .UNSPECIFIED., .F., .F.,
 ( 4, 2, 2, 2, 2, 2, 2, 2, 4 ),
 ( 0.000000000000000000, 0.1250000000000000000, 0.2500000000000000000, 0.3750000000000000000, 0.5000000000000000000, 0.6250000000000000000, 0.7500000000000000000, 0.8750000000000000000, 1.000000000000000000 ),
 .UNSPECIFIED. ) ;
#15760=EDGE_CURVE ( 'NONE', #22442, #4332, #18481, .T. ) ;
#15762=LINE ( 'NONE', #15650, #22665 ) ;
#15769=EDGE_LOOP ( 'NONE', ( #9653, #18760, #9950, #13831 ) ) ;
#15770=DIRECTION ( 'NONE',  ( 0.000000000000000000, -1.000000000000000000, 1.723073263340000007E-12 ) ) ;
#15771=ADVANCED_FACE ( 'NONE', ( #18022 ), #7418, .T. ) ;
#15781=CARTESIAN_POINT ( 'NONE',  ( 31.50000000000000000, 20.96379895120000114, -143.0552959529999839 ) ) ;
#15791=VECTOR ( 'NONE', #23026, 1000.000000000000000 ) ;
#15798=LINE ( 'NONE', #23062, #8569 ) ;
#15806=ORIENTED_EDGE ( 'NONE', *, *, #3400, .F. ) ;
#15808=ORIENTED_EDGE ( 'NONE', *, *, #13438, .T. ) ;
#15811=VERTEX_POINT ( 'NONE', #8110 ) ;
#15821=DIRECTION ( 'NONE',  ( -1.000000000000000000, 0.000000000000000000, 2.245315044999999693E-12 ) ) ;
#15827=DIRECTION ( 'NONE',  ( -1.000000000000000000, 0.000000000000000000, 2.257144641399999941E-12 ) ) ;
#15828=PLANE ( 'NONE',  #19826 ) ;
#15833=CARTESIAN_POINT ( 'NONE',  ( -3.500000000000000000, 46.50000000000000000, -151.0552959529999839 ) ) ;
#15840=VERTEX_POINT ( 'NONE', #2782 ) ;
#15843=ORIENTED_EDGE ( 'NONE', *, *, #9064, .F. ) ;
#15854=AXIS2_PLACEMENT_3D ( 'NONE', #3999, #11349, #2346 ) ;
#15856=DIRECTION ( 'NONE',  ( -0.000000000000000000, 1.000000000000000000, 0.000000000000000000 ) ) ;
#15859=ORIENTED_EDGE ( 'NONE', *, *, #9190, .F. ) ;
#15862=CARTESIAN_POINT ( 'NONE',  ( -2.500000000000000000, 40.00000000000000000, -150.0552959529999839 ) ) ;
#15866=ORIENTED_EDGE ( 'NONE', *, *, #10973, .T. ) ;
#15871=FACE_OUTER_BOUND ( 'NONE', #5250, .T. ) ;
#15878=LINE ( 'NONE', #6837, #3991 ) ;
#15881=CARTESIAN_POINT ( 'NONE',  ( -32.50000000000000000, -36.00000000000000000, -150.5552959529999839 ) ) ;
#15882=UNCERTAINTY_MEASURE_WITH_UNIT (LENGTH_MEASURE( 1.000000000000000082E-05 ), #6140, 'distance_accuracy_value', 'NONE');
#15886=AXIS2_PLACEMENT_3D ( 'NONE', #12309, #12068, #15770 ) ;
#15890=ORIENTED_EDGE ( 'NONE', *, *, #23355, .T. ) ;
#15898=ORIENTED_EDGE ( 'NONE', *, *, #4992, .F. ) ;
#15910=PLANE ( 'NONE',  #18558 ) ;
#15915=VERTEX_POINT ( 'NONE', #4086 ) ;
#15919=ORIENTED_EDGE ( 'NONE', *, *, #3537, .T. ) ;
#15924=VECTOR ( 'NONE', #9037, 1000.000000000000227 ) ;
#15925=FACE_BOUND ( 'NONE', #19612, .T. ) ;
#15930=AXIS2_PLACEMENT_3D ( 'NONE', #21750, #14944, #7336 ) ;
#15931=CARTESIAN_POINT ( 'NONE',  ( 1.133692148550000001, -51.50000000000000000, -134.3952035990000127 ) ) ;
#15941=VECTOR ( 'NONE', #3951, 1000.000000000000000 ) ;
#15949=CARTESIAN_POINT ( 'NONE',  ( 7.133692148549999779, 51.50000000000000000, -137.0552959530000123 ) ) ;
#15965=EDGE_LOOP ( 'NONE', ( #23011, #18402, #22630, #6198 ) ) ;
#15969=DIRECTION ( 'NONE',  ( -0.000000000000000000, 1.000000000000000000, 0.000000000000000000 ) ) ;
#15973=CARTESIAN_POINT ( 'NONE',  ( 31.00000000000000000, -39.80430157320000006, -151.0552959529999839 ) ) ;
#15986=CARTESIAN_POINT ( 'NONE',  ( 31.50000000030000180, -40.03620104859999884, -150.0552959529999839 ) ) ;
#15987=FACE_OUTER_BOUND ( 'NONE', #18440, .T. ) ;
#15992=VERTEX_POINT ( 'NONE', #23232 ) ;
#15995=CARTESIAN_POINT ( 'NONE',  ( 18.95053822279999878, -51.50000000000000000, -149.8052959529999839 ) ) ;
#15996=CIRCLE ( 'NONE', #5733, 1.499999999999996225 ) ;
#15998=CARTESIAN_POINT ( 'NONE',  ( 26.50000000000000000, -20.50000000000000000, -137.0552959530000123 ) ) ;
#15999=COLOUR_RGB ( '', 0.40784314, 0.44705882, 0.49803922) ;
#16004=DIRECTION ( 'NONE',  ( 0.000000000000000000, 0.000000000000000000, 1.000000000000000000 ) ) ;
#16016=VECTOR ( 'NONE', #1226, 1000.000000000000000 ) ;
#16019=DIRECTION ( 'NONE',  ( 0.7633862853691523176, -0.6459422414661291079, 0.000000000000000000 ) ) ;
#16021=CARTESIAN_POINT ( 'NONE',  ( 7.133692148549999779, -51.50000000000000000, -137.0552959530000123 ) ) ;
#16027=ORIENTED_EDGE ( 'NONE', *, *, #19235, .T. ) ;
#16044=ORIENTED_EDGE ( 'NONE', *, *, #13030, .F. ) ;
#16046=ORIENTED_EDGE ( 'NONE', *, *, #4201, .T. ) ;
#16052=ADVANCED_FACE ( 'NONE', ( #19429 ), #3135, .F. ) ;
#16053=DIRECTION ( 'NONE',  ( 0.000000000000000000, 0.000000000000000000, 1.000000000000000000 ) ) ;
#16055=CARTESIAN_POINT ( 'NONE',  ( 4.750000000000000000, 0.000000000000000000, -150.0552959529999839 ) ) ;
#16056=ORIENTED_EDGE ( 'NONE', *, *, #6029, .F. ) ;
#16058=EDGE_CURVE ( 'NONE', #22265, #8748, #19217, .T. ) ;
#16063=DIRECTION ( 'NONE',  ( 0.000000000000000000, 0.000000000000000000, 1.000000000000000000 ) ) ;
#16064=ORIENTED_EDGE ( 'NONE', *, *, #17540, .F. ) ;
#16067=CARTESIAN_POINT ( 'NONE',  ( -31.00000000000000000, -43.00000000000000000, -151.0552959529999839 ) ) ;
#16071=CARTESIAN_POINT ( 'NONE',  ( -32.50000000000000000, -51.00000000000000000, -136.0552959530000123 ) ) ;
#16082=DIRECTION ( 'NONE',  ( 0.000000000000000000, 0.000000000000000000, 1.000000000000000000 ) ) ;
#16089=ORIENTED_EDGE ( 'NONE', *, *, #2786, .F. ) ;
#16091=DIRECTION ( 'NONE',  ( 0.000000000000000000, 0.000000000000000000, 1.000000000000000000 ) ) ;
#16095=ORIENTED_EDGE ( 'NONE', *, *, #4732, .F. ) ;
#16101=ORIENTED_EDGE ( 'NONE', *, *, #1029, .F. ) ;
#16112=ORIENTED_EDGE ( 'NONE', *, *, #9840, .F. ) ;
#16114=DIRECTION ( 'NONE',  ( -1.000000000000000000, 0.000000000000000000, 0.000000000000000000 ) ) ;
#16126=EDGE_CURVE ( 'NONE', #4966, #23428, #10126, .T. ) ;
#16134=DIRECTION ( 'NONE',  ( -1.000000000000000000, 0.000000000000000000, 2.257144641399999941E-12 ) ) ;
#16136=LINE ( 'NONE', #7884, #14896 ) ;
#16139=VECTOR ( 'NONE', #1697, 1000.000000000000000 ) ;
#16140=CARTESIAN_POINT ( 'NONE',  ( -3.500000000000000000, 42.50000000000000000, -150.5552959529999839 ) ) ;
#16145=CARTESIAN_POINT ( 'NONE',  ( 31.96891336220000213, 40.94938100119999547, -149.5552959529999839 ) ) ;
#16154=ORIENTED_EDGE ( 'NONE', *, *, #16494, .F. ) ;
#16158=LINE ( 'NONE', #21517, #5191 ) ;
#16161=ORIENTED_EDGE ( 'NONE', *, *, #4567, .F. ) ;
#16169=ORIENTED_EDGE ( 'NONE', *, *, #20273, .T. ) ;
#16174=VERTEX_POINT ( 'NONE', #21813 ) ;
#16175=DIRECTION ( 'NONE',  ( 0.000000000000000000, 0.000000000000000000, 1.000000000000000000 ) ) ;
#16177=VECTOR ( 'NONE', #13494, 1000.000000000000000 ) ;
#16179=FACE_OUTER_BOUND ( 'NONE', #14337, .T. ) ;
#16184=EDGE_CURVE ( 'NONE', #5292, #22593, #16551, .T. ) ;
#16185=LINE ( 'NONE', #2148, #8949 ) ;
#16197=EDGE_CURVE ( 'NONE', #802, #5378, #4044, .T. ) ;
#16206=VECTOR ( 'NONE', #3861, 1000.000000000000000 ) ;
#16210=DIRECTION ( 'NONE',  ( 1.000000000000000000, 0.000000000000000000, 0.000000000000000000 ) ) ;
#16223=AXIS2_PLACEMENT_3D ( 'NONE', #16360, #21603, #21486 ) ;
#16226=LINE ( 'NONE', #51, #8882 ) ;
#16229=PLANE ( 'NONE',  #18249 ) ;
#16235=EDGE_CURVE ( 'NONE', #5378, #12200, #2518, .T. ) ;
#16236=CARTESIAN_POINT ( 'NONE',  ( -16.50000000000000000, -43.00000000000000000, -140.0552959529999839 ) ) ;
#16238=EDGE_CURVE ( 'NONE', #11906, #3138, #6304, .T. ) ;
#16239=VECTOR ( 'NONE', #20417, 1000.000000000000000 ) ;
#16241=EDGE_CURVE ( 'NONE', #4592, #21084, #10442, .T. ) ;
#16249=ORIENTED_EDGE ( 'NONE', *, *, #11919, .F. ) ;
#16254=DIRECTION ( 'NONE',  ( -2.256967945870000144E-12, 0.000000000000000000, -1.000000000000000000 ) ) ;
#16261=DIRECTION ( 'NONE',  ( -0.7633862853691524286, 0.6459422414661293299, -2.747801985950551593E-15 ) ) ;
#16267=DIRECTION ( 'NONE',  ( 0.000000000000000000, 0.000000000000000000, 1.000000000000000000 ) ) ;
#16269=EDGE_LOOP ( 'NONE', ( #425, #2875, #14130, #12103 ) ) ;
#16270=CIRCLE ( 'NONE', #2212, 1.499999999999998446 ) ;
#16271=DIRECTION ( 'NONE',  ( 0.000000000000000000, 0.000000000000000000, 1.000000000000000000 ) ) ;
#16272=AXIS2_PLACEMENT_3D ( 'NONE', #17314, #13390, #13623 ) ;
#16273=VERTEX_POINT ( 'NONE', #5837 ) ;
#16274=LINE ( 'NONE', #14009, #1096 ) ;
#16275=LINE ( 'NONE', #8760, #17313 ) ;
#16276=EDGE_LOOP ( 'NONE', ( #15242, #7843, #18487, #21035 ) ) ;
#16281=ORIENTED_EDGE ( 'NONE', *, *, #14411, .F. ) ;
#16283=VERTEX_POINT ( 'NONE', #2170 ) ;
#16293=VECTOR ( 'NONE', #19767, 1000.000000000000000 ) ;
#16299=CARTESIAN_POINT ( 'NONE',  ( 3.000000000000000000, -3.500000000000000000, -150.0552959529999839 ) ) ;
#16301=LINE ( 'NONE', #6, #17847 ) ;
#16304=PLANE ( 'NONE',  #9705 ) ;
#16309=EDGE_LOOP ( 'NONE', ( #4245, #19345, #16112, #4902 ) ) ;
#16310=CARTESIAN_POINT ( 'NONE',  ( -31.50000000000000000, -50.00000000000000000, -137.0552959530000123 ) ) ;
#16313=DIRECTION ( 'NONE',  ( 0.000000000000000000, -2.257144641399999941E-12, 1.000000000000000000 ) ) ;
#16315=LINE ( 'NONE', #1584, #14050 ) ;
#16316=EDGE_LOOP ( 'NONE', ( #5762, #20597, #22842, #19112 ) ) ;
#16322=AXIS2_PLACEMENT_3D ( 'NONE', #11792, #995, #4675 ) ;
#16327=CARTESIAN_POINT ( 'NONE',  ( 32.50000000000000000, 39.92025131100000124, -150.0552959529999839 ) ) ;
#16329=AXIS2_PLACEMENT_3D ( 'NONE', #21395, #12562, #8871 ) ;
#16333=LINE ( 'NONE', #7284, #1814 ) ;
#16336=LINE ( 'NONE', #3361, #22866 ) ;
#16337=ORIENTED_EDGE ( 'NONE', *, *, #9256, .F. ) ;
#16338=DIRECTION ( 'NONE',  ( -1.000000000000000000, 0.000000000000000000, 0.000000000000000000 ) ) ;
#16339=EDGE_CURVE ( 'NONE', #19299, #11584, #16788, .T. ) ;
#16350=DIRECTION ( 'NONE',  ( 0.000000000000000000, 0.000000000000000000, 1.000000000000000000 ) ) ;
#16351=ADVANCED_FACE ( 'NONE', ( #2410 ), #9627, .F. ) ;
#16355=CARTESIAN_POINT ( 'NONE',  ( -14.24283201953359956, -44.30969209386396557, -150.0552959529999839 ) ) ;
#16356=LINE ( 'NONE', #16466, #14831 ) ;
#16358=ADVANCED_FACE ( 'NONE', ( #13684 ), #1085, .T. ) ;
#16359=CARTESIAN_POINT ( 'NONE',  ( 14.71940181155087579, 39.42378041200768735, -150.0552959530000123 ) ) ;
#16360=CARTESIAN_POINT ( 'NONE',  ( 19.34345092960000301, -49.66753540199999151, -149.5552959529999839 ) ) ;
#16361=CARTESIAN_POINT ( 'NONE',  ( 1.133692148550000001, 50.50000000000000000, -137.0552959530000123 ) ) ;
#16364=ORIENTED_EDGE ( 'NONE', *, *, #22038, .F. ) ;
#16376=CARTESIAN_POINT ( 'NONE',  ( -5.985376956606384802, 25.11919234682651236, -150.0552959530000123 ) ) ;
#16380=CARTESIAN_POINT ( 'NONE',  ( -32.50000000000000000, 51.00000000000000000, -149.5552959529999839 ) ) ;
#16381=ORIENTED_EDGE ( 'NONE', *, *, #13015, .F. ) ;
#16388=CARTESIAN_POINT ( 'NONE',  ( -31.75000000000000000, 1.000000000000000000, -151.0552959529999839 ) ) ;
#16390=CARTESIAN_POINT ( 'NONE',  ( 5.148789539621256850, -48.22641955295573268, -150.0552959529999839 ) ) ;
#16391=CIRCLE ( 'NONE', #8759, 0.4999999999999987788 ) ;
#16392=LINE ( 'NONE', #103, #21527 ) ;
#16401=ORIENTED_EDGE ( 'NONE', *, *, #14618, .T. ) ;
#16416=LINE ( 'NONE', #20337, #1794 ) ;
#16420=VERTEX_POINT ( 'NONE', #10218 ) ;
#16427=DIRECTION ( 'NONE',  ( 1.000000000000000000, 0.000000000000000000, 0.000000000000000000 ) ) ;
#16432=LINE ( 'NONE', #10573, #1971 ) ;
#16437=B_SPLINE_CURVE_WITH_KNOTS ( 'NONE', 3,
 ( #22320, #4116, #2351, #5666, #13043, #9111, #16728, #5555, #20542, #6014, #319, #14949, #204, #16390, #22209, #12801, #7343, #2230 ),
 .UNSPECIFIED., .F., .F.,
 ( 4, 2, 2, 2, 2, 2, 2, 2, 4 ),
 ( 0.000000000000000000, 0.1250000000000000000, 0.2500000000000000000, 0.3750000000000000000, 0.5000000000000000000, 0.6250000000000000000, 0.7500000000000000000, 0.8750000000000000000, 1.000000000000000000 ),
 .UNSPECIFIED. ) ;
#16442=ORIENTED_EDGE ( 'NONE', *, *, #354, .F. ) ;
#16443=AXIS2_PLACEMENT_3D ( 'NONE', #22683, #13636, #4364 ) ;
#16448=EDGE_LOOP ( 'NONE', ( #14147, #5856, #23459, #18398 ) ) ;
#16455=CARTESIAN_POINT ( 'NONE',  ( 6.500000000000000000, 20.50000000000000000, -151.0552959529999839 ) ) ;
#16459=LINE ( 'NONE', #3848, #19926 ) ;
#16464=CARTESIAN_POINT ( 'NONE',  ( -25.86630785139999844, -51.00000000000000000, -136.0552959530000123 ) ) ;
#16466=CARTESIAN_POINT ( 'NONE',  ( 31.64594224149999846, -40.56768785850000825, -150.0552959529999839 ) ) ;
#16467=DIRECTION ( 'NONE',  ( 0.000000000000000000, 2.256988247090000272E-12, 1.000000000000000000 ) ) ;
#16469=DIRECTION ( 'NONE',  ( 0.000000000000000000, 0.000000000000000000, 1.000000000000000000 ) ) ;
#16476=ORIENTED_EDGE ( 'NONE', *, *, #18049, .F. ) ;
#16480=ORIENTED_EDGE ( 'NONE', *, *, #18197, .T. ) ;
#16493=ORIENTED_EDGE ( 'NONE', *, *, #6385, .F. ) ;
#16494=EDGE_CURVE ( 'NONE', #4645, #22981, #5578, .T. ) ;
#16495=DIRECTION ( 'NONE',  ( -0.7633862853691524286, 0.6459422414661293299, 0.000000000000000000 ) ) ;
#16501=VECTOR ( 'NONE', #15163, 1000.000000000000000 ) ;
#16505=VERTEX_POINT ( 'NONE', #16299 ) ;
#16510=ADVANCED_FACE ( 'NONE', ( #9254 ), #14737, .F. ) ;
#16512=CARTESIAN_POINT ( 'NONE',  ( 31.00000000000000000, 39.80430157320000006, -149.5552959529999839 ) ) ;
#16517=B_SPLINE_CURVE_WITH_KNOTS ( 'NONE', 3,
 ( #8204, #5005, #15472, #3110, #22731, #2990, #6430, #10226, #20963, #4654, #22862, #11895, #6549, #13816, #4768, #17497, #1219, #15714 ),
 .UNSPECIFIED., .F., .F.,
 ( 4, 2, 2, 2, 2, 2, 2, 2, 4 ),
 ( 0.000000000000000000, 0.1250000000000000000, 0.2500000000000000000, 0.3750000000000000000, 0.5000000000000000000, 0.6250000000000000000, 0.7500000000000000000, 0.8750000000000000000, 1.000000000000000000 ),
 .UNSPECIFIED. ) ;
#16532=FACE_OUTER_BOUND ( 'NONE', #7379, .T. ) ;
#16533=FACE_BOUND ( 'NONE', #15519, .T. ) ;
#16539=LINE ( 'NONE', #22020, #4579 ) ;
#16540=CARTESIAN_POINT ( 'NONE',  ( 32.50000000000000000, -40.03620104880000241, -149.5552959529999839 ) ) ;
#16542=CARTESIAN_POINT ( 'NONE',  ( -32.00000000000000000, 19.50000000000000000, -149.5552959529999839 ) ) ;
#16551=LINE ( 'NONE', #18350, #23424 ) ;
#16553=DIRECTION ( 'NONE',  ( 0.000000000000000000, 0.000000000000000000, -1.000000000000000000 ) ) ;
#16567=LINE ( 'NONE', #278, #17474 ) ;
#16568=VECTOR ( 'NONE', #7258, 1000.000000000000000 ) ;
#16573=CARTESIAN_POINT ( 'NONE',  ( 31.96891336220000213, 40.94938100119999547, -149.5552959529999839 ) ) ;
#16578=DIRECTION ( 'NONE',  ( 0.7633862853691524286, -0.6459422414661292189, 2.187574565940437122E-17 ) ) ;
#16583=EDGE_LOOP ( 'NONE', ( #5997, #15377, #20204, #23037 ) ) ;
#16587=ORIENTED_EDGE ( 'NONE', *, *, #19673, .T. ) ;
#16589=LINE ( 'NONE', #18384, #22096 ) ;
#16591=EDGE_LOOP ( 'NONE', ( #17501, #9718, #8457, #17592 ) ) ;
#16603=DIRECTION ( 'NONE',  ( 0.000000000000000000, 0.000000000000000000, -1.000000000000000000 ) ) ;
#16605=DIRECTION ( 'NONE',  ( 0.000000000000000000, 1.000000000000000000, 0.000000000000000000 ) ) ;
#16608=AXIS2_PLACEMENT_3D ( 'NONE', #9392, #11296, #20141 ) ;
#16613=VECTOR ( 'NONE', #16469, 1000.000000000000000 ) ;
#16614=ORIENTED_EDGE ( 'NONE', *, *, #7640, .T. ) ;
#16615=CARTESIAN_POINT ( 'NONE',  ( -18.00000000000000000, -43.00000000000000000, -150.0552959529999839 ) ) ;
#16621=CARTESIAN_POINT ( 'NONE',  ( 13.61765588494693802, 22.91567315752959644, -150.0552959529999555 ) ) ;
#16628=B_SPLINE_CURVE_WITH_KNOTS ( 'NONE', 3,
 ( #16615, #14955, #18761, #212, #4015, #14844, #450, #2119, #566, #9693, #2472, #22103, #11243, #15069, #9341, #16968, #6022, #22330 ),
 .UNSPECIFIED., .F., .F.,
 ( 4, 2, 2, 2, 2, 2, 2, 2, 4 ),
 ( 0.000000000000000000, 0.1250000000000002776, 0.2500000000000005551, 0.3750000000000008327, 0.5000000000000011102, 0.6250000000000007772, 0.7500000000000005551, 0.8750000000000002220, 1.000000000000000000 ),
 .UNSPECIFIED. ) ;
#16638=ORIENTED_EDGE ( 'NONE', *, *, #16058, .T. ) ;
#16640=LINE ( 'NONE', #7937, #9328 ) ;
#16643=CARTESIAN_POINT ( 'NONE',  ( 6.750000000000000000, -47.00000000000000000, -151.0552959529999839 ) ) ;
#16645=DIRECTION ( 'NONE',  ( 0.000000000000000000, 0.000000000000000000, -1.000000000000000000 ) ) ;
#16649=VECTOR ( 'NONE', #18222, 1000.000000000000000 ) ;
#16651=FACE_OUTER_BOUND ( 'NONE', #19505, .T. ) ;
#16655=FACE_OUTER_BOUND ( 'NONE', #1536, .T. ) ;
#16656=LINE ( 'NONE', #16892, #15182 ) ;
#16659=DIRECTION ( 'NONE',  ( -2.257252162960000001E-12, 0.000000000000000000, -1.000000000000000000 ) ) ;
#16660=ADVANCED_FACE ( 'NONE', ( #12066 ), #6600, .F. ) ;
#16663=ORIENTED_EDGE ( 'NONE', *, *, #14639, .F. ) ;
#16664=DIRECTION ( 'NONE',  ( -2.257144641399999941E-12, 0.000000000000000000, -1.000000000000000000 ) ) ;
#16667=CIRCLE ( 'NONE', #5658, 2.999999999999999112 ) ;
#16670=ORIENTED_EDGE ( 'NONE', *, *, #6442, .F. ) ;
#16674=DIRECTION ( 'NONE',  ( 0.000000000000000000, -1.000000000000000000, 0.000000000000000000 ) ) ;
#16675=CARTESIAN_POINT ( 'NONE',  ( 6.500000000000000000, 20.50000000000000000, -150.0552959529999839 ) ) ;
#16676=VECTOR ( 'NONE', #14884, 1000.000000000000000 ) ;
#16689=DIRECTION ( 'NONE',  ( 1.000000000000000000, 0.000000000000000000, 0.000000000000000000 ) ) ;
#16692=PLANE ( 'NONE',  #13624 ) ;
#16696=CARTESIAN_POINT ( 'NONE',  ( 15.10234832539273420, 33.50000000000000000, -150.0552959530000123 ) ) ;
#16697=DIRECTION ( 'NONE',  ( -1.000000000000000000, 0.000000000000000000, 2.257144641399999941E-12 ) ) ;
#16708=VERTEX_POINT ( 'NONE', #1627 ) ;
#16714=LINE ( 'NONE', #427, #15589 ) ;
#16724=CARTESIAN_POINT ( 'NONE',  ( -31.50000000000000000, -50.00000000000000000, -143.3052959529999839 ) ) ;
#16728=CARTESIAN_POINT ( 'NONE',  ( 7.759759976955875160, -48.74600213680044192, -150.0552959529999839 ) ) ;
#16740=ORIENTED_EDGE ( 'NONE', *, *, #8375, .F. ) ;
#16742=CARTESIAN_POINT ( 'NONE',  ( -4.500000000000000000, 34.00000000000000000, -151.0552959529999839 ) ) ;
#16748=CARTESIAN_POINT ( 'NONE',  ( -1.500000000000000000, 44.50000000000000000, -150.0552959529999839 ) ) ;
#16749=ADVANCED_FACE ( 'NONE', ( #22918 ), #8498, .F. ) ;
#16750=DIRECTION ( 'NONE',  ( 0.000000000000000000, 0.000000000000000000, 1.000000000000000000 ) ) ;
#16752=VECTOR ( 'NONE', #1357, 1000.000000000000000 ) ;
#16753=ORIENTED_EDGE ( 'NONE', *, *, #22750, .T. ) ;
#16754=VECTOR ( 'NONE', #12031, 1000.000000000000000 ) ;
#16758=CARTESIAN_POINT ( 'NONE',  ( 20.50000000000000000, 25.50000000000000000, -151.0552959529999839 ) ) ;
#16763=CARTESIAN_POINT ( 'NONE',  ( -31.75000000000000000, -36.00000000000000000, -151.0552959529999839 ) ) ;
#16771=DIRECTION ( 'NONE',  ( 0.000000000000000000, 2.256988247090000272E-12, 1.000000000000000000 ) ) ;
#16774=LINE ( 'NONE', #16542, #9173 ) ;
#16775=VECTOR ( 'NONE', #20718, 1000.000000000000000 ) ;
#16778=VECTOR ( 'NONE', #22869, 1000.000000000000000 ) ;
#16787=EDGE_CURVE ( 'NONE', #3797, #9003, #15878, .T. ) ;
#16788=LINE ( 'NONE', #502, #2857 ) ;
#16797=EDGE_CURVE ( 'NONE', #6475, #20332, #8962, .T. ) ;
#16801=LINE ( 'NONE', #7743, #15529 ) ;
#16805=CARTESIAN_POINT ( 'NONE',  ( -29.18315392600000280, -51.50000000000000000, -136.0552959530000123 ) ) ;
#16806=ORIENTED_EDGE ( 'NONE', *, *, #3389, .F. ) ;
#16808=LINE ( 'NONE', #7637, #18348 ) ;
#16810=ORIENTED_EDGE ( 'NONE', *, *, #11423, .T. ) ;
#16817=ADVANCED_FACE ( 'NONE', ( #12893 ), #20174, .F. ) ;
#16820=CARTESIAN_POINT ( 'NONE',  ( 12.57650987475213533, 37.28094649259004711, -150.0552959529999839 ) ) ;
#16828=AXIS2_PLACEMENT_3D ( 'NONE', #19651, #3232, #4900 ) ;
#16830=VERTEX_POINT ( 'NONE', #10861 ) ;
#16832=EDGE_LOOP ( 'NONE', ( #4209, #18332, #3619, #5535 ) ) ;
#16833=CARTESIAN_POINT ( 'NONE',  ( -18.00000000000000000, -43.00000000000000000, -145.5552959529999839 ) ) ;
#16835=DIRECTION ( 'NONE',  ( 0.000000000000000000, -1.000000000000000000, 0.000000000000000000 ) ) ;
#16839=ORIENTED_EDGE ( 'NONE', *, *, #22546, .T. ) ;
#16851=VERTEX_POINT ( 'NONE', #16361 ) ;
#16857=ORIENTED_EDGE ( 'NONE', *, *, #9632, .T. ) ;
#16861=CARTESIAN_POINT ( 'NONE',  ( 9.824773488038593072, 27.24096059670178249, -150.0552959529999555 ) ) ;
#16862=CARTESIAN_POINT ( 'NONE',  ( 25.31684607480000082, -45.26810052389999584, -136.0552959530000123 ) ) ;
#16869=FACE_OUTER_BOUND ( 'NONE', #23294, .T. ) ;
#16877=VERTEX_POINT ( 'NONE', #9197 ) ;
#16883=VERTEX_POINT ( 'NONE', #11209 ) ;
#16884=CARTESIAN_POINT ( 'NONE',  ( -5.449075813550353864, 45.02080533206300572, -150.0552959530000123 ) ) ;
#16888=CYLINDRICAL_SURFACE ( 'NONE', #8379, 1.499999999999999556 ) ;
#16889=VERTEX_POINT ( 'NONE', #14683 ) ;
#16892=CARTESIAN_POINT ( 'NONE',  ( 32.00000000000000000, 40.03620104880000241, -150.0552959529999839 ) ) ;
#16894=LINE ( 'NONE', #6763, #18580 ) ;
#16902=DIRECTION ( 'NONE',  ( 1.000000000000000000, 0.000000000000000000, -2.257453483404482811E-12 ) ) ;
#16907=CARTESIAN_POINT ( 'NONE',  ( -15.39061678755858864, -41.53835085783378389, -150.0552959529999839 ) ) ;
#16910=EDGE_CURVE ( 'NONE', #12787, #7959, #15401, .T. ) ;
#16925=EDGE_CURVE ( 'NONE', #15915, #18797, #17047, .T. ) ;
#16926=VECTOR ( 'NONE', #2691, 1000.000000000000000 ) ;
#16933=CARTESIAN_POINT ( 'NONE',  ( -32.50000000000000000, 1.000000000000000000, -143.3052959529999839 ) ) ;
#16938=B_SPLINE_CURVE_WITH_KNOTS ( 'NONE', 3,
 ( #13830, #10242, #22745, #5128, #19653, #17278, #21212, #6447, #4901, #13706, #10119, #15614, #21093, #17512, #1235, #8460, #21920, #20250 ),
 .UNSPECIFIED., .F., .F.,
 ( 4, 2, 2, 2, 2, 2, 2, 2, 4 ),
 ( 0.000000000000000000, 0.1250000000000000000, 0.2500000000000000000, 0.3750000000000000000, 0.5000000000000000000, 0.6250000000000000000, 0.7500000000000000000, 0.8750000000000000000, 1.000000000000000000 ),
 .UNSPECIFIED. ) ;
#16946=EDGE_LOOP ( 'NONE', ( #15187, #5095 ) ) ;
#16950=ORIENTED_EDGE ( 'NONE', *, *, #9133, .T. ) ;
#16960=DIRECTION ( 'NONE',  ( 1.000000000000000000, 0.000000000000000000, 0.000000000000000000 ) ) ;
#16968=CARTESIAN_POINT ( 'NONE',  ( -12.07808196999504879, -43.78524365307782062, -150.0552959529999555 ) ) ;
#16969=ORIENTED_EDGE ( 'NONE', *, *, #14309, .F. ) ;
#16975=CARTESIAN_POINT ( 'NONE',  ( 4.500000000000000000, -3.500000000000000000, -145.5552959529999839 ) ) ;
#16980=DIRECTION ( 'NONE',  ( 0.000000000000000000, 0.000000000000000000, 1.000000000000000000 ) ) ;
#16989=ORIENTED_EDGE ( 'NONE', *, *, #22924, .T. ) ;
#16996=CARTESIAN_POINT ( 'NONE',  ( -3.500000000000000000, 46.50000000000000000, -150.0552959529999839 ) ) ;
#17000=CARTESIAN_POINT ( 'NONE',  ( -15.00000000000000000, -43.00000000000000000, -145.5552959529999839 ) ) ;
#17001=EDGE_CURVE ( 'NONE', #16420, #22568, #15504, .T. ) ;
#17012=ORIENTED_EDGE ( 'NONE', *, *, #3400, .T. ) ;
#17013=CARTESIAN_POINT ( 'NONE',  ( 3.714756346922155839, -0.5780819699950539015, -150.0552959529999839 ) ) ;
#17015=CYLINDRICAL_SURFACE ( 'NONE', #9766, 1.500000000000001332 ) ;
#17017=ORIENTED_EDGE ( 'NONE', *, *, #4547, .T. ) ;
#17029=CYLINDRICAL_SURFACE ( 'NONE', #20223, 2.999999999999999112 ) ;
#17038=AXIS2_PLACEMENT_3D ( 'NONE', #14637, #3335, #16427 ) ;
#17044=VECTOR ( 'NONE', #18190, 1000.000000000000227 ) ;
#17047=LINE ( 'NONE', #15151, #5136 ) ;
#17053=VECTOR ( 'NONE', #20906, 1000.000000000000000 ) ;
#17060=ORIENTED_EDGE ( 'NONE', *, *, #3419, .F. ) ;
#17061=VECTOR ( 'NONE', #19716, 1000.000000000000000 ) ;
#17064=ORIENTED_EDGE ( 'NONE', *, *, #15610, .F. ) ;
#17071=AXIS2_PLACEMENT_3D ( 'NONE', #12861, #18352, #16553 ) ;
#17075=ADVANCED_FACE ( 'NONE', ( #17290 ), #1002, .F. ) ;
#17077=VECTOR ( 'NONE', #1318, 1000.000000000000000 ) ;
#17079=CARTESIAN_POINT ( 'NONE',  ( -15.50000000000000000, 21.50000000000000000, -150.5552959529999839 ) ) ;
#17084=DIRECTION ( 'NONE',  ( 0.000000000000000000, 0.000000000000000000, 1.000000000000000000 ) ) ;
#17087=EDGE_CURVE ( 'NONE', #19419, #17813, #18258, .T. ) ;
#17088=ORIENTED_EDGE ( 'NONE', *, *, #4815, .F. ) ;
#17092=LINE ( 'NONE', #809, #8708 ) ;
#17103=DIRECTION ( 'NONE',  ( 1.000000000000000000, 0.000000000000000000, 0.000000000000000000 ) ) ;
#17106=EDGE_CURVE ( 'NONE', #17493, #4135, #21224, .T. ) ;
#17108=PLANE ( 'NONE',  #4848 ) ;
#17133=VECTOR ( 'NONE', #9648, 1000.000000000000000 ) ;
#17139=FACE_OUTER_BOUND ( 'NONE', #521, .T. ) ;
#17143=CARTESIAN_POINT ( 'NONE',  ( -7.500000000000000000, 25.50000000000000000, -150.5552959529999839 ) ) ;
#17148=VECTOR ( 'NONE', #17735, 1000.000000000000000 ) ;
#17153=LINE ( 'NONE', #11659, #1699 ) ;
#17167=EDGE_CURVE ( 'NONE', #5668, #15811, #21345, .T. ) ;
#17169=CARTESIAN_POINT ( 'NONE',  ( 1.544882029667944634, 14.84887268567880270, -150.0552959529999839 ) ) ;
#17174=CARTESIAN_POINT ( 'NONE',  ( 8.976561295253542738, -38.03342539458719074, -150.0552959529999555 ) ) ;
#17180=VECTOR ( 'NONE', #1229, 1000.000000000000000 ) ;
#17181=CARTESIAN_POINT ( 'NONE',  ( 18.95053822279999878, 50.00000000000000000, -150.0552959529999839 ) ) ;
#17182=CIRCLE ( 'NONE', #9945, 0.5000000000000009992 ) ;
#17185=DIRECTION ( 'NONE',  ( 1.000000000000000000, 0.000000000000000000, 0.000000000000000000 ) ) ;
#17187=ORIENTED_EDGE ( 'NONE', *, *, #4894, .T. ) ;
#17188=FACE_OUTER_BOUND ( 'NONE', #15443, .T. ) ;
#17193=CARTESIAN_POINT ( 'NONE',  ( 3.000000000000000000, -3.500000000000000000, -150.0552959529999839 ) ) ;
#17198=ORIENTED_EDGE ( 'NONE', *, *, #20568, .T. ) ;
#17201=CARTESIAN_POINT ( 'NONE',  ( -13.86630785140000022, 50.99999999970000175, -136.0552959530000123 ) ) ;
#17203=ORIENTED_EDGE ( 'NONE', *, *, #17167, .T. ) ;
#17221=DIRECTION ( 'NONE',  ( 0.000000000000000000, 0.000000000000000000, 1.000000000000000000 ) ) ;
#17229=CARTESIAN_POINT ( 'NONE',  ( 20.50000000000000355, -20.89269908169873347, -150.0552959530000123 ) ) ;
#17234=EDGE_CURVE ( 'NONE', #3138, #21821, #9521, .T. ) ;
#17236=ORIENTED_EDGE ( 'NONE', *, *, #22546, .F. ) ;
#17239=B_SPLINE_CURVE_WITH_KNOTS ( 'NONE', 3,
 ( #14925, #22182, #5868, #13126, #18608, #10263, #13842, #15630, #4563, #1128, #6578, #22895, #8358, #3026, #2901, #13365, #11803, #13723, #17291, #9773, #6342, #1003, #15742, #21109, #19080, #15506, #17530, #4330, #2670, #10132, #4799, #12043, #17174, #13596 ),
 .UNSPECIFIED., .F., .F.,
 ( 4, 2, 2, 2, 2, 2, 2, 2, 2, 2, 2, 2, 2, 2, 2, 2, 4 ),
 ( 0.000000000000000000, 0.06250000000000004163, 0.1250000000000000833, 0.1875000000000001943, 0.2500000000000002776, 0.3125000000000003331, 0.3750000000000003886, 0.4375000000000003886, 0.5000000000000004441, 0.5625000000000004441, 0.6250000000000004441, 0.6875000000000003331, 0.7500000000000002220, 0.8125000000000002220, 0.8750000000000001110, 0.9375000000000001110, 1.000000000000000000 ),
 .UNSPECIFIED. ) ;
#17249=ADVANCED_FACE ( 'NONE', ( #7851 ), #6200, .T. ) ;
#17251=ORIENTED_EDGE ( 'NONE', *, *, #11999, .F. ) ;
#17268=DIRECTION ( 'NONE',  ( 1.000000000000000000, 0.000000000000000000, 0.000000000000000000 ) ) ;
#17271=CARTESIAN_POINT ( 'NONE',  ( 20.50000000000000000, -20.50000000000000000, -143.5552959529999839 ) ) ;
#17277=EDGE_CURVE ( 'NONE', #13352, #18640, #20715, .T. ) ;
#17278=CARTESIAN_POINT ( 'NONE',  ( 5.419886383052536338, -2.299140194000087511, -150.0552959529999839 ) ) ;
#17279=ORIENTED_EDGE ( 'NONE', *, *, #10028, .T. ) ;
#17281=DIRECTION ( 'NONE',  ( -1.000000000000000000, 0.000000000000000000, -2.245315044999999693E-12 ) ) ;
#17283=ORIENTED_EDGE ( 'NONE', *, *, #21016, .F. ) ;
#17290=FACE_OUTER_BOUND ( 'NONE', #11785, .T. ) ;
#17291=CARTESIAN_POINT ( 'NONE',  ( 7.351088731964408041, -33.04529868153298366, -150.0552959529999839 ) ) ;
#17293=SURFACE_SIDE_STYLE ('',( #4802 ) ) ;
#17302=AXIS2_PLACEMENT_3D ( 'NONE', #20607, #4530, #2300 ) ;
#17307=CARTESIAN_POINT ( 'NONE',  ( -16.50000000000000000, -43.19873783136716128, -150.0552959530000123 ) ) ;
#17313=VECTOR ( 'NONE', #19958, 1000.000000000000000 ) ;
#17314=CARTESIAN_POINT ( 'NONE',  ( -15.00000000000000000, -43.00000000000000000, -140.0552959529999839 ) ) ;
#17318=ORIENTED_EDGE ( 'NONE', *, *, #8060, .F. ) ;
#17320=ORIENTED_EDGE ( 'NONE', *, *, #8041, .T. ) ;
#17321=LINE ( 'NONE', #6258, #10631 ) ;
#17324=ADVANCED_FACE ( 'NONE', ( #4065 ), #22268, .F. ) ;
#17331=ORIENTED_EDGE ( 'NONE', *, *, #5639, .T. ) ;
#17338=ORIENTED_EDGE ( 'NONE', *, *, #11917, .F. ) ;
#17341=ORIENTED_EDGE ( 'NONE', *, *, #16238, .T. ) ;
#17347=CARTESIAN_POINT ( 'NONE',  ( 21.98914305888730780, -23.12135916506278122, -150.0552959529999839 ) ) ;
#17355=DIRECTION ( 'NONE',  ( -0.6459422414661291079, -0.7633862853691523176, -2.245315045000450442E-12 ) ) ;
#17360=ORIENTED_EDGE ( 'NONE', *, *, #20164, .F. ) ;
#17367=ORIENTED_EDGE ( 'NONE', *, *, #7602, .T. ) ;
#17373=LINE ( 'NONE', #861, #20062 ) ;
#17374=CARTESIAN_POINT ( 'NONE',  ( -32.50000000000000000, 19.50000000000000000, -149.5552959529999839 ) ) ;
#17375=EDGE_CURVE ( 'NONE', #10456, #12686, #4652, .T. ) ;
#17377=CARTESIAN_POINT ( 'NONE',  ( -15.19857565926003673, -41.49993277010363357, -150.0552959530000123 ) ) ;
#17379=LINE ( 'NONE', #22980, #13229 ) ;
#17380=EDGE_CURVE ( 'NONE', #4360, #6192, #3108, .T. ) ;
#17388=DIRECTION ( 'NONE',  ( 3.494344380199214996E-12, 0.000000000000000000, -1.000000000000000000 ) ) ;
#17389=DIRECTION ( 'NONE',  ( 0.000000000000000000, 0.000000000000000000, 1.000000000000000000 ) ) ;
#17398=ORIENTED_EDGE ( 'NONE', *, *, #5328, .T. ) ;
#17402=FACE_OUTER_BOUND ( 'NONE', #11327, .T. ) ;
#17406=ADVANCED_FACE ( 'NONE', ( #13924 ), #1328, .F. ) ;
#17412=ORIENTED_EDGE ( 'NONE', *, *, #668, .T. ) ;
#17421=CARTESIAN_POINT ( 'NONE',  ( -31.50000000000000000, -36.00000000000000000, -149.5552959529999839 ) ) ;
#17425=DIRECTION ( 'NONE',  ( 0.000000000000000000, 0.000000000000000000, 1.000000000000000000 ) ) ;
#17427=CARTESIAN_POINT ( 'NONE',  ( 5.809451030008016659, -4.257397883940200245, -150.0552959529999839 ) ) ;
#17430=EDGE_CURVE ( 'NONE', #23438, #328, #1745, .T. ) ;
#17443=ORIENTED_EDGE ( 'NONE', *, *, #19207, .F. ) ;
#17444=PLANE ( 'NONE',  #2293 ) ;
#17445=CARTESIAN_POINT ( 'NONE',  ( 32.50000000000000000, 40.03620104890000420, -136.0552959530000123 ) ) ;
#17447=CARTESIAN_POINT ( 'NONE',  ( 32.50000000000000000, 39.80430157320000006, -149.8052959529999839 ) ) ;
#17456=CARTESIAN_POINT ( 'NONE',  ( -32.00000000000000000, -36.00000000000000000, -149.5552959529999839 ) ) ;
#17457=ORIENTED_EDGE ( 'NONE', *, *, #3451, .F. ) ;
#17459=DIRECTION ( 'NONE',  ( 0.6459422414661299960, -0.7633862853691516515, 0.000000000000000000 ) ) ;
#17462=CARTESIAN_POINT ( 'NONE',  ( 1.133692148550000001, 51.50000000000000000, -137.0552959530000123 ) ) ;
#17464=LINE ( 'NONE', #15562, #8180 ) ;
#17474=VECTOR ( 'NONE', #7519, 1000.000000000000000 ) ;
#17478=CARTESIAN_POINT ( 'NONE',  ( -3.500000000000000000, 44.50000000000000000, -150.0552959529999839 ) ) ;
#17492=LINE ( 'NONE', #10221, #15569 ) ;
#17493=VERTEX_POINT ( 'NONE', #17374 ) ;
#17496=DIRECTION ( 'NONE',  ( 0.000000000000000000, 1.000000000000000000, 0.000000000000000000 ) ) ;
#17497=CARTESIAN_POINT ( 'NONE',  ( 20.57808196999505412, -19.71475634692216872, -150.0552959530000123 ) ) ;
#17499=CARTESIAN_POINT ( 'NONE',  ( 31.50000000000000000, -39.80430157320000006, -149.5552959529999839 ) ) ;
#17501=ORIENTED_EDGE ( 'NONE', *, *, #20730, .F. ) ;
#17507=CARTESIAN_POINT ( 'NONE',  ( -7.500000000000000000, 19.50000000000000000, -150.5552959529999839 ) ) ;
#17512=CARTESIAN_POINT ( 'NONE',  ( 3.299140194000170556, -2.580113616947039556, -150.0552959529999839 ) ) ;
#17518=EDGE_LOOP ( 'NONE', ( #595, #11463, #11892, #16169 ) ) ;
#17525=ORIENTED_EDGE ( 'NONE', *, *, #11559, .F. ) ;
#17527=AXIS2_PLACEMENT_3D ( 'NONE', #5664, #20199, #18053 ) ;
#17530=CARTESIAN_POINT ( 'NONE',  ( 9.724682038177496324, -35.50721777958683134, -150.0552959529999839 ) ) ;
#17532=ORIENTED_EDGE ( 'NONE', *, *, #22410, .F. ) ;
#17533=FILL_AREA_STYLE_COLOUR ( '', #15999 ) ;
#17540=EDGE_CURVE ( 'NONE', #8058, #213, #6678, .T. ) ;
#17541=ORIENTED_EDGE ( 'NONE', *, *, #15210, .F. ) ;
#17542=FACE_OUTER_BOUND ( 'NONE', #23299, .T. ) ;
#17548=CYLINDRICAL_SURFACE ( 'NONE', #1564, 1.500000000000001332 ) ;
#17552=CARTESIAN_POINT ( 'NONE',  ( -16.30969209386606167, -43.75716798044907563, -150.0552959530000123 ) ) ;
#17557=CARTESIAN_POINT ( 'NONE',  ( 4.301424340775872324, -4.999932770097081480, -150.0552959529999555 ) ) ;
#17560=B_SPLINE_CURVE_WITH_KNOTS ( 'NONE', 3,
 ( #14212, #21718, #8839, #10739, #58, #1731, #12653, #19682, #7066, #3380, #21243, #12182, #17900, #3158, #21596, #1621, #3506, #5280 ),
 .UNSPECIFIED., .F., .F.,
 ( 4, 2, 2, 2, 2, 2, 2, 2, 4 ),
 ( 0.000000000000000000, 0.1250000000000000000, 0.2500000000000000000, 0.3750000000000000000, 0.5000000000000000000, 0.6250000000000000000, 0.7500000000000000000, 0.8750000000000000000, 1.000000000000000000 ),
 .UNSPECIFIED. ) ;
#17561=EDGE_LOOP ( 'NONE', ( #19340, #11286, #14468, #19820 ) ) ;
#17564=VECTOR ( 'NONE', #13484, 1000.000000000000000 ) ;
#17567=EDGE_LOOP ( 'NONE', ( #9726, #505, #17457, #18010 ) ) ;
#17570=CARTESIAN_POINT ( 'NONE',  ( 1.133692148550000001, -50.50000000000000000, -137.0552959530000123 ) ) ;
#17572=ORIENTED_EDGE ( 'NONE', *, *, #10028, .F. ) ;
#17574=LINE ( 'NONE', #2817, #7949 ) ;
#17584=AXIS2_PLACEMENT_3D ( 'NONE', #5098, #10550, #17832 ) ;
#17589=ORIENTED_EDGE ( 'NONE', *, *, #21042, .F. ) ;
#17591=CARTESIAN_POINT ( 'NONE',  ( 18.95053822279999878, 50.00000000000000000, -150.0552959529999839 ) ) ;
#17592=ORIENTED_EDGE ( 'NONE', *, *, #15465, .F. ) ;
#17607=ADVANCED_FACE ( 'NONE', ( #16532 ), #16304, .F. ) ;
#17610=EDGE_CURVE ( 'NONE', #9607, #5909, #16185, .T. ) ;
#17615=DIRECTION ( 'NONE',  ( -0.6459422414661291079, 0.7633862853691523176, -2.245315045000450442E-12 ) ) ;
#17621=CARTESIAN_POINT ( 'NONE',  ( -6.024730888589999722, -50.00000000000000000, -151.0552959529999839 ) ) ;
#17622=CARTESIAN_POINT ( 'NONE',  ( 31.32297112069999656, -40.18599471579999971, -143.0552959529999839 ) ) ;
#17626=DIRECTION ( 'NONE',  ( 1.000000000000000000, 0.000000000000000000, 0.000000000000000000 ) ) ;
#17629=DIRECTION ( 'NONE',  ( 0.000000000000000000, -1.000000000000000000, 2.257144641399999941E-12 ) ) ;
#17631=ADVANCED_FACE ( 'NONE', ( #8905 ), #21791, .F. ) ;
#17637=DIRECTION ( 'NONE',  ( 1.000000000000000000, 0.000000000000000000, 0.000000000000000000 ) ) ;
#17638=ORIENTED_EDGE ( 'NONE', *, *, #11081, .F. ) ;
#17640=CARTESIAN_POINT ( 'NONE',  ( 6.500000000000000000, 20.50000000000000000, -150.0552959529999839 ) ) ;
#17646=CARTESIAN_POINT ( 'NONE',  ( 2.742437130618089913, 27.00952979664189968, -150.0552959529999839 ) ) ;
#17650=ORIENTED_EDGE ( 'NONE', *, *, #15058, .T. ) ;
#17652=EDGE_CURVE ( 'NONE', #2146, #5378, #14525, .T. ) ;
#17655=CARTESIAN_POINT ( 'NONE',  ( 25.00000000000000000, -20.50000000000000000, -137.0552959530000123 ) ) ;
#17658=CARTESIAN_POINT ( 'NONE',  ( -32.50000000000000000, 51.50000000000000000, -151.0552959529999839 ) ) ;
#17661=ORIENTED_EDGE ( 'NONE', *, *, #1313, .F. ) ;
#17664=DIRECTION ( 'NONE',  ( 1.000000000000000000, 0.000000000000000000, 0.000000000000000000 ) ) ;
#17675=EDGE_CURVE ( 'NONE', #10143, #384, #12605, .T. ) ;
#17679=DIRECTION ( 'NONE',  ( 0.000000000000000000, 0.000000000000000000, 1.000000000000000000 ) ) ;
#17680=ORIENTED_EDGE ( 'NONE', *, *, #18855, .T. ) ;
#17681=EDGE_CURVE ( 'NONE', #1386, #4332, #16640, .T. ) ;
#17693=FACE_OUTER_BOUND ( 'NONE', #211, .T. ) ;
#17717=CARTESIAN_POINT ( 'NONE',  ( 23.00000000000000000, 25.50000000000000000, -150.0552959529999839 ) ) ;
#17719=VERTEX_POINT ( 'NONE', #20573 ) ;
#17722=DIRECTION ( 'NONE',  ( 0.000000000000000000, 1.000000000000000000, 0.000000000000000000 ) ) ;
#17727=ORIENTED_EDGE ( 'NONE', *, *, #2459, .F. ) ;
#17728=DIRECTION ( 'NONE',  ( -0.7633862853691524286, 0.6459422414661292189, 1.776356839390353219E-15 ) ) ;
#17732=EDGE_CURVE ( 'NONE', #17914, #4735, #4151, .T. ) ;
#17735=DIRECTION ( 'NONE',  ( -1.000000000000000000, 0.000000000000000000, 2.245315044999999693E-12 ) ) ;
#17747=DIRECTION ( 'NONE',  ( 0.000000000000000000, -1.000000000000000000, 0.000000000000000000 ) ) ;
#17750=LINE ( 'NONE', #8924, #15924 ) ;
#17754=ORIENTED_EDGE ( 'NONE', *, *, #20170, .F. ) ;
#17757=CARTESIAN_POINT ( 'NONE',  ( 19.00000000000000000, 39.50000000000000000, -150.0552959529999839 ) ) ;
#17758=ADVANCED_FACE ( 'NONE', ( #22128 ), #4273, .F. ) ;
#17761=ADVANCED_FACE ( 'NONE', ( #8054 ), #11504, .T. ) ;
#17767=DIRECTION ( 'NONE',  ( 0.6459422414661291079, -0.7633862853691523176, 2.245315045000450442E-12 ) ) ;
#17768=DIRECTION ( 'NONE',  ( 0.000000000000000000, 1.000000000000000000, 0.000000000000000000 ) ) ;
#17772=ORIENTED_EDGE ( 'NONE', *, *, #19703, .T. ) ;
#17776=LINE ( 'NONE', #11940, #5566 ) ;
#17780=CARTESIAN_POINT ( 'NONE',  ( -19.86630785140000199, -51.50000000000000000, -137.0552959530000123 ) ) ;
#17785=EDGE_LOOP ( 'NONE', ( #8359, #10400, #20322, #16806 ) ) ;
#17790=ORIENTED_EDGE ( 'NONE', *, *, #21919, .F. ) ;
#17796=ORIENTED_EDGE ( 'NONE', *, *, #14309, .T. ) ;
#17802=ORIENTED_EDGE ( 'NONE', *, *, #17675, .F. ) ;
#17803=PLANE ( 'NONE',  #6487 ) ;
#17809=PLANE ( 'NONE',  #16329 ) ;
#17813=VERTEX_POINT ( 'NONE', #18893 ) ;
#17816=VECTOR ( 'NONE', #21300, 1000.000000000000000 ) ;
#17819=ORIENTED_EDGE ( 'NONE', *, *, #15587, .F. ) ;
#17820=DIRECTION ( 'NONE',  ( 0.000000000000000000, 2.257144641399999941E-12, -1.000000000000000000 ) ) ;
#17821=DIRECTION ( 'NONE',  ( 0.000000000000000000, 0.000000000000000000, 1.000000000000000000 ) ) ;
#17823=CARTESIAN_POINT ( 'NONE',  ( 26.50000000000000711, -20.89269908169871570, -150.0552959529999839 ) ) ;
#17826=CARTESIAN_POINT ( 'NONE',  ( -5.101575545681980017, 43.27312978694517653, -150.0552959529999839 ) ) ;
#17832=DIRECTION ( 'NONE',  ( 1.000000000000000000, 0.000000000000000000, 0.000000000000000000 ) ) ;
#17833=EDGE_LOOP ( 'NONE', ( #7429, #3673, #23224, #19379 ) ) ;
#17843=ORIENTED_EDGE ( 'NONE', *, *, #8509, .T. ) ;
#17847=VECTOR ( 'NONE', #23436, 1000.000000000000000 ) ;
#17853=VECTOR ( 'NONE', #1392, 1000.000000000000000 ) ;
#17854=FACE_BOUND ( 'NONE', #13130, .T. ) ;
#17857=VECTOR ( 'NONE', #6832, 1000.000000000000000 ) ;
#17863=DIRECTION ( 'NONE',  ( -1.000000000000000000, 0.000000000000000000, 0.000000000000000000 ) ) ;
#17867=ORIENTED_EDGE ( 'NONE', *, *, #21807, .F. ) ;
#17871=VECTOR ( 'NONE', #8271, 1000.000000000000000 ) ;
#17873=EDGE_CURVE ( 'NONE', #232, #12791, #17464, .T. ) ;
#17875=ADVANCED_FACE ( 'NONE', ( #1411 ), #3191, .T. ) ;
#17876=CARTESIAN_POINT ( 'NONE',  ( 25.00000000000000000, -20.50000000000000000, -135.0552959530000123 ) ) ;
#17877=VERTEX_POINT ( 'NONE', #15688 ) ;
#17880=DIRECTION ( 'NONE',  ( 1.000000000000000000, 0.000000000000000000, 0.000000000000000000 ) ) ;
#17887=ORIENTED_EDGE ( 'NONE', *, *, #22496, .F. ) ;
#17896=CARTESIAN_POINT ( 'NONE',  ( -32.50000000000000000, 21.50000000000000000, -151.0552959529999839 ) ) ;
#17899=ADVANCED_FACE ( 'NONE', ( #19375 ), #6394, .F. ) ;
#17900=CARTESIAN_POINT ( 'NONE',  ( 18.09818317339652083, 24.33939095839998856, -150.0552959529999839 ) ) ;
#17902=VECTOR ( 'NONE', #19946, 1000.000000000000000 ) ;
#17903=EDGE_CURVE ( 'NONE', #7233, #9003, #8167, .T. ) ;
#17912=B_SPLINE_CURVE_WITH_KNOTS ( 'NONE', 1,
 ( #10223, #6659 ),
 .UNSPECIFIED., .F., .F.,
 ( 2, 2 ),
 ( -6.000000000000000000, 6.000000000000000000 ),
 .UNSPECIFIED. ) ;
#17913=CARTESIAN_POINT ( 'NONE',  ( -15.50000000000000000, 47.50000000000000000, -151.0552959529999839 ) ) ;
#17914=VERTEX_POINT ( 'NONE', #17591 ) ;
#17920=VECTOR ( 'NONE', #4656, 1000.000000000000000 ) ;
#17922=VECTOR ( 'NONE', #19055, 1000.000000000000000 ) ;
#17928=ORIENTED_EDGE ( 'NONE', *, *, #6327, .T. ) ;
#17932=EDGE_CURVE ( 'NONE', #17877, #3870, #22950, .T. ) ;
#17933=CARTESIAN_POINT ( 'NONE',  ( 8.250000000000000000, -40.23606797749999942, -150.0552959529999839 ) ) ;
#17934=CARTESIAN_POINT ( 'NONE',  ( -32.50000000000000000, -51.50000000000000000, -142.8052959529999839 ) ) ;
#17937=VECTOR ( 'NONE', #22516, 1000.000000000000000 ) ;
#17943=PLANE ( 'NONE',  #4425 ) ;
#17946=ORIENTED_EDGE ( 'NONE', *, *, #9808, .T. ) ;
#17949=ORIENTED_EDGE ( 'NONE', *, *, #15210, .T. ) ;
#17955=ORIENTED_EDGE ( 'NONE', *, *, #19756, .T. ) ;
#17960=CARTESIAN_POINT ( 'NONE',  ( 24.97526911139999939, -44.90215078659999648, -151.0552959529999839 ) ) ;
#17962=CARTESIAN_POINT ( 'NONE',  ( 6.000000000000000000, -3.500000000000000000, -145.5552959529999839 ) ) ;
#17963=EDGE_CURVE ( 'NONE', #13650, #19480, #15798, .T. ) ;
#17970=EDGE_LOOP ( 'NONE', ( #6415, #16587, #16950, #16095, #11138, #14708, #13632, #2651, #15564, #10719, #18353, #8035, #21261, #8084, #3566 ) ) ;
#17988=VERTEX_POINT ( 'NONE', #8418 ) ;
#17994=CARTESIAN_POINT ( 'NONE',  ( -3.500000000000000000, 46.50000000000000000, -150.0552959529999839 ) ) ;
#17998=CARTESIAN_POINT ( 'NONE',  ( 31.32297112069999656, -40.18599471579999971, -149.5552959529999839 ) ) ;
#18010=ORIENTED_EDGE ( 'NONE', *, *, #21448, .T. ) ;
#18011=LINE ( 'NONE', #1836, #1991 ) ;
#18013=CARTESIAN_POINT ( 'NONE',  ( 32.50000000000000000, -40.03620104880000241, -136.0552959519999945 ) ) ;
#18015=DIRECTION ( 'NONE',  ( 0.000000000000000000, 0.000000000000000000, 1.000000000000000000 ) ) ;
#18022=FACE_OUTER_BOUND ( 'NONE', #9492, .T. ) ;
#18033=ADVANCED_FACE ( 'NONE', ( #12691, #3302 ), #8990, .T. ) ;
#18034=ORIENTED_EDGE ( 'NONE', *, *, #22626, .T. ) ;
#18037=LINE ( 'NONE', #1748, #22467 ) ;
#18049=EDGE_CURVE ( 'NONE', #4360, #17493, #16275, .T. ) ;
#18053=DIRECTION ( 'NONE',  ( 1.000000000000000000, 0.000000000000000000, 0.000000000000000000 ) ) ;
#18059=CARTESIAN_POINT ( 'NONE',  ( 26.42191803000496009, -21.28524365307783484, -150.0552959530000123 ) ) ;
#18060=ORIENTED_EDGE ( 'NONE', *, *, #10734, .T. ) ;
#18083=LINE ( 'NONE', #9015, #20132 ) ;
#18084=VERTEX_POINT ( 'NONE', #6990 ) ;
#18091=VECTOR ( 'NONE', #23324, 1000.000000000000000 ) ;
#18092=EDGE_CURVE ( 'NONE', #3905, #21024, #16158, .T. ) ;
#18097=CARTESIAN_POINT ( 'NONE',  ( 2.656359840075261047, -5.899000527194546706, -150.0552959529999839 ) ) ;
#18102=ADVANCED_FACE ( 'NONE', ( #14493 ), #17943, .T. ) ;
#18103=CARTESIAN_POINT ( 'NONE',  ( -31.75000000000000000, 1.000000000000000000, -151.0552959529999839 ) ) ;
#18108=LINE ( 'NONE', #16327, #15159 ) ;
#18111=EDGE_CURVE ( 'NONE', #22981, #7563, #16392, .T. ) ;
#18112=CARTESIAN_POINT ( 'NONE',  ( -32.50000000000000000, 48.75000000000000000, -151.0552959529999839 ) ) ;
#18131=EDGE_LOOP ( 'NONE', ( #5339, #15463, #11149, #3705 ) ) ;
#18132=ADVANCED_FACE ( 'NONE', ( #15871 ), #3160, .T. ) ;
#18139=DIRECTION ( 'NONE',  ( 1.000000000000000000, 0.000000000000000000, 0.000000000000000000 ) ) ;
#18146=DIRECTION ( 'NONE',  ( 0.000000000000000000, -1.000000000000000000, 1.723073263340000007E-12 ) ) ;
#18152=EDGE_LOOP ( 'NONE', ( #15632, #10883, #11158, #20764 ) ) ;
#18156=CARTESIAN_POINT ( 'NONE',  ( -6.719053507402335867, 25.42349012523258267, -150.0552959530000123 ) ) ;
#18160=CARTESIAN_POINT ( 'NONE',  ( -32.50000000000000000, -50.00000000000000000, -143.3052959529999839 ) ) ;
#18168=ORIENTED_EDGE ( 'NONE', *, *, #18257, .F. ) ;
#18174=DIRECTION ( 'NONE',  ( 1.000000000000000000, 0.000000000000000000, 0.000000000000000000 ) ) ;
#18175=ORIENTED_EDGE ( 'NONE', *, *, #12272, .F. ) ;
#18179=CARTESIAN_POINT ( 'NONE',  ( 19.45666326950000169, -50.88169314249999786, -149.5552959529999839 ) ) ;
#18190=DIRECTION ( 'NONE',  ( -0.7633862853691523176, -0.6459422414661291079, 0.000000000000000000 ) ) ;
#18194=EDGE_CURVE ( 'NONE', #19589, #18962, #17776, .T. ) ;
#18196=VECTOR ( 'NONE', #18527, 1000.000000000000000 ) ;
#18197=EDGE_CURVE ( 'NONE', #258, #23250, #15762, .T. ) ;
#18209=CARTESIAN_POINT ( 'NONE',  ( 32.50000000000000000, -33.03620104880000241, -136.5552959530000123 ) ) ;
#18213=CARTESIAN_POINT ( 'NONE',  ( 4.750000000000000000, -38.23606797749999942, -150.0552959529999839 ) ) ;
#18214=VECTOR ( 'NONE', #17863, 1000.000000000000000 ) ;
#18216=AXIS2_PLACEMENT_3D ( 'NONE', #6453, #15618, #6799 ) ;
#18217=DIRECTION ( 'NONE',  ( 0.000000000000000000, 0.000000000000000000, 1.000000000000000000 ) ) ;
#18222=DIRECTION ( 'NONE',  ( 1.000000000000000000, 0.000000000000000000, 0.000000000000000000 ) ) ;
#18225=VECTOR ( 'NONE', #18369, 1000.000000000000000 ) ;
#18227=ADVANCED_FACE ( 'NONE', ( #4937 ), #12183, .F. ) ;
#18230=VECTOR ( 'NONE', #11142, 1000.000000000000000 ) ;
#18233=AXIS2_PLACEMENT_3D ( 'NONE', #16763, #7481, #22130 ) ;
#18249=AXIS2_PLACEMENT_3D ( 'NONE', #17658, #21471, #18015 ) ;
#18256=DIRECTION ( 'NONE',  ( 0.000000000000000000, 0.000000000000000000, 1.000000000000000000 ) ) ;
#18257=EDGE_CURVE ( 'NONE', #7545, #20852, #8833, .T. ) ;
#18258=B_SPLINE_CURVE_WITH_KNOTS ( 'NONE', 3,
 ( #21577, #6810, #5259, #14077, #5037, #3140, #13841, #22894, #23238, #8695, #19190, #17646, #19552, #6692, #12388, #2900, #13951, #15628 ),
 .UNSPECIFIED., .F., .F.,
 ( 4, 2, 2, 2, 2, 2, 2, 2, 4 ),
 ( 0.000000000000000000, 0.1250000000000000000, 0.2500000000000000000, 0.3750000000000000000, 0.5000000000000000000, 0.6250000000000000000, 0.7500000000000000000, 0.8750000000000000000, 1.000000000000000000 ),
 .UNSPECIFIED. ) ;
#18259=CARTESIAN_POINT ( 'NONE',  ( 8.750000000000000000, -44.61803398880000060, -151.0552959529999839 ) ) ;
#18262=DIRECTION ( 'NONE',  ( -1.457881434619999915E-12, 1.723066134219999902E-12, 1.000000000000000000 ) ) ;
#18263=CARTESIAN_POINT ( 'NONE',  ( 15.50000000000000000, 33.50000000000000000, -150.0552959529999839 ) ) ;
#18266=VECTOR ( 'NONE', #16771, 1000.000000000000000 ) ;
#18267=CARTESIAN_POINT ( 'NONE',  ( 3.552713678799999608E-15, 50.00000000000000000, -149.5552959529999839 ) ) ;
#18269=EDGE_CURVE ( 'NONE', #16883, #1705, #10803, .T. ) ;
#18277=ORIENTED_EDGE ( 'NONE', *, *, #12566, .F. ) ;
#18278=DIRECTION ( 'NONE',  ( 0.000000000000000000, 0.000000000000000000, 1.000000000000000000 ) ) ;
#18280=VERTEX_POINT ( 'NONE', #12884 ) ;
#18283=ADVANCED_FACE ( 'NONE', ( #5746 ), #12530, .F. ) ;
#18287=FACE_OUTER_BOUND ( 'NONE', #12928, .T. ) ;
#18296=LINE ( 'NONE', #14709, #22735 ) ;
#18297=CIRCLE ( 'NONE', #12971, 7.499999999999999112 ) ;
#18298=ORIENTED_EDGE ( 'NONE', *, *, #20170, .T. ) ;
#18309=CARTESIAN_POINT ( 'NONE',  ( -7.500000000000000000, 25.50000000000000000, -151.0552959529999839 ) ) ;
#18312=FACE_OUTER_BOUND ( 'NONE', #14620, .T. ) ;
#18318=LINE ( 'NONE', #9475, #19747 ) ;
#18321=CARTESIAN_POINT ( 'NONE',  ( -31.75000000030000180, -51.50000000000000000, -149.5552959529999839 ) ) ;
#18326=CARTESIAN_POINT ( 'NONE',  ( -6.683153925719999222, 51.50000000000000000, -136.0552959530000123 ) ) ;
#18327=FACE_BOUND ( 'NONE', #4710, .T. ) ;
#18332=ORIENTED_EDGE ( 'NONE', *, *, #6691, .T. ) ;
#18343=DIRECTION ( 'NONE',  ( 0.000000000000000000, -3.386627385143914456E-17, -1.000000000000000000 ) ) ;
#18348=VECTOR ( 'NONE', #752, 1000.000000000000000 ) ;
#18350=CARTESIAN_POINT ( 'NONE',  ( 1.133692148550000001, -51.00000000000000000, -136.0552959530000123 ) ) ;
#18352=DIRECTION ( 'NONE',  ( 0.000000000000000000, -1.000000000000000000, 0.000000000000000000 ) ) ;
#18353=ORIENTED_EDGE ( 'NONE', *, *, #5237, .F. ) ;
#18356=CARTESIAN_POINT ( 'NONE',  ( -31.00000000000000000, 19.50000000000000000, -151.0552959529999839 ) ) ;
#18358=CARTESIAN_POINT ( 'NONE',  ( -13.86630785140000022, -50.50000000000000000, -136.0552959530000123 ) ) ;
#18369=DIRECTION ( 'NONE',  ( 0.000000000000000000, -1.000000000000000000, 0.000000000000000000 ) ) ;
#18373=CARTESIAN_POINT ( 'NONE',  ( -32.50000000000000000, 19.50000000000000000, -143.3052959529999839 ) ) ;
#18375=DIRECTION ( 'NONE',  ( 1.000000000000000000, 0.000000000000000000, 2.257144641399999941E-12 ) ) ;
#18377=EDGE_CURVE ( 'NONE', #13765, #751, #9067, .T. ) ;
#18381=ORIENTED_EDGE ( 'NONE', *, *, #23008, .F. ) ;
#18382=VERTEX_POINT ( 'NONE', #16236 ) ;
#18384=CARTESIAN_POINT ( 'NONE',  ( 13.13369214859999978, 51.50000000000000000, -136.5552959530000123 ) ) ;
#18390=CARTESIAN_POINT ( 'NONE',  ( 8.750000000000000000, -42.23606797749999942, -150.0552959529999839 ) ) ;
#18397=CARTESIAN_POINT ( 'NONE',  ( 18.95053822279999878, 50.00000000000000000, -151.0552959529999839 ) ) ;
#18398=ORIENTED_EDGE ( 'NONE', *, *, #11820, .F. ) ;
#18402=ORIENTED_EDGE ( 'NONE', *, *, #16197, .F. ) ;
#18403=LINE ( 'NONE', #2113, #15518 ) ;
#18405=ORIENTED_EDGE ( 'NONE', *, *, #5639, .F. ) ;
#18410=ADVANCED_FACE ( 'NONE', ( #20479 ), #7502, .F. ) ;
#18412=PLANE ( 'NONE',  #9431 ) ;
#18418=CARTESIAN_POINT ( 'NONE',  ( 13.00952979661476583, 24.25756286942641538, -150.0552959529999839 ) ) ;
#18429=EDGE_CURVE ( 'NONE', #12791, #11661, #501, .T. ) ;
#18438=PLANE ( 'NONE',  #12859 ) ;
#18440=EDGE_LOOP ( 'NONE', ( #10540, #3131, #1307, #18793 ) ) ;
#18451=VERTEX_POINT ( 'NONE', #14766 ) ;
#18461=VECTOR ( 'NONE', #18262, 1000.000000000000000 ) ;
#18463=PLANE ( 'NONE',  #18532 ) ;
#18474=EDGE_LOOP ( 'NONE', ( #11109, #11197, #2206, #7800 ) ) ;
#18475=CARTESIAN_POINT ( 'NONE',  ( 7.500000000000000000, -3.500000000000000000, -140.0552959529999839 ) ) ;
#18481=LINE ( 'NONE', #5283, #6680 ) ;
#18482=CARTESIAN_POINT ( 'NONE',  ( 12.57628698940784773, 35.71923945895441221, -150.0552959529999839 ) ) ;
#18487=ORIENTED_EDGE ( 'NONE', *, *, #17167, .F. ) ;
#18489=LINE ( 'NONE', #20639, #13648 ) ;
#18491=ORIENTED_EDGE ( 'NONE', *, *, #17380, .F. ) ;
#18498=CYLINDRICAL_SURFACE ( 'NONE', #7156, 1.500000000000000444 ) ;
#18507=DIRECTION ( 'NONE',  ( 0.6459422414661299960, 0.7633862853691516515, 0.000000000000000000 ) ) ;
#18508=ORIENTED_EDGE ( 'NONE', *, *, #19567, .F. ) ;
#18515=VECTOR ( 'NONE', #3513, 1000.000000000000000 ) ;
#18517=DIRECTION ( 'NONE',  ( 0.000000000000000000, 0.000000000000000000, 1.000000000000000000 ) ) ;
#18527=DIRECTION ( 'NONE',  ( 1.000000000000000000, 0.000000000000000000, 0.000000000000000000 ) ) ;
#18530=DIRECTION ( 'NONE',  ( 0.000000000000000000, 0.000000000000000000, 1.000000000000000000 ) ) ;
#18532=AXIS2_PLACEMENT_3D ( 'NONE', #13099, #4190, #11424 ) ;
#18534=EDGE_CURVE ( 'NONE', #3203, #18084, #15243, .T. ) ;
#18535=CIRCLE ( 'NONE', #8264, 0.5000000000000004441 ) ;
#18537=LINE ( 'NONE', #9920, #8602 ) ;
#18542=DIRECTION ( 'NONE',  ( 0.000000000000000000, -1.000000000000000000, 0.000000000000000000 ) ) ;
#18547=EDGE_LOOP ( 'NONE', ( #4029, #21921, #11152, #10705 ) ) ;
#18548=FACE_OUTER_BOUND ( 'NONE', #22339, .T. ) ;
#18551=EDGE_LOOP ( 'NONE', ( #9423, #5926, #9703, #21881, #18911, #20034, #2491, #4472, #8578, #499, #3563 ) ) ;
#18553=CARTESIAN_POINT ( 'NONE',  ( -24.00000000000000000, 47.50000000000000000, -151.0552959529999839 ) ) ;
#18558=AXIS2_PLACEMENT_3D ( 'NONE', #3301, #10537, #17820 ) ;
#18570=VECTOR ( 'NONE', #3183, 1000.000000000000000 ) ;
#18572=CYLINDRICAL_SURFACE ( 'NONE', #8246, 0.5000000000000079936 ) ;
#18577=AXIS2_PLACEMENT_3D ( 'NONE', #10512, #1634, #10403 ) ;
#18578=DIRECTION ( 'NONE',  ( 0.6459422414661314393, -0.7633862853691505412, 0.000000000000000000 ) ) ;
#18580=VECTOR ( 'NONE', #1077, 1000.000000000000227 ) ;
#18589=EDGE_CURVE ( 'NONE', #1386, #13765, #19400, .T. ) ;
#18598=CIRCLE ( 'NONE', #10229, 1.500000000000001332 ) ;
#18604=CARTESIAN_POINT ( 'NONE',  ( 13.66060904159877154, 34.09818317339773586, -150.0552959529999839 ) ) ;
#18606=DIRECTION ( 'NONE',  ( -1.457881434619999915E-12, -1.723066134219999902E-12, 1.000000000000000000 ) ) ;
#18607=VECTOR ( 'NONE', #10059, 1000.000000000000000 ) ;
#18608=CARTESIAN_POINT ( 'NONE',  ( 3.906463970568107236, -37.00246044238615184, -150.0552959529999839 ) ) ;
#18610=VECTOR ( 'NONE', #455, 1000.000000000000000 ) ;
#18611=VECTOR ( 'NONE', #4453, 1000.000000000000000 ) ;
#18613=ORIENTED_EDGE ( 'NONE', *, *, #21600, .F. ) ;
#18615=AXIS2_PLACEMENT_3D ( 'NONE', #3221, #7018, #10345 ) ;
#18620=CARTESIAN_POINT ( 'NONE',  ( -31.00000000000000000, -7.105427357599999217E-15, -149.5552959529999839 ) ) ;
#18622=EDGE_LOOP ( 'NONE', ( #9234, #7256, #7325, #13008 ) ) ;
#18634=ORIENTED_EDGE ( 'NONE', *, *, #7700, .F. ) ;
#18635=DIRECTION ( 'NONE',  ( 0.000000000000000000, 1.000000000000000000, 0.000000000000000000 ) ) ;
#18636=ORIENTED_EDGE ( 'NONE', *, *, #17652, .F. ) ;
#18640=VERTEX_POINT ( 'NONE', #12007 ) ;
#18648=ORIENTED_EDGE ( 'NONE', *, *, #13640, .T. ) ;
#18651=CARTESIAN_POINT ( 'NONE',  ( 6.992624432235133192, 28.00000000000000711, -150.0552959530000408 ) ) ;
#18652=EDGE_CURVE ( 'NONE', #12670, #6404, #19934, .T. ) ;
#18654=DIRECTION ( 'NONE',  ( -0.6459422414661292189, 0.7633862853691524286, 0.000000000000000000 ) ) ;
#18671=CARTESIAN_POINT ( 'NONE',  ( -3.500000000000000000, 40.00000000000000000, -150.0552959529999839 ) ) ;
#18672=ADVANCED_FACE ( 'NONE', ( #13556 ), #11762, .T. ) ;
#18673=EDGE_LOOP ( 'NONE', ( #17572, #14477, #12311, #7550 ) ) ;
#18674=LINE ( 'NONE', #2496, #20900 ) ;
#18679=ORIENTED_EDGE ( 'NONE', *, *, #11430, .T. ) ;
#18695=ADVANCED_FACE ( 'NONE', ( #16179 ), #12471, .T. ) ;
#18700=DIRECTION ( 'NONE',  ( -1.000000000000000000, 0.000000000000000000, -2.245315044929999938E-12 ) ) ;
#18702=VERTEX_POINT ( 'NONE', #8544 ) ;
#18713=ADVANCED_FACE ( 'NONE', ( #3213 ), #19628, .T. ) ;
#18717=CARTESIAN_POINT ( 'NONE',  ( 15.50000000000000000, 33.50000000000000000, -151.0552959529999839 ) ) ;
#18719=VERTEX_POINT ( 'NONE', #10337 ) ;
#18721=FACE_BOUND ( 'NONE', #21421, .T. ) ;
#18722=ORIENTED_EDGE ( 'NONE', *, *, #14743, .F. ) ;
#18724=CARTESIAN_POINT ( 'NONE',  ( 32.14594224169999848, -40.79958733389999992, -150.0552959529999839 ) ) ;
#18735=EDGE_CURVE ( 'NONE', #18822, #9410, #8781, .T. ) ;
#18749=CARTESIAN_POINT ( 'NONE',  ( -25.86630785139999844, -50.50000000000000000, -137.0552959530000123 ) ) ;
#18750=DIRECTION ( 'NONE',  ( 0.000000000000000000, -4.253943788710456142E-15, -1.000000000000000000 ) ) ;
#18760=ORIENTED_EDGE ( 'NONE', *, *, #14743, .T. ) ;
#18761=CARTESIAN_POINT ( 'NONE',  ( -17.92191803000494588, -43.78524365307784905, -150.0552959529999839 ) ) ;
#18769=LINE ( 'NONE', #7582, #18196 ) ;
#18770=ORIENTED_EDGE ( 'NONE', *, *, #20825, .F. ) ;
#18771=FACE_OUTER_BOUND ( 'NONE', #11875, .T. ) ;
#18778=DIRECTION ( 'NONE',  ( 0.000000000000000000, 1.000000000000000000, 0.000000000000000000 ) ) ;
#18783=DIRECTION ( 'NONE',  ( -1.000000000000000000, 0.000000000000000000, 2.257453483404482811E-12 ) ) ;
#18788=DIRECTION ( 'NONE',  ( -2.257144641399999941E-12, 0.000000000000000000, -1.000000000000000000 ) ) ;
#18793=ORIENTED_EDGE ( 'NONE', *, *, #17903, .F. ) ;
#18796=LINE ( 'NONE', #15106, #19369 ) ;
#18797=VERTEX_POINT ( 'NONE', #19872 ) ;
#18800=ORIENTED_EDGE ( 'NONE', *, *, #4547, .F. ) ;
#18802=B_SPLINE_CURVE_WITH_KNOTS ( 'NONE', 3,
 ( #22335, #18651, #14723, #9588, #21990, #16861, #5681, #12937, #4253, #11489, #3910, #18418, #2126, #16621, #331, #7577, #14852, #22109 ),
 .UNSPECIFIED., .F., .F.,
 ( 4, 2, 2, 2, 2, 2, 2, 2, 4 ),
 ( 0.000000000000000000, 0.1249999999999998057, 0.2499999999999998335, 0.3749999999999998335, 0.4999999999999998890, 0.6249999999999998890, 0.7499999999999998890, 0.8750000000000000000, 1.000000000000000000 ),
 .UNSPECIFIED. ) ;
#18803=VERTEX_POINT ( 'NONE', #14033 ) ;
#18806=CARTESIAN_POINT ( 'NONE',  ( 23.50000000000000000, -20.50000000000000000, -136.0552959530000123 ) ) ;
#18812=LINE ( 'NONE', #21081, #9025 ) ;
#18813=DIRECTION ( 'NONE',  ( 0.000000000000000000, 0.000000000000000000, 1.000000000000000000 ) ) ;
#18818=EDGE_CURVE ( 'NONE', #23189, #6609, #20771, .T. ) ;
#18822=VERTEX_POINT ( 'NONE', #5691 ) ;
#18824=LINE ( 'NONE', #11787, #11873 ) ;
#18825=ORIENTED_EDGE ( 'NONE', *, *, #5568, .T. ) ;
#18830=AXIS2_PLACEMENT_3D ( 'NONE', #1852, #16578, #7310 ) ;
#18841=VERTEX_POINT ( 'NONE', #1914 ) ;
#18844=AXIS2_PLACEMENT_3D ( 'NONE', #239, #7135, #14278 ) ;
#18845=DIRECTION ( 'NONE',  ( 0.000000000000000000, 0.000000000000000000, 1.000000000000000000 ) ) ;
#18855=EDGE_CURVE ( 'NONE', #2146, #8510, #16416, .T. ) ;
#18857=EDGE_CURVE ( 'NONE', #21113, #11661, #18537, .T. ) ;
#18858=DIRECTION ( 'NONE',  ( -1.000000000000000000, 0.000000000000000000, 0.000000000000000000 ) ) ;
#18859=FACE_OUTER_BOUND ( 'NONE', #18131, .T. ) ;
#18866=ORIENTED_EDGE ( 'NONE', *, *, #23008, .T. ) ;
#18879=DIRECTION ( 'NONE',  ( 2.257144641399999941E-12, 0.000000000000000000, -1.000000000000000000 ) ) ;
#18882=ORIENTED_EDGE ( 'NONE', *, *, #10349, .F. ) ;
#18888=VECTOR ( 'NONE', #9195, 1000.000000000000227 ) ;
#18890=CARTESIAN_POINT ( 'NONE',  ( -3.500000000000000000, 44.50000000000000000, -151.0552959529999839 ) ) ;
#18892=ORIENTED_EDGE ( 'NONE', *, *, #668, .F. ) ;
#18893=CARTESIAN_POINT ( 'NONE',  ( 6.500000000000000000, 28.00000000000000000, -150.0552959529999839 ) ) ;
#18897=ORIENTED_EDGE ( 'NONE', *, *, #3451, .T. ) ;
#18899=APPLICATION_CONTEXT ( 'automotive_design' ) ;
#18901=EDGE_LOOP ( 'NONE', ( #17064, #1831, #11632, #1993 ) ) ;
#18904=CARTESIAN_POINT ( 'NONE',  ( 6.500000000000000000, 20.50000000000000000, -150.0552959529999839 ) ) ;
#18906=CARTESIAN_POINT ( 'NONE',  ( -25.86630785139999844, -51.50000000000000000, -136.0552959530000123 ) ) ;
#18911=ORIENTED_EDGE ( 'NONE', *, *, #17375, .F. ) ;
#18912=ADVANCED_FACE ( 'NONE', ( #7471 ), #5577, .T. ) ;
#18919=CARTESIAN_POINT ( 'NONE',  ( 1.499999999999999112, -3.107300918301282522, -150.0552959529999839 ) ) ;
#18920=B_SPLINE_CURVE_WITH_KNOTS ( 'NONE', 3,
 ( #20688, #17229, #4383, #15335, #2839, #10069, #17347, #22592, #6281, #13535, #8292, #15566, #3426, #23298, #6872, #18059, #17823, #1540 ),
 .UNSPECIFIED., .F., .F.,
 ( 4, 2, 2, 2, 2, 2, 2, 2, 4 ),
 ( 0.000000000000000000, 0.1250000000000000000, 0.2500000000000000000, 0.3750000000000000000, 0.5000000000000000000, 0.6250000000000000000, 0.7500000000000000000, 0.8750000000000000000, 1.000000000000000000 ),
 .UNSPECIFIED. ) ;
#18923=DIRECTION ( 'NONE',  ( -2.257242012349999735E-12, 0.000000000000000000, 1.000000000000000000 ) ) ;
#18932=CARTESIAN_POINT ( 'NONE',  ( 19.13369214859999801, -51.50000000000000000, -143.0552959529999839 ) ) ;
#18940=CARTESIAN_POINT ( 'NONE',  ( 19.13369214859999801, -50.50000000000000000, -136.0552959530000123 ) ) ;
#18952=DIRECTION ( 'NONE',  ( -1.000000000000000000, 0.000000000000000000, 2.257144641399999941E-12 ) ) ;
#18955=DIRECTION ( 'NONE',  ( 0.7633862853691523176, -0.6459422414661291079, 0.000000000000000000 ) ) ;
#18957=ORIENTED_EDGE ( 'NONE', *, *, #21161, .T. ) ;
#18962=VERTEX_POINT ( 'NONE', #22003 ) ;
#18967=EDGE_CURVE ( 'NONE', #16505, #23292, #23010, .T. ) ;
#18972=ORIENTED_EDGE ( 'NONE', *, *, #4567, .T. ) ;
#18973=CARTESIAN_POINT ( 'NONE',  ( 23.50000000000000000, -20.50000000000000000, -136.0552959530000123 ) ) ;
#18978=EDGE_CURVE ( 'NONE', #11661, #11512, #6345, .T. ) ;
#18981=EDGE_CURVE ( 'NONE', #19891, #16708, #4823, .T. ) ;
#18986=ORIENTED_EDGE ( 'NONE', *, *, #9948, .T. ) ;
#18998=ORIENTED_EDGE ( 'NONE', *, *, #20825, .T. ) ;
#18999=CYLINDRICAL_SURFACE ( 'NONE', #5683, 2.999999999999999112 ) ;
#19005=DIRECTION ( 'NONE',  ( 0.000000000000000000, 1.000000000000000000, -2.245315044999999693E-12 ) ) ;
#19008=FACE_OUTER_BOUND ( 'NONE', #18551, .T. ) ;
#19010=CARTESIAN_POINT ( 'NONE',  ( 25.42371301058693689, 37.28076054106433901, -150.0552959529999839 ) ) ;
#19011=ORIENTED_EDGE ( 'NONE', *, *, #2138, .F. ) ;
#19014=ORIENTED_EDGE ( 'NONE', *, *, #5889, .T. ) ;
#19015=DIRECTION ( 'NONE',  ( -1.000000000000000000, 0.000000000000000000, 0.000000000000000000 ) ) ;
#19031=CARTESIAN_POINT ( 'NONE',  ( -7.500000000000000000, 19.50000000000000000, -150.0552959529999839 ) ) ;
#19036=AXIS2_PLACEMENT_3D ( 'NONE', #12799, #20310, #16271 ) ;
#19043=ORIENTED_EDGE ( 'NONE', *, *, #8899, .T. ) ;
#19047=DIRECTION ( 'NONE',  ( 0.000000000000000000, -2.252420471819999940E-12, 1.000000000000000000 ) ) ;
#19052=VECTOR ( 'NONE', #12166, 1000.000000000000227 ) ;
#19055=DIRECTION ( 'NONE',  ( 0.000000000000000000, 0.000000000000000000, 1.000000000000000000 ) ) ;
#19058=CARTESIAN_POINT ( 'NONE',  ( -10.00000000000000000, 48.50000000000000000, -151.0552959529999839 ) ) ;
#19063=CARTESIAN_POINT ( 'NONE',  ( -25.86630785139999844, -50.50000000000000000, -137.0552959530000123 ) ) ;
#19066=CARTESIAN_POINT ( 'NONE',  ( 19.13369214859999801, 51.50000000000000000, -149.5552959529999839 ) ) ;
#19067=CARTESIAN_POINT ( 'NONE',  ( -13.86630785140000022, 50.50000000000000000, -142.8052959529999839 ) ) ;
#19076=DIRECTION ( 'NONE',  ( 0.000000000000000000, -1.000000000000000000, 0.000000000000000000 ) ) ;
#19080=CARTESIAN_POINT ( 'NONE',  ( 9.444192711117707972, -34.64608312524905642, -150.0552959529999555 ) ) ;
#19083=ADVANCED_FACE ( 'NONE', ( #19928 ), #5414, .F. ) ;
#19091=PLANE ( 'NONE',  #23187 ) ;
#19094=DIRECTION ( 'NONE',  ( 0.000000000000000000, -1.000000000000000000, 2.257144641399999941E-12 ) ) ;
#19098=DIRECTION ( 'NONE',  ( 1.000000000000000000, -2.312964634635743450E-15, 0.000000000000000000 ) ) ;
#19100=CARTESIAN_POINT ( 'NONE',  ( 6.000000000000000000, -3.500000000000000000, -150.0552959529999839 ) ) ;
#19103=CARTESIAN_POINT ( 'NONE',  ( -2.500000000000000000, 37.00000000000000000, -151.0552959529999839 ) ) ;
#19105=ORIENTED_EDGE ( 'NONE', *, *, #6442, .T. ) ;
#19108=FACE_OUTER_BOUND ( 'NONE', #18547, .T. ) ;
#19112=ORIENTED_EDGE ( 'NONE', *, *, #18652, .T. ) ;
#19114=ADVANCED_FACE ( 'NONE', ( #3384 ), #12660, .F. ) ;
#19124=ADVANCED_FACE ( 'NONE', ( #23380 ), #7075, .F. ) ;
#19126=EDGE_LOOP ( 'NONE', ( #726, #19014, #18613, #15866 ) ) ;
#19130=DIRECTION ( 'NONE',  ( 1.000000000000000000, 0.000000000000000000, -2.257453483404482811E-12 ) ) ;
#19142=ORIENTED_EDGE ( 'NONE', *, *, #20869, .F. ) ;
#19145=DIRECTION ( 'NONE',  ( 0.000000000000000000, 0.000000000000000000, 1.000000000000000000 ) ) ;
#19151=DIRECTION ( 'NONE',  ( 1.000000000000000000, 0.000000000000000000, 0.000000000000000000 ) ) ;
#19160=EDGE_LOOP ( 'NONE', ( #21342, #1280, #2382, #1632 ) ) ;
#19174=ORIENTED_EDGE ( 'NONE', *, *, #2755, .T. ) ;
#19182=LINE ( 'NONE', #2893, #4541 ) ;
#19190=CARTESIAN_POINT ( 'NONE',  ( 1.924079216156750372, 26.46241645103150475, -150.0552959529999839 ) ) ;
#19192=VERTEX_POINT ( 'NONE', #20172 ) ;
#19207=EDGE_CURVE ( 'NONE', #6404, #8234, #9072, .T. ) ;
#19209=LINE ( 'NONE', #2920, #5536 ) ;
#19217=CIRCLE ( 'NONE', #618, 2.999999999999999112 ) ;
#19224=VERTEX_POINT ( 'NONE', #8845 ) ;
#19225=ORIENTED_EDGE ( 'NONE', *, *, #12168, .T. ) ;
#19226=DIRECTION ( 'NONE',  ( 0.000000000000000000, -1.000000000000000000, 0.000000000000000000 ) ) ;
#19233=DIRECTION ( 'NONE',  ( 0.000000000000000000, 2.257144641399999941E-12, -1.000000000000000000 ) ) ;
#19235=EDGE_CURVE ( 'NONE', #2055, #12686, #3863, .T. ) ;
#19237=CARTESIAN_POINT ( 'NONE',  ( -31.75000000000000000, 1.000000000000000000, -150.0552959529999839 ) ) ;
#19238=CARTESIAN_POINT ( 'NONE',  ( 24.33939095839631861, 38.90181682659950724, -150.0552959529999839 ) ) ;
#19239=EDGE_LOOP ( 'NONE', ( #8141, #17949, #7935, #3893 ) ) ;
#19241=FACE_OUTER_BOUND ( 'NONE', #6703, .T. ) ;
#19246=DIRECTION ( 'NONE',  ( 1.000000000000000000, 0.000000000000000000, 0.000000000000000000 ) ) ;
#19254=EDGE_CURVE ( 'NONE', #18797, #2028, #3743, .T. ) ;
#19255=CARTESIAN_POINT ( 'NONE',  ( -2.500000000000000000, 37.00000000000000000, -150.0552959529999839 ) ) ;
#19258=ADVANCED_FACE ( 'NONE', ( #14805 ), #13239, .F. ) ;
#19260=ORIENTED_EDGE ( 'NONE', *, *, #12218, .T. ) ;
#19261=CARTESIAN_POINT ( 'NONE',  ( -32.50000000000000000, 50.50000000000000000, -137.0552959530000123 ) ) ;
#19267=ORIENTED_EDGE ( 'NONE', *, *, #21861, .F. ) ;
#19270=ORIENTED_EDGE ( 'NONE', *, *, #13448, .F. ) ;
#19271=CARTESIAN_POINT ( 'NONE',  ( 6.343640159924743394, -1.100999472805458401, -150.0552959529999839 ) ) ;
#19277=DIRECTION ( 'NONE',  ( -1.000000000000000000, 0.000000000000000000, 0.000000000000000000 ) ) ;
#19280=DIRECTION ( 'NONE',  ( 0.000000000000000000, 0.000000000000000000, 1.000000000000000000 ) ) ;
#19281=CARTESIAN_POINT ( 'NONE',  ( -14.80142434073996860, -41.50006722989636643, -150.0552959529999839 ) ) ;
#19287=EDGE_CURVE ( 'NONE', #14651, #7053, #7765, .T. ) ;
#19288=FACE_OUTER_BOUND ( 'NONE', #604, .T. ) ;
#19292=CARTESIAN_POINT ( 'NONE',  ( 13.13369214859999978, -50.50000000000000000, -136.0552959530000123 ) ) ;
#19299=VERTEX_POINT ( 'NONE', #11450 ) ;
#19302=DIRECTION ( 'NONE',  ( 1.000000000000000000, 0.000000000000000000, 0.000000000000000000 ) ) ;
#19303=EDGE_LOOP ( 'NONE', ( #15859, #8021, #7942, #4988 ) ) ;
#19305=DIRECTION ( 'NONE',  ( 2.257144641399999941E-12, 0.000000000000000000, 1.000000000000000000 ) ) ;
#19316=ADVANCED_FACE ( 'NONE', ( #13363 ), #22292, .T. ) ;
#19317=EDGE_CURVE ( 'NONE', #16851, #954, #11066, .T. ) ;
#19318=ORIENTED_EDGE ( 'NONE', *, *, #8608, .T. ) ;
#19322=AXIS2_PLACEMENT_3D ( 'NONE', #14825, #9884, #12908 ) ;
#19329=AXIS2_PLACEMENT_3D ( 'NONE', #2027, #14154, #7004 ) ;
#19331=CARTESIAN_POINT ( 'NONE',  ( -16.51085694111269930, -40.37864083493722234, -150.0552959529999555 ) ) ;
#19334=DIRECTION ( 'NONE',  ( 0.000000000000000000, 1.000000000000000000, 0.000000000000000000 ) ) ;
#19336=CARTESIAN_POINT ( 'NONE',  ( -13.86630785140000022, 51.00000000000000000, -137.0552959530000123 ) ) ;
#19340=ORIENTED_EDGE ( 'NONE', *, *, #21868, .F. ) ;
#19345=ORIENTED_EDGE ( 'NONE', *, *, #20704, .F. ) ;
#19347=AXIS2_PLACEMENT_3D ( 'NONE', #7469, #14732, #3679 ) ;
#19351=ADVANCED_FACE ( 'NONE', ( #533 ), #5866, .F. ) ;
#19364=VECTOR ( 'NONE', #13165, 1000.000000000000227 ) ;
#19369=VECTOR ( 'NONE', #4396, 1000.000000000000000 ) ;
#19375=FACE_OUTER_BOUND ( 'NONE', #17785, .T. ) ;
#19379=ORIENTED_EDGE ( 'NONE', *, *, #952, .T. ) ;
#19387=EDGE_LOOP ( 'NONE', ( #17017, #4444 ) ) ;
#19392=ORIENTED_EDGE ( 'NONE', *, *, #17087, .T. ) ;
#19398=ORIENTED_EDGE ( 'NONE', *, *, #20348, .F. ) ;
#19400=LINE ( 'NONE', #9738, #7461 ) ;
#19414=CARTESIAN_POINT ( 'NONE',  ( -32.50000000000000000, 20.50000000000000000, -151.0552959529999839 ) ) ;
#19419=VERTEX_POINT ( 'NONE', #8113 ) ;
#19420=DIRECTION ( 'NONE',  ( -1.000000000000000000, 0.000000000000000000, 0.000000000000000000 ) ) ;
#19425=FACE_OUTER_BOUND ( 'NONE', #5529, .T. ) ;
#19429=FACE_OUTER_BOUND ( 'NONE', #8587, .T. ) ;
#19432=CARTESIAN_POINT ( 'NONE',  ( -31.00000000000000000, 19.50000000000000000, -149.5552959529999839 ) ) ;
#19434=ORIENTED_EDGE ( 'NONE', *, *, #8625, .F. ) ;
#19436=CIRCLE ( 'NONE', #22084, 2.000000000000000000 ) ;
#19437=VECTOR ( 'NONE', #12785, 1000.000000000000000 ) ;
#19440=EDGE_CURVE ( 'NONE', #13274, #4135, #16333, .T. ) ;
#19445=FILL_AREA_STYLE ('',( #17533 ) ) ;
#19451=ORIENTED_EDGE ( 'NONE', *, *, #529, .T. ) ;
#19455=VECTOR ( 'NONE', #7516, 1000.000000000000000 ) ;
#19457=AXIS2_PLACEMENT_3D ( 'NONE', #14990, #9378, #13430 ) ;
#19459=CARTESIAN_POINT ( 'NONE',  ( 19.00000000000000000, 33.50000000000000000, -150.0552959529999839 ) ) ;
#19463=EDGE_CURVE ( 'NONE', #1863, #22853, #22042, .T. ) ;
#19467=VERTEX_POINT ( 'NONE', #9284 ) ;
#19468=PLANE ( 'NONE',  #14401 ) ;
#19476=ORIENTED_EDGE ( 'NONE', *, *, #12699, .F. ) ;
#19480=VERTEX_POINT ( 'NONE', #13446 ) ;
#19481=DIRECTION ( 'NONE',  ( 1.000000000000000000, 0.000000000000000000, 0.000000000000000000 ) ) ;
#19482=CARTESIAN_POINT ( 'NONE',  ( -13.86630785140000022, -51.50000000000000000, -137.0552959530000123 ) ) ;
#19483=CARTESIAN_POINT ( 'NONE',  ( -3.500000000000000000, 42.50000000000000000, -150.0552959529999839 ) ) ;
#19487=LINE ( 'NONE', #13644, #18570 ) ;
#19489=AXIS2_PLACEMENT_3D ( 'NONE', #8218, #21445, #3125 ) ;
#19491=CARTESIAN_POINT ( 'NONE',  ( -16.50000000000000000, -43.00000000000000000, -145.5552959529999839 ) ) ;
#19497=CARTESIAN_POINT ( 'NONE',  ( 31.82297112080000190, 40.41789419139999495, -136.0552959530000123 ) ) ;
#19498=ORIENTED_EDGE ( 'NONE', *, *, #14572, .T. ) ;
#19505=EDGE_LOOP ( 'NONE', ( #23412, #13560, #21077, #21606 ) ) ;
#19510=EDGE_LOOP ( 'NONE', ( #1729, #10485, #13751, #13061 ) ) ;
#19523=ORIENTED_EDGE ( 'NONE', *, *, #10388, .T. ) ;
#19527=CARTESIAN_POINT ( 'NONE',  ( 32.50000000000000000, 39.80430157320000006, -149.5552959529999839 ) ) ;
#19533=CARTESIAN_POINT ( 'NONE',  ( -32.50000000000000000, -50.00000000000000000, -137.0552959530000123 ) ) ;
#19536=CARTESIAN_POINT ( 'NONE',  ( -31.75000000000000000, -51.50000000000000000, -149.5552959529999839 ) ) ;
#19539=AXIS2_PLACEMENT_3D ( 'NONE', #18904, #9966, #11874 ) ;
#19540=PLANE ( 'NONE',  #16828 ) ;
#19546=CARTESIAN_POINT ( 'NONE',  ( -32.50000000000000000, 50.00000000000000000, -149.5552959529999839 ) ) ;
#19552=CARTESIAN_POINT ( 'NONE',  ( 3.175121949262585286, 27.24084097722915132, -150.0552959529999839 ) ) ;
#19555=VECTOR ( 'NONE', #4316, 1000.000000000000000 ) ;
#19557=ORIENTED_EDGE ( 'NONE', *, *, #5568, .F. ) ;
#19559=ORIENTED_EDGE ( 'NONE', *, *, #12358, .T. ) ;
#19563=EDGE_CURVE ( 'NONE', #9566, #12161, #6199, .T. ) ;
#19567=EDGE_CURVE ( 'NONE', #14976, #2513, #13334, .T. ) ;
#19569=CARTESIAN_POINT ( 'NONE',  ( 1.133692148550000001, 51.50000000000000000, -136.5552959530000123 ) ) ;
#19589=VERTEX_POINT ( 'NONE', #22974 ) ;
#19590=EDGE_CURVE ( 'NONE', #21465, #20697, #2174, .T. ) ;
#19592=CARTESIAN_POINT ( 'NONE',  ( -7.101996734231647679, 19.50000000000000711, -150.0552959529999839 ) ) ;
#19597=DIRECTION ( 'NONE',  ( -1.000000000000000000, 0.000000000000000000, -2.245315044999999693E-12 ) ) ;
#19606=ORIENTED_EDGE ( 'NONE', *, *, #6146, .F. ) ;
#19612=EDGE_LOOP ( 'NONE', ( #19398, #8426 ) ) ;
#19615=ORIENTED_EDGE ( 'NONE', *, *, #16910, .T. ) ;
#19619=EDGE_CURVE ( 'NONE', #12394, #9978, #6546, .T. ) ;
#19625=ORIENTED_EDGE ( 'NONE', *, *, #3520, .F. ) ;
#19627=ORIENTED_EDGE ( 'NONE', *, *, #16238, .F. ) ;
#19628=PLANE ( 'NONE',  #14703 ) ;
#19640=ORIENTED_EDGE ( 'NONE', *, *, #6753, .T. ) ;
#19644=DIRECTION ( 'NONE',  ( -0.6459422414661291079, 0.7633862853691523176, -2.273736754430455399E-12 ) ) ;
#19651=CARTESIAN_POINT ( 'NONE',  ( 0.000000000000000000, 0.000000000000000000, -150.0552959529999839 ) ) ;
#19653=CARTESIAN_POINT ( 'NONE',  ( 5.700764968559962398, -2.580208454387413752, -150.0552959529999839 ) ) ;
#19669=CARTESIAN_POINT ( 'NONE',  ( 15.50000000000000000, 36.50000000000000000, -150.0552959529999839 ) ) ;
#19670=ORIENTED_EDGE ( 'NONE', *, *, #6340, .T. ) ;
#19673=EDGE_CURVE ( 'NONE', #9183, #3527, #17912, .T. ) ;
#19674=LINE ( 'NONE', #7406, #6614 ) ;
#19675=ORIENTED_EDGE ( 'NONE', *, *, #14903, .T. ) ;
#19682=CARTESIAN_POINT ( 'NONE',  ( 17.57628698940784773, 21.71923945896039854, -150.0552959529999839 ) ) ;
#19683=CARTESIAN_POINT ( 'NONE',  ( -18.00000000000000000, -43.00000000000000000, -150.0552959529999839 ) ) ;
#19691=CARTESIAN_POINT ( 'NONE',  ( 18.95053822279999878, -51.50000000000000000, -149.5552959529999839 ) ) ;
#19695=VECTOR ( 'NONE', #6072, 1000.000000000000000 ) ;
#19703=EDGE_CURVE ( 'NONE', #17877, #6526, #17373, .T. ) ;
#19704=LINE ( 'NONE', #10639, #1308 ) ;
#19710=ORIENTED_EDGE ( 'NONE', *, *, #2189, .F. ) ;
#19716=DIRECTION ( 'NONE',  ( 0.000000000000000000, 1.000000000000000000, -2.245315044999999693E-12 ) ) ;
#19720=VECTOR ( 'NONE', #5905, 1000.000000000000000 ) ;
#19728=ADVANCED_FACE ( 'NONE', ( #7134 ), #8, .T. ) ;
#19741=VECTOR ( 'NONE', #14371, 1000.000000000000000 ) ;
#19744=PLANE ( 'NONE',  #7223 ) ;
#19745=VECTOR ( 'NONE', #19644, 1000.000000000000227 ) ;
#19747=VECTOR ( 'NONE', #16750, 1000.000000000000000 ) ;
#19752=ORIENTED_EDGE ( 'NONE', *, *, #16126, .T. ) ;
#19756=EDGE_CURVE ( 'NONE', #11584, #7053, #3455, .T. ) ;
#19767=DIRECTION ( 'NONE',  ( 0.000000000000000000, 0.000000000000000000, 1.000000000000000000 ) ) ;
#19768=ORIENTED_EDGE ( 'NONE', *, *, #19619, .T. ) ;
#19770=B_SPLINE_CURVE_WITH_KNOTS ( 'NONE', 3,
 ( #5484, #5367, #1579, #1933, #5594, #18097, #21912, #12728, #250, #12843, #10702, #21556, #5238, #23, #19772, #1807, #7382, #5711 ),
 .UNSPECIFIED., .F., .F.,
 ( 4, 2, 2, 2, 2, 2, 2, 2, 4 ),
 ( 0.000000000000000000, 0.1250000000000000000, 0.2500000000000000000, 0.3750000000000000000, 0.5000000000000000000, 0.6250000000000000000, 0.7500000000000000000, 0.8750000000000000000, 1.000000000000000000 ),
 .UNSPECIFIED. ) ;
#19772=CARTESIAN_POINT ( 'NONE',  ( 7.121359165062779439, -5.010856941112688645, -150.0552959529999839 ) ) ;
#19775=ORIENTED_EDGE ( 'NONE', *, *, #22788, .F. ) ;
#19776=FACE_OUTER_BOUND ( 'NONE', #22721, .T. ) ;
#19777=CARTESIAN_POINT ( 'NONE',  ( 19.77963439019999825, 51.26338628519999929, -143.0552959529999839 ) ) ;
#19784=CARTESIAN_POINT ( 'NONE',  ( 4.750000000000000000, -38.23606797749999942, -150.5552959529999839 ) ) ;
#19797=VECTOR ( 'NONE', #8595, 1000.000000000000000 ) ;
#19809=CARTESIAN_POINT ( 'NONE',  ( -15.39054929727204879, -44.46182274717511973, -150.0552959529999839 ) ) ;
#19812=AXIS2_PLACEMENT_3D ( 'NONE', #10603, #16338, #1719 ) ;
#19817=EDGE_CURVE ( 'NONE', #17914, #384, #18535, .T. ) ;
#19820=ORIENTED_EDGE ( 'NONE', *, *, #21534, .T. ) ;
#19825=ORIENTED_EDGE ( 'NONE', *, *, #5030, .F. ) ;
#19826=AXIS2_PLACEMENT_3D ( 'NONE', #1446, #8908, #23328 ) ;
#19834=VERTEX_POINT ( 'NONE', #5813 ) ;
#19845=AXIS2_PLACEMENT_3D ( 'NONE', #13824, #981, #21206 ) ;
#19863=DIRECTION ( 'NONE',  ( -1.000000000000000000, 0.000000000000000000, 2.245315044999999693E-12 ) ) ;
#19865=DIRECTION ( 'NONE',  ( 1.000000000000000000, 0.000000000000000000, 0.000000000000000000 ) ) ;
#19868=LINE ( 'NONE', #17962, #4523 ) ;
#19872=CARTESIAN_POINT ( 'NONE',  ( -4.500000000000000000, 40.00000000000000000, -151.0552959529999839 ) ) ;
#19876=VERTEX_POINT ( 'NONE', #14632 ) ;
#19879=CARTESIAN_POINT ( 'NONE',  ( 18.95053822279999878, 51.00000000000000000, -149.5552959529999839 ) ) ;
#19882=FACE_OUTER_BOUND ( 'NONE', #15206, .T. ) ;
#19883=CARTESIAN_POINT ( 'NONE',  ( 31.96891336220000213, -40.94938100119999547, -149.8052959529999839 ) ) ;
#19891=VERTEX_POINT ( 'NONE', #5583 ) ;
#19896=ORIENTED_EDGE ( 'NONE', *, *, #11989, .F. ) ;
#19899=CARTESIAN_POINT ( 'NONE',  ( 6.500000000000000000, 20.50000000000000000, -151.0552959529999839 ) ) ;
#19902=FACE_BOUND ( 'NONE', #13381, .T. ) ;
#19904=ORIENTED_EDGE ( 'NONE', *, *, #11859, .F. ) ;
#19912=ORIENTED_EDGE ( 'NONE', *, *, #984, .T. ) ;
#19913=FACE_OUTER_BOUND ( 'NONE', #585, .T. ) ;
#19916=ORIENTED_EDGE ( 'NONE', *, *, #18857, .F. ) ;
#19919=CARTESIAN_POINT ( 'NONE',  ( 19.00000000000000000, 39.50000000000000000, -151.0552959529999839 ) ) ;
#19926=VECTOR ( 'NONE', #12758, 1000.000000000000000 ) ;
#19928=FACE_OUTER_BOUND ( 'NONE', #1764, .T. ) ;
#19930=DIRECTION ( 'NONE',  ( -1.000000000000000000, 0.000000000000000000, 2.257144641399999941E-12 ) ) ;
#19931=ORIENTED_EDGE ( 'NONE', *, *, #6628, .F. ) ;
#19934=B_SPLINE_CURVE_WITH_KNOTS ( 'NONE', 3,
 ( #22969, #2751, #12121, #964, #15356, #19271, #13441, #9979, #2981, #13917, #17013, #728, #7963, #20708, #4402, #11643, #18919, #9861 ),
 .UNSPECIFIED., .F., .F.,
 ( 4, 2, 2, 2, 2, 2, 2, 2, 4 ),
 ( 0.000000000000000000, 0.1250000000000000000, 0.2500000000000000000, 0.3750000000000000000, 0.5000000000000000000, 0.6250000000000000000, 0.7500000000000000000, 0.8750000000000000000, 1.000000000000000000 ),
 .UNSPECIFIED. ) ;
#19946=DIRECTION ( 'NONE',  ( 0.000000000000000000, 1.000000000000000000, 2.273736754430000208E-12 ) ) ;
#19949=ORIENTED_EDGE ( 'NONE', *, *, #21562, .F. ) ;
#19951=DIRECTION ( 'NONE',  ( 2.256683728769999802E-12, 0.000000000000000000, 1.000000000000000000 ) ) ;
#19952=DIRECTION ( 'NONE',  ( 0.000000000000000000, -1.000000000000000000, 0.000000000000000000 ) ) ;
#19954=CARTESIAN_POINT ( 'NONE',  ( 19.13369214859999801, -50.50000000000000000, -150.0552959529999839 ) ) ;
#19958=DIRECTION ( 'NONE',  ( -2.257252162960000001E-12, 0.000000000000000000, -1.000000000000000000 ) ) ;
#19973=CARTESIAN_POINT ( 'NONE',  ( 19.13369214859999801, -51.50000000000000000, -150.0552959529999839 ) ) ;
#19975=ORIENTED_EDGE ( 'NONE', *, *, #3959, .T. ) ;
#19978=AXIS2_PLACEMENT_3D ( 'NONE', #20892, #4582, #19098 ) ;
#19981=ORIENTED_EDGE ( 'NONE', *, *, #18978, .F. ) ;
#19992=PLANE ( 'NONE',  #18233 ) ;
#20001=DIRECTION ( 'NONE',  ( -1.000000000000000000, 0.000000000000000000, 0.000000000000000000 ) ) ;
#20008=VERTEX_POINT ( 'NONE', #17462 ) ;
#20028=DIRECTION ( 'NONE',  ( 0.6459422414661291079, 0.7633862853691523176, 2.273736754430455399E-12 ) ) ;
#20031=CYLINDRICAL_SURFACE ( 'NONE', #848, 1.499999999999996225 ) ;
#20034=ORIENTED_EDGE ( 'NONE', *, *, #5158, .F. ) ;
#20037=ORIENTED_EDGE ( 'NONE', *, *, #8128, .F. ) ;
#20039=PLANE ( 'NONE',  #5676 ) ;
#20046=SHAPE_DEFINITION_REPRESENTATION ( #1199, #15114 ) ;
#20049=FACE_OUTER_BOUND ( 'NONE', #14184, .T. ) ;
#20050=ORIENTED_EDGE ( 'NONE', *, *, #20568, .F. ) ;
#20052=ORIENTED_EDGE ( 'NONE', *, *, #15186, .T. ) ;
#20060=DIRECTION ( 'NONE',  ( 0.000000000000000000, 1.000000000000000000, 0.000000000000000000 ) ) ;
#20062=VECTOR ( 'NONE', #8200, 1000.000000000000000 ) ;
#20063=CARTESIAN_POINT ( 'NONE',  ( 13.13369214859999978, -51.50000000000000000, -137.0552959530000123 ) ) ;
#20064=ORIENTED_EDGE ( 'NONE', *, *, #554, .F. ) ;
#20066=ORIENTED_EDGE ( 'NONE', *, *, #22649, .T. ) ;
#20081=ORIENTED_EDGE ( 'NONE', *, *, #14777, .T. ) ;
#20087=LINE ( 'NONE', #7354, #4551 ) ;
#20091=CARTESIAN_POINT ( 'NONE',  ( -32.00000000000000000, -50.00000000000000000, -149.5552959529999839 ) ) ;
#20092=EDGE_CURVE ( 'NONE', #10473, #18841, #16274, .T. ) ;
#20097=CARTESIAN_POINT ( 'NONE',  ( 32.14594224149999491, 40.79958733410000349, -142.8052959529999839 ) ) ;
#20099=VECTOR ( 'NONE', #3562, 1000.000000000000000 ) ;
#20100=ORIENTED_EDGE ( 'NONE', *, *, #20435, .F. ) ;
#20101=CARTESIAN_POINT ( 'NONE',  ( 3.580113616945115318, -4.700859805997813723, -150.0552959529999839 ) ) ;
#20105=CARTESIAN_POINT ( 'NONE',  ( -3.500000000000000000, 46.50000000000000000, -150.5552959529999839 ) ) ;
#20126=PLANE ( 'NONE',  #8673 ) ;
#20132=VECTOR ( 'NONE', #15821, 1000.000000000000000 ) ;
#20133=ORIENTED_EDGE ( 'NONE', *, *, #13531, .F. ) ;
#20136=AXIS2_PLACEMENT_3D ( 'NONE', #20553, #19226, #1287 ) ;
#20139=VECTOR ( 'NONE', #8841, 1000.000000000000000 ) ;
#20140=VECTOR ( 'NONE', #13910, 1000.000000000000000 ) ;
#20141=DIRECTION ( 'NONE',  ( 0.000000000000000000, 1.000000000000000000, 0.000000000000000000 ) ) ;
#20149=DIRECTION ( 'NONE',  ( -0.7071067811865474617, 0.7071067811865476838, 0.000000000000000000 ) ) ;
#20151=ADVANCED_FACE ( 'NONE', ( #8635 ), #15910, .T. ) ;
#20152=DIRECTION ( 'NONE',  ( 0.6459422414661299960, 0.7633862853691516515, 2.257453483404490485E-12 ) ) ;
#20161=CARTESIAN_POINT ( 'NONE',  ( 19.13369214859999801, 51.00000000000000000, -149.5552959529999839 ) ) ;
#20163=PLANE ( 'NONE',  #13655 ) ;
#20164=EDGE_CURVE ( 'NONE', #20657, #16830, #16437, .T. ) ;
#20168=EDGE_CURVE ( 'NONE', #21310, #18719, #14837, .T. ) ;
#20170=EDGE_CURVE ( 'NONE', #14107, #10473, #13268, .T. ) ;
#20172=CARTESIAN_POINT ( 'NONE',  ( -32.50000000000000000, -36.00000000000000000, -151.0552959529999839 ) ) ;
#20174=CYLINDRICAL_SURFACE ( 'NONE', #1733, 0.5000000000000079936 ) ;
#20182=ORIENTED_EDGE ( 'NONE', *, *, #12431, .F. ) ;
#20189=CARTESIAN_POINT ( 'NONE',  ( 4.500000000000000000, -3.500000000000000000, -145.5552959529999839 ) ) ;
#20197=CARTESIAN_POINT ( 'NONE',  ( 1.500000000000000000, -3.500000000000000000, -150.0552959529999839 ) ) ;
#20198=EDGE_LOOP ( 'NONE', ( #6602, #7947, #489, #21753 ) ) ;
#20199=DIRECTION ( 'NONE',  ( 0.000000000000000000, 0.000000000000000000, 1.000000000000000000 ) ) ;
#20202=VECTOR ( 'NONE', #15088, 1000.000000000000000 ) ;
#20204=ORIENTED_EDGE ( 'NONE', *, *, #13438, .F. ) ;
#20205=DIRECTION ( 'NONE',  ( 0.000000000000000000, 0.000000000000000000, 1.000000000000000000 ) ) ;
#20212=ORIENTED_EDGE ( 'NONE', *, *, #3210, .F. ) ;
#20213=LINE ( 'NONE', #14959, #18230 ) ;
#20215=CARTESIAN_POINT ( 'NONE',  ( -23.18315392570000100, 51.50000000000000000, -137.0552959530000123 ) ) ;
#20219=DIRECTION ( 'NONE',  ( 0.000000000000000000, 1.000000000000000000, 0.000000000000000000 ) ) ;
#20221=DIRECTION ( 'NONE',  ( 1.000000000000000000, 0.000000000000000000, 0.000000000000000000 ) ) ;
#20223=AXIS2_PLACEMENT_3D ( 'NONE', #15259, #15607, #7979 ) ;
#20237=DIRECTION ( 'NONE',  ( 0.000000000000000000, -1.000000000000000000, 0.000000000000000000 ) ) ;
#20240=VECTOR ( 'NONE', #11543, 1000.000000000000000 ) ;
#20243=CARTESIAN_POINT ( 'NONE',  ( -31.00000000000000000, -36.00000000000000000, -151.0552959529999839 ) ) ;
#20245=CARTESIAN_POINT ( 'NONE',  ( -12.50000000000000000, 25.50000000000000000, -151.0552959529999839 ) ) ;
#20247=ORIENTED_EDGE ( 'NONE', *, *, #22379, .T. ) ;
#20248=EDGE_CURVE ( 'NONE', #6873, #20386, #18296, .T. ) ;
#20250=CARTESIAN_POINT ( 'NONE',  ( 3.000000000000000000, -3.500000000000000000, -150.0552959529999839 ) ) ;
#20258=DIRECTION ( 'NONE',  ( 5.968558980390000333E-14, -1.000000000000000000, 0.000000000000000000 ) ) ;
#20259=LINE ( 'NONE', #11183, #13661 ) ;
#20260=ORIENTED_EDGE ( 'NONE', *, *, #18652, .F. ) ;
#20267=CARTESIAN_POINT ( 'NONE',  ( 7.500000000000000000, -3.500000000000000000, -150.0552959529999839 ) ) ;
#20273=EDGE_CURVE ( 'NONE', #7104, #3870, #18403, .T. ) ;
#20280=LINE ( 'NONE', #7649, #16206 ) ;
#20282=DIRECTION ( 'NONE',  ( 0.000000000000000000, 0.000000000000000000, 1.000000000000000000 ) ) ;
#20283=DIRECTION ( 'NONE',  ( 0.000000000000000000, -1.000000000000000000, 2.257144641399999941E-12 ) ) ;
#20284=DIRECTION ( 'NONE',  ( 0.000000000000000000, 0.000000000000000000, -1.000000000000000000 ) ) ;
#20294=DIRECTION ( 'NONE',  ( 0.7633862853691524286, 0.6459422414661293299, 0.000000000000000000 ) ) ;
#20295=DIRECTION ( 'NONE',  ( 0.000000000000000000, 1.000000000000000000, 0.000000000000000000 ) ) ;
#20297=EDGE_CURVE ( 'NONE', #9607, #2844, #13866, .T. ) ;
#20300=EDGE_CURVE ( 'NONE', #15915, #16877, #15658, .T. ) ;
#20301=CARTESIAN_POINT ( 'NONE',  ( -32.50000000000000000, 47.50000000000000000, -150.5552959529999839 ) ) ;
#20310=DIRECTION ( 'NONE',  ( -1.000000000000000000, 0.000000000000000000, 0.000000000000000000 ) ) ;
#20312=CARTESIAN_POINT ( 'NONE',  ( 19.84954298759999958, 51.20423285660000090, -150.0552959529999839 ) ) ;
#20322=ORIENTED_EDGE ( 'NONE', *, *, #7416, .F. ) ;
#20328=CARTESIAN_POINT ( 'NONE',  ( -6.683153925719999222, -51.50000000000000000, -136.0552959530000123 ) ) ;
#20332=VERTEX_POINT ( 'NONE', #9687 ) ;
#20333=CARTESIAN_POINT ( 'NONE',  ( -31.50000000000000000, 14.00000000000000000, -144.0552959529999839 ) ) ;
#20337=CARTESIAN_POINT ( 'NONE',  ( -31.00000000000000000, -36.00000000000000000, -150.5552959529999839 ) ) ;
#20348=EDGE_CURVE ( 'NONE', #18382, #10837, #2977, .T. ) ;
#20372=DIRECTION ( 'NONE',  ( 0.7633862853691524286, 0.6459422414661293299, -5.745404152441152829E-15 ) ) ;
#20381=ORIENTED_EDGE ( 'NONE', *, *, #2912, .T. ) ;
#20384=AXIS2_PLACEMENT_3D ( 'NONE', #15995, #17664, #10151 ) ;
#20386=VERTEX_POINT ( 'NONE', #2697 ) ;
#20387=DIRECTION ( 'NONE',  ( 0.000000000000000000, -1.000000000000000000, -2.245315044999999693E-12 ) ) ;
#20393=CARTESIAN_POINT ( 'NONE',  ( 13.66051412332252646, 38.90191174487609516, -150.0552959529999839 ) ) ;
#20398=ORIENTED_EDGE ( 'NONE', *, *, #8041, .F. ) ;
#20413=AXIS2_PLACEMENT_3D ( 'NONE', #3020, #10366, #21220 ) ;
#20415=ADVANCED_FACE ( 'NONE', ( #20902 ), #11949, .F. ) ;
#20417=DIRECTION ( 'NONE',  ( 2.255973186040000320E-12, 0.000000000000000000, 1.000000000000000000 ) ) ;
#20422=AXIS2_PLACEMENT_3D ( 'NONE', #9740, #6196, #13331 ) ;
#20425=ORIENTED_EDGE ( 'NONE', *, *, #9522, .T. ) ;
#20428=VERTEX_POINT ( 'NONE', #2069 ) ;
#20430=ORIENTED_EDGE ( 'NONE', *, *, #10093, .T. ) ;
#20435=EDGE_CURVE ( 'NONE', #19192, #19834, #8607, .T. ) ;
#20436=LINE ( 'NONE', #4477, #18610 ) ;
#20437=CARTESIAN_POINT ( 'NONE',  ( -6.774730888589999722, 51.50000000000000000, -149.5552959529999839 ) ) ;
#20440=CARTESIAN_POINT ( 'NONE',  ( 1.133692148550000001, 50.99999999970000175, -136.0552959530000123 ) ) ;
#20442=ORIENTED_EDGE ( 'NONE', *, *, #10432, .F. ) ;
#20444=AXIS2_PLACEMENT_3D ( 'NONE', #9746, #2524, #11771 ) ;
#20445=ADVANCED_FACE ( 'NONE', ( #1955 ), #10507, .F. ) ;
#20462=CARTESIAN_POINT ( 'NONE',  ( -3.765581077048879788, 46.49999999999999289, -150.0552959529999839 ) ) ;
#20467=LINE ( 'NONE', #5823, #13302 ) ;
#20469=CARTESIAN_POINT ( 'NONE',  ( 31.50000000000000000, 0.000000000000000000, -136.0552959530000123 ) ) ;
#20473=ORIENTED_EDGE ( 'NONE', *, *, #20704, .T. ) ;
#20476=EDGE_LOOP ( 'NONE', ( #16161, #13708, #8027, #21846 ) ) ;
#20479=FACE_OUTER_BOUND ( 'NONE', #18901, .T. ) ;
#20484=CARTESIAN_POINT ( 'NONE',  ( 31.00000000000000000, 39.80430157320000006, -149.5552959529999839 ) ) ;
#20502=VECTOR ( 'NONE', #10590, 1000.000000000000000 ) ;
#20505=VECTOR ( 'NONE', #12550, 1000.000000000000000 ) ;
#20506=ADVANCED_FACE ( 'NONE', ( #6719 ), #19468, .F. ) ;
#20517=ORIENTED_EDGE ( 'NONE', *, *, #6361, .F. ) ;
#20520=DIRECTION ( 'NONE',  ( 0.000000000000000000, 0.000000000000000000, 1.000000000000000000 ) ) ;
#20525=CARTESIAN_POINT ( 'NONE',  ( 31.00000000000000000, 39.80430157320000006, -151.0552959529999839 ) ) ;
#20530=VERTEX_POINT ( 'NONE', #18358 ) ;
#20534=EDGE_CURVE ( 'NONE', #20624, #7366, #16801, .T. ) ;
#20538=CYLINDRICAL_SURFACE ( 'NONE', #14329, 0.5000000000000079936 ) ;
#20540=CARTESIAN_POINT ( 'NONE',  ( 19.84954298779999959, -51.20423285649999912, -149.5552959529999839 ) ) ;
#20542=CARTESIAN_POINT ( 'NONE',  ( 7.014880255698754397, -48.99993274156953049, -150.0552959529999839 ) ) ;
#20547=ORIENTED_EDGE ( 'NONE', *, *, #20297, .T. ) ;
#20548=LINE ( 'NONE', #11483, #9105 ) ;
#20552=ORIENTED_EDGE ( 'NONE', *, *, #10246, .F. ) ;
#20553=CARTESIAN_POINT ( 'NONE',  ( -10.00000000000000000, 42.50000000000000000, -150.0552959529999839 ) ) ;
#20556=DIRECTION ( 'NONE',  ( 0.000000000000000000, 0.000000000000000000, 1.000000000000000000 ) ) ;
#20559=ORIENTED_EDGE ( 'NONE', *, *, #16787, .T. ) ;
#20560=CARTESIAN_POINT ( 'NONE',  ( -1.898424454315990273, 45.72687021304480481, -150.0552959530000123 ) ) ;
#20568=EDGE_CURVE ( 'NONE', #13256, #2055, #17379, .T. ) ;
#20573=CARTESIAN_POINT ( 'NONE',  ( -31.00000000000000000, 19.50000000000000000, -150.0552959529999839 ) ) ;
#20574=ORIENTED_EDGE ( 'NONE', *, *, #1371, .F. ) ;
#20578=CARTESIAN_POINT ( 'NONE',  ( -4.726870213046807656, 46.10157554568340288, -150.0552959529999839 ) ) ;
#20588=VECTOR ( 'NONE', #21082, 1000.000000000000000 ) ;
#20597=ORIENTED_EDGE ( 'NONE', *, *, #9302, .F. ) ;
#20607=CARTESIAN_POINT ( 'NONE',  ( -13.86630785140000022, -51.50000000000000000, -137.0552959530000123 ) ) ;
#20608=EDGE_CURVE ( 'NONE', #2844, #13263, #13565, .T. ) ;
#20610=B_SPLINE_CURVE_WITH_KNOTS ( 'NONE', 1,
 ( #7203, #7321 ),
 .UNSPECIFIED., .F., .F.,
 ( 2, 2 ),
 ( -0.5146970993560000540, 15.26952906260000020 ),
 .UNSPECIFIED. ) ;
#20619=DIRECTION ( 'NONE',  ( 0.000000000000000000, 2.259525899719999991E-12, 1.000000000000000000 ) ) ;
#20623=FACE_BOUND ( 'NONE', #3252, .T. ) ;
#20624=VERTEX_POINT ( 'NONE', #12135 ) ;
#20639=CARTESIAN_POINT ( 'NONE',  ( 8.750000000000000000, 0.000000000000000000, -150.0552959529999839 ) ) ;
#20644=DIRECTION ( 'NONE',  ( 0.7633862853691524286, -0.6459422414661293299, 2.886579864030576411E-15 ) ) ;
#20646=EDGE_LOOP ( 'NONE', ( #20655, #557, #20064, #17279 ) ) ;
#20648=CARTESIAN_POINT ( 'NONE',  ( -32.50000000000000000, 47.50000000000000000, -150.0552959529999839 ) ) ;
#20655=ORIENTED_EDGE ( 'NONE', *, *, #3938, .T. ) ;
#20657=VERTEX_POINT ( 'NONE', #4771 ) ;
#20661=ORIENTED_EDGE ( 'NONE', *, *, #19317, .T. ) ;
#20664=EDGE_LOOP ( 'NONE', ( #1541, #21155 ) ) ;
#20670=LINE ( 'NONE', #570, #20897 ) ;
#20674=CARTESIAN_POINT ( 'NONE',  ( 32.50000000000000000, 36.50000000010000178, -136.0552959530000123 ) ) ;
#20682=DIRECTION ( 'NONE',  ( 0.000000000000000000, 0.000000000000000000, -1.000000000000000000 ) ) ;
#20683=ORIENTED_EDGE ( 'NONE', *, *, #17277, .T. ) ;
#20688=CARTESIAN_POINT ( 'NONE',  ( 20.50000000000000000, -20.50000000000000000, -150.0552959529999839 ) ) ;
#20696=CARTESIAN_POINT ( 'NONE',  ( 8.750000000000000000, -47.00000000000000000, -151.0552959529999839 ) ) ;
#20697=VERTEX_POINT ( 'NONE', #6314 ) ;
#20703=LINE ( 'NONE', #15351, #16676 ) ;
#20704=EDGE_CURVE ( 'NONE', #2624, #6475, #20966, .T. ) ;
#20708=CARTESIAN_POINT ( 'NONE',  ( 2.100999472805455959, -1.656359840075259937, -150.0552959529999839 ) ) ;
#20715=LINE ( 'NONE', #17143, #7041 ) ;
#20717=CARTESIAN_POINT ( 'NONE',  ( -13.79923503141243302, -42.08020845437312829, -150.0552959529999839 ) ) ;
#20718=DIRECTION ( 'NONE',  ( -1.000000000000000000, 0.000000000000000000, 0.000000000000000000 ) ) ;
#20721=DIRECTION ( 'NONE',  ( 1.000000000000000000, 0.000000000000000000, 0.000000000000000000 ) ) ;
#20725=CARTESIAN_POINT ( 'NONE',  ( 18.95053822279999878, -51.00000000000000000, -149.5552959529999839 ) ) ;
#20729=CARTESIAN_POINT ( 'NONE',  ( 31.50000000000000000, 40.03620104880000241, -136.0552959530000123 ) ) ;
#20730=EDGE_CURVE ( 'NONE', #9450, #8748, #12837, .T. ) ;
#20736=AXIS2_PLACEMENT_3D ( 'NONE', #6310, #507, #2638 ) ;
#20748=ADVANCED_FACE ( 'NONE', ( #21678 ), #3693, .T. ) ;
#20755=ORIENTED_EDGE ( 'NONE', *, *, #2855, .F. ) ;
#20761=ORIENTED_EDGE ( 'NONE', *, *, #2669, .T. ) ;
#20763=CARTESIAN_POINT ( 'NONE',  ( -25.86630785139999844, -51.50000000000000000, -137.0552959530000123 ) ) ;
#20764=ORIENTED_EDGE ( 'NONE', *, *, #10136, .T. ) ;
#20771=LINE ( 'NONE', #22667, #13938 ) ;
#20777=( LENGTH_UNIT ( ) NAMED_UNIT ( * ) SI_UNIT ( .MILLI., .METRE. ) );
#20782=ORIENTED_EDGE ( 'NONE', *, *, #7034, .F. ) ;
#20783=VECTOR ( 'NONE', #11471, 1000.000000000000000 ) ;
#20786=CARTESIAN_POINT ( 'NONE',  ( 13.13369214859999978, 50.50000000000000000, -137.0552959530000123 ) ) ;
#20792=ORIENTED_EDGE ( 'NONE', *, *, #5158, .T. ) ;
#20793=CARTESIAN_POINT ( 'NONE',  ( 13.13369214859999978, -51.00000000000000000, -137.0552959530000123 ) ) ;
#20796=CARTESIAN_POINT ( 'NONE',  ( 24.01497134762854913, 33.88109793996614627, -150.0552959529999839 ) ) ;
#20823=FACE_OUTER_BOUND ( 'NONE', #5974, .T. ) ;
#20825=EDGE_CURVE ( 'NONE', #3203, #4135, #14770, .T. ) ;
#20827=ORIENTED_EDGE ( 'NONE', *, *, #11999, .T. ) ;
#20829=CARTESIAN_POINT ( 'NONE',  ( -31.50000000000000000, 14.00000000000000000, -144.0552959529999839 ) ) ;
#20836=LINE ( 'NONE', #4532, #4488 ) ;
#20844=DIRECTION ( 'NONE',  ( 0.000000000000000000, -1.000000000000000000, 0.000000000000000000 ) ) ;
#20847=ORIENTED_EDGE ( 'NONE', *, *, #15642, .F. ) ;
#20852=VERTEX_POINT ( 'NONE', #3579 ) ;
#20865=DIRECTION ( 'NONE',  ( 2.257242012349999735E-12, 0.000000000000000000, -1.000000000000000000 ) ) ;
#20869=EDGE_CURVE ( 'NONE', #17719, #18084, #21551, .T. ) ;
#20872=VECTOR ( 'NONE', #13805, 1000.000000000000000 ) ;
#20876=LINE ( 'NONE', #6235, #17564 ) ;
#20878=VECTOR ( 'NONE', #6669, 1000.000000000000000 ) ;
#20879=ADVANCED_FACE ( 'NONE', ( #7263 ), #1688, .F. ) ;
#20884=ADVANCED_FACE ( 'NONE', ( #11509 ), #481, .T. ) ;
#20887=EDGE_CURVE ( 'NONE', #11360, #19834, #11396, .T. ) ;
#20891=AXIS2_PLACEMENT_3D ( 'NONE', #1591, #15969, #19302 ) ;
#20892=CARTESIAN_POINT ( 'NONE',  ( 20.50000000000000000, 22.50000000000000000, -150.0552959529999839 ) ) ;
#20896=CARTESIAN_POINT ( 'NONE',  ( 4.698575659218127143, -5.000067229902920296, -150.0552959529999839 ) ) ;
#20897=VECTOR ( 'NONE', #687, 1000.000000000000000 ) ;
#20900=VECTOR ( 'NONE', #11621, 1000.000000000000227 ) ;
#20901=ORIENTED_EDGE ( 'NONE', *, *, #9804, .T. ) ;
#20902=FACE_OUTER_BOUND ( 'NONE', #5088, .T. ) ;
#20904=( NAMED_UNIT ( * ) SI_UNIT ( $, .STERADIAN. ) SOLID_ANGLE_UNIT ( ) );
#20906=DIRECTION ( 'NONE',  ( 0.000000000000000000, 1.000000000000000000, 2.245315043809999812E-12 ) ) ;
#20907=EDGE_LOOP ( 'NONE', ( #16337, #14380, #3756, #19559 ) ) ;
#20911=CARTESIAN_POINT ( 'NONE',  ( -32.50000000000000000, 1.000000000000000000, -149.5552959529999839 ) ) ;
#20919=AXIS2_PLACEMENT_3D ( 'NONE', #8884, #10901, #7349 ) ;
#20920=LINE ( 'NONE', #4608, #3392 ) ;
#20925=ORIENTED_EDGE ( 'NONE', *, *, #15327, .T. ) ;
#20926=DIRECTION ( 'NONE',  ( -1.000000000000000000, 0.000000000000000000, 0.000000000000000000 ) ) ;
#20927=DIRECTION ( 'NONE',  ( 1.000000000000000000, 0.000000000000000000, 0.000000000000000000 ) ) ;
#20930=VECTOR ( 'NONE', #488, 1000.000000000000000 ) ;
#20932=VERTEX_POINT ( 'NONE', #15227 ) ;
#20934=DIRECTION ( 'NONE',  ( 0.000000000000000000, 0.000000000000000000, 1.000000000000000000 ) ) ;
#20941=ADVANCED_FACE ( 'NONE', ( #6172 ), #18438, .F. ) ;
#20942=ORIENTED_EDGE ( 'NONE', *, *, #15058, .F. ) ;
#20945=EDGE_CURVE ( 'NONE', #15811, #6002, #11556, .T. ) ;
#20946=ORIENTED_EDGE ( 'NONE', *, *, #15760, .T. ) ;
#20947=PLANE ( 'NONE',  #4946 ) ;
#20953=( GEOMETRIC_REPRESENTATION_CONTEXT ( 3 ) GLOBAL_UNCERTAINTY_ASSIGNED_CONTEXT ( ( #10868 ) ) GLOBAL_UNIT_ASSIGNED_CONTEXT ( ( #13599, #3250, #2790 ) ) REPRESENTATION_CONTEXT ( 'NONE', 'WORKASPACE' ) );
#20963=CARTESIAN_POINT ( 'NONE',  ( 23.89269908169871925, -17.50000000000000000, -150.0552959529999839 ) ) ;
#20966=LINE ( 'NONE', #4658, #22751 ) ;
#20967=VECTOR ( 'NONE', #3112, 1000.000000000000000 ) ;
#20968=ORIENTED_EDGE ( 'NONE', *, *, #17106, .T. ) ;
#20981=EDGE_LOOP ( 'NONE', ( #8648, #14836, #17796, #8138 ) ) ;
#20984=CARTESIAN_POINT ( 'NONE',  ( 32.50000000000000000, -33.03620104880000241, -131.8162870490000103 ) ) ;
#20986=CIRCLE ( 'NONE', #464, 2.999999999999999112 ) ;
#20989=CARTESIAN_POINT ( 'NONE',  ( -0.9520167400862425966, 19.51924065639807537, -150.0552959530000123 ) ) ;
#20994=ORIENTED_EDGE ( 'NONE', *, *, #18735, .F. ) ;
#21004=ORIENTED_EDGE ( 'NONE', *, *, #21566, .F. ) ;
#21008=CARTESIAN_POINT ( 'NONE',  ( -16.84364015992474606, -40.60099947280546218, -150.0552959529999839 ) ) ;
#21015=ADVANCED_FACE ( 'NONE', ( #18548 ), #2152, .T. ) ;
#21016=EDGE_CURVE ( 'NONE', #23105, #18841, #358, .T. ) ;
#21021=ORIENTED_EDGE ( 'NONE', *, *, #3959, .F. ) ;
#21023=EDGE_CURVE ( 'NONE', #17988, #22710, #16667, .T. ) ;
#21024=VERTEX_POINT ( 'NONE', #14015 ) ;
#21035=ORIENTED_EDGE ( 'NONE', *, *, #11810, .T. ) ;
#21042=EDGE_CURVE ( 'NONE', #567, #5050, #837, .T. ) ;
#21046=ORIENTED_EDGE ( 'NONE', *, *, #10954, .T. ) ;
#21048=DIRECTION ( 'NONE',  ( 0.000000000000000000, -8.980547998385300260E-15, -1.000000000000000000 ) ) ;
#21056=ORIENTED_EDGE ( 'NONE', *, *, #19287, .T. ) ;
#21059=ORIENTED_EDGE ( 'NONE', *, *, #13454, .F. ) ;
#21069=VECTOR ( 'NONE', #11309, 1000.000000000000000 ) ;
#21077=ORIENTED_EDGE ( 'NONE', *, *, #4158, .F. ) ;
#21081=CARTESIAN_POINT ( 'NONE',  ( 31.64594224149999846, 40.56768785850000825, -149.5552959529999839 ) ) ;
#21082=DIRECTION ( 'NONE',  ( -1.000000000000000000, 0.000000000000000000, 0.000000000000000000 ) ) ;
#21084=VERTEX_POINT ( 'NONE', #3550 ) ;
#21089=DIRECTION ( 'NONE',  ( 1.000000000000000000, 0.000000000000000000, 0.000000000000000000 ) ) ;
#21092=DIRECTION ( 'NONE',  ( 1.000000000000000000, 0.000000000000000000, 0.000000000000000000 ) ) ;
#21093=CARTESIAN_POINT ( 'NONE',  ( 3.580208454387329375, -2.299235031440459931, -150.0552959529999839 ) ) ;
#21094=EDGE_LOOP ( 'NONE', ( #6721, #21177, #3476, #1236 ) ) ;
#21097=CARTESIAN_POINT ( 'NONE',  ( 31.00000000000000000, 39.80430157320000006, -150.5552959529999839 ) ) ;
#21098=EDGE_LOOP ( 'NONE', ( #17251, #17650, #20946, #8244 ) ) ;
#21099=EDGE_CURVE ( 'NONE', #18640, #21821, #7111, .T. ) ;
#21108=CARTESIAN_POINT ( 'NONE',  ( -32.50000000000000000, 10.25000000000000000, -149.5552959529999839 ) ) ;
#21109=CARTESIAN_POINT ( 'NONE',  ( 9.295843182377716118, -34.38416640352239284, -150.0552959530000123 ) ) ;
#21110=ORIENTED_EDGE ( 'NONE', *, *, #229, .T. ) ;
#21113=VERTEX_POINT ( 'NONE', #9338 ) ;
#21118=CARTESIAN_POINT ( 'NONE',  ( 31.96891336220000213, -40.94938100119999547, -149.8052959529999839 ) ) ;
#21123=ORIENTED_EDGE ( 'NONE', *, *, #22496, .T. ) ;
#21131=EDGE_CURVE ( 'NONE', #903, #13274, #5671, .T. ) ;
#21139=ORIENTED_EDGE ( 'NONE', *, *, #9532, .F. ) ;
#21145=DIRECTION ( 'NONE',  ( 0.000000000000000000, 1.000000000000000000, 0.000000000000000000 ) ) ;
#21148=CARTESIAN_POINT ( 'NONE',  ( -15.00000000000000000, -43.00000000000000000, -140.0552959529999839 ) ) ;
#21155=ORIENTED_EDGE ( 'NONE', *, *, #6889, .T. ) ;
#21159=LINE ( 'NONE', #12440, #3773 ) ;
#21161=EDGE_CURVE ( 'NONE', #7656, #16174, #2581, .T. ) ;
#21164=VERTEX_POINT ( 'NONE', #13393 ) ;
#21166=DIRECTION ( 'NONE',  ( 0.000000000000000000, 1.000000000000000000, 0.000000000000000000 ) ) ;
#21167=ORIENTED_EDGE ( 'NONE', *, *, #21302, .F. ) ;
#21168=LINE ( 'NONE', #13898, #7952 ) ;
#21170=VERTEX_POINT ( 'NONE', #11593 ) ;
#21177=ORIENTED_EDGE ( 'NONE', *, *, #25, .T. ) ;
#21181=CARTESIAN_POINT ( 'NONE',  ( 13.13369214859999978, -50.50000000000000000, -137.0552959530000123 ) ) ;
#21187=CIRCLE ( 'NONE', #10131, 2.999999999999999112 ) ;
#21189=VECTOR ( 'NONE', #12984, 1000.000000000000000 ) ;
#21192=DIRECTION ( 'NONE',  ( -1.000000000000000000, 0.000000000000000000, 0.000000000000000000 ) ) ;
#21202=LINE ( 'NONE', #18932, #16016 ) ;
#21203=VECTOR ( 'NONE', #8087, 1000.000000000000000 ) ;
#21206=DIRECTION ( 'NONE',  ( 1.000000000000000000, 0.000000000000000000, 0.000000000000000000 ) ) ;
#21212=CARTESIAN_POINT ( 'NONE',  ( 5.257235470750120321, -2.190481511161879169, -150.0552959529999839 ) ) ;
#21213=ORIENTED_EDGE ( 'NONE', *, *, #18981, .F. ) ;
#21216=ORIENTED_EDGE ( 'NONE', *, *, #20092, .T. ) ;
#21220=DIRECTION ( 'NONE',  ( 1.000000000000000000, 0.000000000000000000, 0.000000000000000000 ) ) ;
#21224=LINE ( 'NONE', #21108, #22252 ) ;
#21226=LINE ( 'NONE', #17079, #16752 ) ;
#21229=EDGE_LOOP ( 'NONE', ( #21213, #13895, #7351, #11378 ) ) ;
#21234=VECTOR ( 'NONE', #4365, 1000.000000000000000 ) ;
#21235=ORIENTED_EDGE ( 'NONE', *, *, #9133, .F. ) ;
#21237=CARTESIAN_POINT ( 'NONE',  ( 0.000000000000000000, 0.000000000000000000, -150.0552959529999839 ) ) ;
#21238=CARTESIAN_POINT ( 'NONE',  ( 25.22833163479999996, -45.34299735780000162, -149.5552959529999839 ) ) ;
#21239=AXIS2_PLACEMENT_3D ( 'NONE', #9265, #9372, #16645 ) ;
#21240=ORIENTED_EDGE ( 'NONE', *, *, #7468, .T. ) ;
#21241=LINE ( 'NONE', #4577, #19797 ) ;
#21243=CARTESIAN_POINT ( 'NONE',  ( 17.57650987475626891, 23.28094649260091842, -150.0552959529999839 ) ) ;
#21248=CARTESIAN_POINT ( 'NONE',  ( 5.257167980435379029, -4.809692093865743701, -150.0552959530000123 ) ) ;
#21249=DIRECTION ( 'NONE',  ( 1.000000000000000000, 0.000000000000000000, 0.000000000000000000 ) ) ;
#21250=AXIS2_PLACEMENT_3D ( 'NONE', #19459, #23372, #3263 ) ;
#21252=ORIENTED_EDGE ( 'NONE', *, *, #16126, .F. ) ;
#21258=DIRECTION ( 'NONE',  ( 0.000000000000000000, 0.000000000000000000, 1.000000000000000000 ) ) ;
#21261=ORIENTED_EDGE ( 'NONE', *, *, #15345, .T. ) ;
#21266=EDGE_CURVE ( 'NONE', #7656, #20624, #9807, .T. ) ;
#21272=LINE ( 'NONE', #6269, #3371 ) ;
#21273=AXIS2_PLACEMENT_3D ( 'NONE', #7690, #13164, #4127 ) ;
#21275=VECTOR ( 'NONE', #13, 1000.000000000000000 ) ;
#21279=ORIENTED_EDGE ( 'NONE', *, *, #554, .T. ) ;
#21282=ADVANCED_FACE ( 'NONE', ( #19108 ), #4471, .T. ) ;
#21285=DIRECTION ( 'NONE',  ( -2.257144641399999941E-12, 0.000000000000000000, -1.000000000000000000 ) ) ;
#21287=DIRECTION ( 'NONE',  ( 0.000000000000000000, 0.000000000000000000, 1.000000000000000000 ) ) ;
#21291=VECTOR ( 'NONE', #3153, 1000.000000000000000 ) ;
#21300=DIRECTION ( 'NONE',  ( -1.457881434569999917E-12, -1.723066134159999823E-12, 1.000000000000000000 ) ) ;
#21302=EDGE_CURVE ( 'NONE', #9978, #12270, #10041, .T. ) ;
#21304=VECTOR ( 'NONE', #5178, 1000.000000000000000 ) ;
#21306=DIRECTION ( 'NONE',  ( -1.000000000000000000, 0.000000000000000000, 0.000000000000000000 ) ) ;
#21310=VERTEX_POINT ( 'NONE', #11954 ) ;
#21313=EDGE_CURVE ( 'NONE', #17988, #1030, #22529, .T. ) ;
#21342=ORIENTED_EDGE ( 'NONE', *, *, #14639, .T. ) ;
#21345=LINE ( 'NONE', #8474, #23387 ) ;
#21346=AXIS2_PLACEMENT_3D ( 'NONE', #5534, #21615, #298 ) ;
#21353=APPLICATION_CONTEXT ( 'automotive_design' ) ;
#21360=CARTESIAN_POINT ( 'NONE',  ( 32.50000000000000000, 32.96379895129999937, -136.0552959530000123 ) ) ;
#21361=VECTOR ( 'NONE', #6782, 1000.000000000000000 ) ;
#21367=CARTESIAN_POINT ( 'NONE',  ( -12.07808196999505412, -42.21475634692215806, -150.0552959529999839 ) ) ;
#21374=EDGE_CURVE ( 'NONE', #3905, #6268, #7555, .T. ) ;
#21376=EDGE_CURVE ( 'NONE', #467, #12707, #17750, .T. ) ;
#21377=( GEOMETRIC_REPRESENTATION_CONTEXT ( 3 ) GLOBAL_UNCERTAINTY_ASSIGNED_CONTEXT ( ( #15882 ) ) GLOBAL_UNIT_ASSIGNED_CONTEXT ( ( #6140, #13758, #21609 ) ) REPRESENTATION_CONTEXT ( 'NONE', 'WORKASPACE' ) );
#21381=SHAPE_REPRESENTATION_RELATIONSHIP ( 'NONE' , 'NONE' ,  #15114, #3292 ) ;
#21387=CARTESIAN_POINT ( 'NONE',  ( -4.576509874761471863, 21.71905350741746332, -150.0552959529999839 ) ) ;
#21392=VERTEX_POINT ( 'NONE', #1465 ) ;
#21395=CARTESIAN_POINT ( 'NONE',  ( 25.31684607429999900, -45.26810052439999765, -150.0552959529999839 ) ) ;
#21398=EDGE_CURVE ( 'NONE', #567, #7407, #1881, .T. ) ;
#21399=CARTESIAN_POINT ( 'NONE',  ( -3.500000000000000000, 44.50000000000000000, -150.0552959529999839 ) ) ;
#21402=EDGE_CURVE ( 'NONE', #1705, #10837, #3351, .T. ) ;
#21404=ORIENTED_EDGE ( 'NONE', *, *, #6361, .T. ) ;
#21407=ORIENTED_EDGE ( 'NONE', *, *, #6629, .T. ) ;
#21413=CARTESIAN_POINT ( 'NONE',  ( 6.500000000000000000, 20.50000000000000000, -150.0552959529999839 ) ) ;
#21414=PLANE ( 'NONE',  #17584 ) ;
#21417=PLANE ( 'NONE',  #19329 ) ;
#21421=EDGE_LOOP ( 'NONE', ( #3807, #9764, #14312, #19523 ) ) ;
#21424=VECTOR ( 'NONE', #18278, 1000.000000000000000 ) ;
#21429=EDGE_CURVE ( 'NONE', #10756, #12039, #8815, .T. ) ;
#21445=DIRECTION ( 'NONE',  ( 1.000000000000000000, 0.000000000000000000, 2.257144641399999941E-12 ) ) ;
#21446=CARTESIAN_POINT ( 'NONE',  ( -15.50000000000000000, 21.50000000000000000, -151.0552959529999839 ) ) ;
#21448=EDGE_CURVE ( 'NONE', #1104, #21465, #18108, .T. ) ;
#21456=ORIENTED_EDGE ( 'NONE', *, *, #13640, .F. ) ;
#21462=VERTEX_POINT ( 'NONE', #3137 ) ;
#21465=VERTEX_POINT ( 'NONE', #15625 ) ;
#21468=PLANE ( 'NONE',  #3590 ) ;
#21469=ADVANCED_FACE ( 'NONE', ( #11922 ), #4913, .F. ) ;
#21471=DIRECTION ( 'NONE',  ( -1.000000000000000000, 0.000000000000000000, 0.000000000000000000 ) ) ;
#21474=CARTESIAN_POINT ( 'NONE',  ( 18.95053822279999878, -50.00000000000000000, -150.0552959529999839 ) ) ;
#21478=CARTESIAN_POINT ( 'NONE',  ( -13.15635984007525749, -40.60099947280546928, -150.0552959530000123 ) ) ;
#21486=DIRECTION ( 'NONE',  ( -0.4567501391959232770, 0.5397956190499111351, 0.7071067811858601226 ) ) ;
#21490=DIRECTION ( 'NONE',  ( 0.000000000000000000, 0.000000000000000000, 1.000000000000000000 ) ) ;
#21491=ORIENTED_EDGE ( 'NONE', *, *, #19254, .T. ) ;
#21496=CARTESIAN_POINT ( 'NONE',  ( 32.50000000000000000, 32.96379895120000469, -137.0552959530000123 ) ) ;
#21502=DIRECTION ( 'NONE',  ( 1.000000000000000000, 0.000000000000000000, -2.257157423930000049E-12 ) ) ;
#21504=ORIENTED_EDGE ( 'NONE', *, *, #15053, .T. ) ;
#21517=CARTESIAN_POINT ( 'NONE',  ( -32.50000000000000000, 51.50000000000000000, -143.3052959529999839 ) ) ;
#21518=ORIENTED_EDGE ( 'NONE', *, *, #11189, .F. ) ;
#21520=ORIENTED_EDGE ( 'NONE', *, *, #21313, .F. ) ;
#21523=ORIENTED_EDGE ( 'NONE', *, *, #10954, .F. ) ;
#21527=VECTOR ( 'NONE', #7344, 1000.000000000000000 ) ;
#21534=EDGE_CURVE ( 'NONE', #19480, #2516, #12160, .T. ) ;
#21535=CARTESIAN_POINT ( 'NONE',  ( -12.50000000000000000, 22.50000000000000000, -150.0552959529999839 ) ) ;
#21536=VERTEX_POINT ( 'NONE', #7995 ) ;
#21540=DIRECTION ( 'NONE',  ( 0.000000000000000000, 0.000000000000000000, 1.000000000000000000 ) ) ;
#21549=CARTESIAN_POINT ( 'NONE',  ( -32.50000000000000000, 14.00000000000000000, -144.0552959529999839 ) ) ;
#21550=LINE ( 'NONE', #18209, #6136 ) ;
#21551=LINE ( 'NONE', #16, #10571 ) ;
#21556=CARTESIAN_POINT ( 'NONE',  ( 6.010856941112707297, -6.121359165062768781, -150.0552959529999839 ) ) ;
#21559=DIRECTION ( 'NONE',  ( -1.000000000000000000, 0.000000000000000000, 0.000000000000000000 ) ) ;
#21561=ORIENTED_EDGE ( 'NONE', *, *, #2941, .F. ) ;
#21562=EDGE_CURVE ( 'NONE', #20932, #12200, #21649, .T. ) ;
#21566=EDGE_CURVE ( 'NONE', #10756, #14446, #1134, .T. ) ;
#21573=DIRECTION ( 'NONE',  ( -1.000000000000000000, 0.000000000000000000, 0.000000000000000000 ) ) ;
#21577=CARTESIAN_POINT ( 'NONE',  ( -1.000000000000000000, 20.50000000000000000, -150.0552959529999839 ) ) ;
#21578=CIRCLE ( 'NONE', #12428, 0.4999999999999987788 ) ;
#21590=DIRECTION ( 'NONE',  ( -1.000000000000000000, 0.000000000000000000, 0.000000000000000000 ) ) ;
#21596=CARTESIAN_POINT ( 'NONE',  ( 18.98502865237968606, 25.11890206003841541, -150.0552959529999839 ) ) ;
#21600=EDGE_CURVE ( 'NONE', #12372, #3522, #12896, .T. ) ;
#21603=DIRECTION ( 'NONE',  ( 0.7633862853691872896, 0.6459422414660880296, -5.370703881624201706E-14 ) ) ;
#21605=CARTESIAN_POINT ( 'NONE',  ( 14.00000000000000000, 20.50000000000000000, -151.0552959529999839 ) ) ;
#21606=ORIENTED_EDGE ( 'NONE', *, *, #2549, .T. ) ;
#21609=( NAMED_UNIT ( * ) SI_UNIT ( $, .STERADIAN. ) SOLID_ANGLE_UNIT ( ) );
#21612=VECTOR ( 'NONE', #22921, 1000.000000000000000 ) ;
#21615=DIRECTION ( 'NONE',  ( -0.000000000000000000, 1.000000000000000000, 0.000000000000000000 ) ) ;
#21616=DIRECTION ( 'NONE',  ( 0.000000000000000000, 1.000000000000000000, 0.000000000000000000 ) ) ;
#21621=ADVANCED_FACE ( 'NONE', ( #14656 ), #21926, .F. ) ;
#21635=DIRECTION ( 'NONE',  ( 0.000000000000000000, 0.000000000000000000, 1.000000000000000000 ) ) ;
#21639=ORIENTED_EDGE ( 'NONE', *, *, #20164, .T. ) ;
#21641=EDGE_CURVE ( 'NONE', #12270, #1424, #14772, .T. ) ;
#21643=EDGE_CURVE ( 'NONE', #12394, #7397, #20259, .T. ) ;
#21644=CARTESIAN_POINT ( 'NONE',  ( -3.765209112811370051, 42.50000000000000711, -150.0552959530000123 ) ) ;
#21648=DIRECTION ( 'NONE',  ( 0.000000000000000000, 1.000000000000000000, 0.000000000000000000 ) ) ;
#21649=CIRCLE ( 'NONE', #11348, 0.5000000000000004441 ) ;
#21655=AXIS2_PLACEMENT_3D ( 'NONE', #5024, #23108, #17747 ) ;
#21658=EDGE_LOOP ( 'NONE', ( #18986, #4243, #10817, #3208 ) ) ;
#21670=VECTOR ( 'NONE', #1017, 1000.000000000000000 ) ;
#21672=AXIS2_PLACEMENT_3D ( 'NONE', #21237, #9785, #17185 ) ;
#21678=FACE_OUTER_BOUND ( 'NONE', #6465, .T. ) ;
#21683=CARTESIAN_POINT ( 'NONE',  ( -32.50000000000000000, -51.50000000000000000, -142.8052959529999839 ) ) ;
#21691=VECTOR ( 'NONE', #19597, 1000.000000000000000 ) ;
#21706=EDGE_CURVE ( 'NONE', #5909, #13263, #9982, .T. ) ;
#21709=ORIENTED_EDGE ( 'NONE', *, *, #17610, .T. ) ;
#21712=DIRECTION ( 'NONE',  ( 0.000000000000000000, -1.000000000000000000, 0.000000000000000000 ) ) ;
#21716=ORIENTED_EDGE ( 'NONE', *, *, #21831, .T. ) ;
#21718=CARTESIAN_POINT ( 'NONE',  ( 20.10234832539997285, 19.49999999999999645, -150.0552959530000123 ) ) ;
#21719=DIRECTION ( 'NONE',  ( 0.000000000000000000, 1.000000000000000000, -2.245315044929999938E-12 ) ) ;
#21739=VERTEX_POINT ( 'NONE', #11646 ) ;
#21742=LINE ( 'NONE', #5430, #22812 ) ;
#21744=CARTESIAN_POINT ( 'NONE',  ( 18.95053822279999878, 50.00000000000000000, -149.5552959529999839 ) ) ;
#21750=CARTESIAN_POINT ( 'NONE',  ( -6.683153925719999222, 51.50000000000000000, -136.0552959530000123 ) ) ;
#21752=STYLED_ITEM ( 'NONE', ( #8261 ), #3292 ) ;
#21753=ORIENTED_EDGE ( 'NONE', *, *, #6126, .T. ) ;
#21762=DIRECTION ( 'NONE',  ( -1.000000000000000000, 0.000000000000000000, 2.257144641399999941E-12 ) ) ;
#21763=ORIENTED_EDGE ( 'NONE', *, *, #20092, .F. ) ;
#21765=LINE ( 'NONE', #18179, #4513 ) ;
#21771=CARTESIAN_POINT ( 'NONE',  ( 31.50000000000000000, -40.03620104880000241, -136.0552959530000123 ) ) ;
#21772=EDGE_LOOP ( 'NONE', ( #21056, #15639, #21806, #21504 ) ) ;
#21778=PLANE ( 'NONE',  #6412 ) ;
#21791=PLANE ( 'NONE',  #18844 ) ;
#21795=DIRECTION ( 'NONE',  ( 0.7633862853691522066, 0.6459422414661292189, 1.795096815436260566E-28 ) ) ;
#21799=FACE_OUTER_BOUND ( 'NONE', #13865, .T. ) ;
#21801=DIRECTION ( 'NONE',  ( 1.000000000000000000, 0.000000000000000000, 0.000000000000000000 ) ) ;
#21804=DIRECTION ( 'NONE',  ( 0.000000000000000000, 1.000000000000000000, -2.245315044929999938E-12 ) ) ;
#21806=ORIENTED_EDGE ( 'NONE', *, *, #16339, .F. ) ;
#21807=EDGE_CURVE ( 'NONE', #350, #15992, #17492, .T. ) ;
#21813=CARTESIAN_POINT ( 'NONE',  ( 1.133692148550000001, 50.50000000000000000, -136.0552959530000123 ) ) ;
#21819=PLANE ( 'NONE',  #13213 ) ;
#21821=VERTEX_POINT ( 'NONE', #14039 ) ;
#21822=CARTESIAN_POINT ( 'NONE',  ( -12.50000000000000000, 19.50000000000000000, -151.0552959529999839 ) ) ;
#21828=PLANE ( 'NONE',  #9860 ) ;
#21831=EDGE_CURVE ( 'NONE', #844, #21875, #12125, .T. ) ;
#21834=DIRECTION ( 'NONE',  ( -1.000000000000000000, 0.000000000000000000, 2.257144641399999941E-12 ) ) ;
#21840=CARTESIAN_POINT ( 'NONE',  ( 15.50000000000000000, 39.50000000000000000, -150.0552959529999839 ) ) ;
#21842=DIRECTION ( 'NONE',  ( 0.000000000000000000, 1.000000000000000000, 0.000000000000000000 ) ) ;
#21845=CARTESIAN_POINT ( 'NONE',  ( -31.50000000000000000, -24.50000000000000000, -150.0552959529999839 ) ) ;
#21846=ORIENTED_EDGE ( 'NONE', *, *, #18534, .F. ) ;
#21850=ORIENTED_EDGE ( 'NONE', *, *, #20534, .F. ) ;
#21852=PLANE ( 'NONE',  #21346 ) ;
#21853=ORIENTED_EDGE ( 'NONE', *, *, #16797, .T. ) ;
#21856=CARTESIAN_POINT ( 'NONE',  ( -5.098088255175412087, 24.33948587670916908, -150.0552959529999839 ) ) ;
#21859=ORIENTED_EDGE ( 'NONE', *, *, #8509, .F. ) ;
#21861=EDGE_CURVE ( 'NONE', #18962, #6192, #16301, .T. ) ;
#21866=DIRECTION ( 'NONE',  ( 0.7633862853691524286, -0.6459422414661292189, 2.747801985950550015E-15 ) ) ;
#21867=ORIENTED_EDGE ( 'NONE', *, *, #19817, .F. ) ;
#21868=EDGE_CURVE ( 'NONE', #12270, #2516, #18083, .T. ) ;
#21869=DIRECTION ( 'NONE',  ( 0.000000000000000000, 0.000000000000000000, 1.000000000000000000 ) ) ;
#21875=VERTEX_POINT ( 'NONE', #8785 ) ;
#21880=EDGE_CURVE ( 'NONE', #7890, #3203, #6774, .T. ) ;
#21881=ORIENTED_EDGE ( 'NONE', *, *, #2124, .F. ) ;
#21887=EDGE_LOOP ( 'NONE', ( #11716, #15890, #10138, #7042 ) ) ;
#21891=VECTOR ( 'NONE', #1624, 1000.000000000000227 ) ;
#21895=DIRECTION ( 'NONE',  ( 1.000000000000000000, 0.000000000000000000, 0.000000000000000000 ) ) ;
#21902=FACE_BOUND ( 'NONE', #12204, .T. ) ;
#21912=CARTESIAN_POINT ( 'NONE',  ( 2.989143058887309135, -6.121359165062779439, -150.0552959529999839 ) ) ;
#21919=EDGE_CURVE ( 'NONE', #12787, #6002, #9139, .T. ) ;
#21920=CARTESIAN_POINT ( 'NONE',  ( 3.000000000000000888, -3.300910577262573309, -150.0552959529999839 ) ) ;
#21921=ORIENTED_EDGE ( 'NONE', *, *, #3184, .F. ) ;
#21926=PLANE ( 'NONE',  #17071 ) ;
#21932=DIRECTION ( 'NONE',  ( -2.257144641399999941E-12, 0.000000000000000000, 1.000000000000000000 ) ) ;
#21940=EDGE_LOOP ( 'NONE', ( #3850, #13204, #12579, #13695 ) ) ;
#21945=DIRECTION ( 'NONE',  ( 0.000000000000000000, 1.000000000000000000, -2.245315044929999938E-12 ) ) ;
#21946=CARTESIAN_POINT ( 'NONE',  ( -13.79914019398160896, -43.91988638304457737, -150.0552959529999839 ) ) ;
#21950=CARTESIAN_POINT ( 'NONE',  ( 31.00000000000000000, 39.80430157320000006, -151.0552959529999839 ) ) ;
#21954=CARTESIAN_POINT ( 'NONE',  ( 25.50000000000000000, 22.50000000000000000, -151.0552959529999839 ) ) ;
#21958=VERTEX_POINT ( 'NONE', #16758 ) ;
#21959=DIRECTION ( 'NONE',  ( 0.000000000000000000, 0.000000000000000000, 1.000000000000000000 ) ) ;
#21961=FACE_OUTER_BOUND ( 'NONE', #18474, .T. ) ;
#21967=EDGE_LOOP ( 'NONE', ( #22692, #13078, #14950, #12541 ) ) ;
#21980=EDGE_LOOP ( 'NONE', ( #8293, #18277, #19825, #6143 ) ) ;
#21990=CARTESIAN_POINT ( 'NONE',  ( 8.915777720172247456, 27.61753626548571106, -150.0552959529999555 ) ) ;
#22003=CARTESIAN_POINT ( 'NONE',  ( -31.50000000000000000, 1.000000000000000000, -137.0552959530000123 ) ) ;
#22018=ORIENTED_EDGE ( 'NONE', *, *, #11989, .T. ) ;
#22020=CARTESIAN_POINT ( 'NONE',  ( 8.750000000000000000, -39.23606797749999942, -151.0552959529999839 ) ) ;
#22038=EDGE_CURVE ( 'NONE', #328, #23438, #11427, .T. ) ;
#22042=LINE ( 'NONE', #9395, #14331 ) ;
#22045=CARTESIAN_POINT ( 'NONE',  ( 19.91945158500000090, 51.14507942810000429, -149.8052959529999839 ) ) ;
#22053=VECTOR ( 'NONE', #13854, 1000.000000000000227 ) ;
#22054=VECTOR ( 'NONE', #19863, 1000.000000000000000 ) ;
#22059=FACE_OUTER_BOUND ( 'NONE', #12700, .T. ) ;
#22060=CARTESIAN_POINT ( 'NONE',  ( -13.50000000000000000, -43.00000000000000000, -150.0552959529999839 ) ) ;
#22065=CARTESIAN_POINT ( 'NONE',  ( 31.50000000020000002, -40.03620104850000416, -143.0552959529999839 ) ) ;
#22067=CARTESIAN_POINT ( 'NONE',  ( 12.88103053855259894, 34.98519100496140766, -150.0552959529999839 ) ) ;
#22069=AXIS2_PLACEMENT_3D ( 'NONE', #19255, #1637, #22838 ) ;
#22071=VECTOR ( 'NONE', #19005, 1000.000000000000000 ) ;
#22078=CARTESIAN_POINT ( 'NONE',  ( -31.75000000000000000, -36.00000000000000000, -151.0552959529999839 ) ) ;
#22081=CARTESIAN_POINT ( 'NONE',  ( 13.13369214859999978, 50.50000000000000000, -136.0552959530000123 ) ) ;
#22084=AXIS2_PLACEMENT_3D ( 'NONE', #18890, #20682, #20927 ) ;
#22090=EDGE_CURVE ( 'NONE', #16889, #5668, #19436, .T. ) ;
#22091=DIRECTION ( 'NONE',  ( 0.7071067811870332953, 0.000000000000000000, 0.7071067811860618502 ) ) ;
#22096=VECTOR ( 'NONE', #9558, 1000.000000000000000 ) ;
#22103=CARTESIAN_POINT ( 'NONE',  ( -13.48914305888729004, -45.62135916506274924, -150.0552959529999555 ) ) ;
#22104=EDGE_LOOP ( 'NONE', ( #20968, #6300, #5933, #15402 ) ) ;
#22109=CARTESIAN_POINT ( 'NONE',  ( 14.00000000000000000, 20.50000000000000000, -150.0552959529999839 ) ) ;
#22114=CARTESIAN_POINT ( 'NONE',  ( 7.500000000000000000, -3.500000000000000000, -145.5552959529999839 ) ) ;
#22118=EDGE_CURVE ( 'NONE', #16851, #16174, #15217, .T. ) ;
#22122=DIRECTION ( 'NONE',  ( 0.000000000000000000, 0.000000000000000000, 1.000000000000000000 ) ) ;
#22128=FACE_OUTER_BOUND ( 'NONE', #3174, .T. ) ;
#22130=DIRECTION ( 'NONE',  ( 1.000000000000000000, 0.000000000000000000, 0.000000000000000000 ) ) ;
#22136=VECTOR ( 'NONE', #11631, 1000.000000000000000 ) ;
#22138=CARTESIAN_POINT ( 'NONE',  ( 32.50000000000000000, -33.03620104880000241, -137.0552959530000123 ) ) ;
#22144=CARTESIAN_POINT ( 'NONE',  ( -32.50000000000000000, 50.00000000000000000, -150.0552959529999839 ) ) ;
#22148=ORIENTED_EDGE ( 'NONE', *, *, #12290, .F. ) ;
#22162=DIRECTION ( 'NONE',  ( 1.000000000000000000, 0.000000000000000000, 0.000000000000000000 ) ) ;
#22179=DIRECTION ( 'NONE',  ( -1.457881434619999915E-12, -1.723066134219999902E-12, 1.000000000000000000 ) ) ;
#22182=CARTESIAN_POINT ( 'NONE',  ( 4.523700915356613450, -38.03365992288669162, -150.0552959530000123 ) ) ;
#22183=ADVANCED_FACE ( 'NONE', ( #10771 ), #1653, .F. ) ;
#22184=EDGE_LOOP ( 'NONE', ( #3319, #6627, #5019, #21404 ) ) ;
#22187=ORIENTED_EDGE ( 'NONE', *, *, #10257, .T. ) ;
#22198=ORIENTED_EDGE ( 'NONE', *, *, #22788, .T. ) ;
#22200=ADVANCED_FACE ( 'NONE', ( #12328 ), #3421, .F. ) ;
#22201=AXIS2_PLACEMENT_3D ( 'NONE', #19536, #8677, #17629 ) ;
#22209=CARTESIAN_POINT ( 'NONE',  ( 5.004065293326166675, -48.00992235983122924, -150.0552959529999839 ) ) ;
#22211=DIRECTION ( 'NONE',  ( -1.000000000000000000, 0.000000000000000000, 0.000000000000000000 ) ) ;
#22215=EDGE_LOOP ( 'NONE', ( #13328, #20398, #10770, #20661 ) ) ;
#22216=FACE_OUTER_BOUND ( 'NONE', #15322, .T. ) ;
#22219=ORIENTED_EDGE ( 'NONE', *, *, #12290, .T. ) ;
#22221=CARTESIAN_POINT ( 'NONE',  ( -32.50000000000000000, 19.50000000000000000, -150.0552959529999839 ) ) ;
#22223=PLANE ( 'NONE',  #12237 ) ;
#22225=LINE ( 'NONE', #7809, #10647 ) ;
#22232=CARTESIAN_POINT ( 'NONE',  ( 3.000000000000000000, -3.698737831368826612, -150.0552959530000408 ) ) ;
#22234=CARTESIAN_POINT ( 'NONE',  ( 19.13369214859999801, 51.50000000000000000, -142.8052959529999839 ) ) ;
#22241=DIRECTION ( 'NONE',  ( 1.000000000000000000, 0.000000000000000000, 0.000000000000000000 ) ) ;
#22249=EDGE_CURVE ( 'NONE', #328, #5806, #23293, .T. ) ;
#22251=CARTESIAN_POINT ( 'NONE',  ( 32.00000000000000000, 20.96379895120000114, -137.0552959530000123 ) ) ;
#22252=VECTOR ( 'NONE', #6577, 1000.000000000000000 ) ;
#22259=ORIENTED_EDGE ( 'NONE', *, *, #21023, .F. ) ;
#22262=DIRECTION ( 'NONE',  ( 0.000000000000000000, -1.000000000000000000, 0.000000000000000000 ) ) ;
#22265=VERTEX_POINT ( 'NONE', #8874 ) ;
#22266=CARTESIAN_POINT ( 'NONE',  ( -32.00000000000000000, -50.00000000000000000, -137.0552959530000123 ) ) ;
#22268=CYLINDRICAL_SURFACE ( 'NONE', #20736, 0.4999999999999936717 ) ;
#22275=DIRECTION ( 'NONE',  ( 1.000000000000000000, 0.000000000000000000, 0.000000000000000000 ) ) ;
#22278=CARTESIAN_POINT ( 'NONE',  ( -25.86630785139999844, -51.00000000000000000, -137.0552959530000123 ) ) ;
#22280=ORIENTED_EDGE ( 'NONE', *, *, #13351, .F. ) ;
#22282=FACE_BOUND ( 'NONE', #15108, .T. ) ;
#22292=PLANE ( 'NONE',  #10519 ) ;
#22297=AXIS2_PLACEMENT_3D ( 'NONE', #7422, #6955, #21842 ) ;
#22299=ORIENTED_EDGE ( 'NONE', *, *, #8625, .T. ) ;
#22300=ORIENTED_EDGE ( 'NONE', *, *, #2250, .T. ) ;
#22303=CARTESIAN_POINT ( 'NONE',  ( 31.50000000000000000, 32.96379895120000469, -137.0552959530000123 ) ) ;
#22320=CARTESIAN_POINT ( 'NONE',  ( 8.750000000000000000, -47.00000000000000000, -150.0552959529999839 ) ) ;
#22324=FILL_AREA_STYLE ('',( #11710 ) ) ;
#22325=ORIENTED_EDGE ( 'NONE', *, *, #19235, .F. ) ;
#22327=EDGE_CURVE ( 'NONE', #11744, #11360, #1886, .T. ) ;
#22330=CARTESIAN_POINT ( 'NONE',  ( -12.00000000000000000, -43.00000000000000000, -150.0552959529999839 ) ) ;
#22335=CARTESIAN_POINT ( 'NONE',  ( 6.500000000000000000, 28.00000000000000000, -150.0552959529999839 ) ) ;
#22336=CARTESIAN_POINT ( 'NONE',  ( 31.50000000000000000, -21.03620104879999886, -137.0552959530000123 ) ) ;
#22339=EDGE_LOOP ( 'NONE', ( #23255, #22486, #20547, #13191 ) ) ;
#22347=ADVANCED_FACE ( 'NONE', ( #316 ), #438, .T. ) ;
#22349=ADVANCED_FACE ( 'NONE', ( #1767 ), #13151, .T. ) ;
#22359=CARTESIAN_POINT ( 'NONE',  ( -32.50000000000000000, 0.000000000000000000, -150.0552959529999839 ) ) ;
#22374=FACE_OUTER_BOUND ( 'NONE', #18622, .T. ) ;
#22376=EDGE_LOOP ( 'NONE', ( #9043, #9902, #7983, #7089 ) ) ;
#22379=EDGE_CURVE ( 'NONE', #14539, #17914, #16391, .T. ) ;
#22382=PLANE ( 'NONE',  #20422 ) ;
#22387=CIRCLE ( 'NONE', #13646, 0.5000000000000004441 ) ;
#22394=CARTESIAN_POINT ( 'NONE',  ( 23.00000000000000000, 19.50000000000000000, -150.0552959529999839 ) ) ;
#22395=CARTESIAN_POINT ( 'NONE',  ( 13.13369214859999978, -51.50000000000000000, -136.5552959530000123 ) ) ;
#22400=VECTOR ( 'NONE', #5695, 1000.000000000000000 ) ;
#22403=AXIS2_PLACEMENT_3D ( 'NONE', #13768, #6504, #12788 ) ;
#22410=EDGE_CURVE ( 'NONE', #10473, #6870, #8987, .T. ) ;
#22412=DIRECTION ( 'NONE',  ( -2.257144641399999941E-12, 0.000000000000000000, -1.000000000000000000 ) ) ;
#22416=CARTESIAN_POINT ( 'NONE',  ( 4.750000000000000000, -42.61803398880000060, -151.0552959529999839 ) ) ;
#22419=VECTOR ( 'NONE', #7245, 1000.000000000000000 ) ;
#22434=VECTOR ( 'NONE', #9062, 1000.000000000000000 ) ;
#22437=ADVANCED_FACE ( 'NONE', ( #11017 ), #11234, .T. ) ;
#22442=VERTEX_POINT ( 'NONE', #19954 ) ;
#22449=EDGE_LOOP ( 'NONE', ( #7518, #7154, #4320, #16401 ) ) ;
#22453=CARTESIAN_POINT ( 'NONE',  ( 22.50000000000000000, 39.50000000000000000, -150.0552959529999839 ) ) ;
#22456=CARTESIAN_POINT ( 'NONE',  ( -32.50000000000000000, 50.50000000000000000, -137.0552959530000123 ) ) ;
#22457=EDGE_CURVE ( 'NONE', #20386, #3522, #9109, .T. ) ;
#22466=EDGE_LOOP ( 'NONE', ( #19043, #7867, #19931, #17236 ) ) ;
#22467=VECTOR ( 'NONE', #2449, 1000.000000000000000 ) ;
#22486=ORIENTED_EDGE ( 'NONE', *, *, #17610, .F. ) ;
#22493=EDGE_LOOP ( 'NONE', ( #2742, #12446 ) ) ;
#22496=EDGE_CURVE ( 'NONE', #4521, #18822, #21226, .T. ) ;
#22497=LINE ( 'NONE', #14885, #19695 ) ;
#22498=ORIENTED_EDGE ( 'NONE', *, *, #368, .F. ) ;
#22503=LINE ( 'NONE', #613, #15107 ) ;
#22509=VECTOR ( 'NONE', #571, 1000.000000000000000 ) ;
#22516=DIRECTION ( 'NONE',  ( 1.000000000000000000, 0.000000000000000000, 0.000000000000000000 ) ) ;
#22521=ADVANCED_FACE ( 'NONE', ( #7789 ), #22560, .T. ) ;
#22529=LINE ( 'NONE', #11446, #4159 ) ;
#22542=EDGE_CURVE ( 'NONE', #14976, #3870, #6812, .T. ) ;
#22544=ADVANCED_FACE ( 'NONE', ( #12044 ), #6249, .T. ) ;
#22546=EDGE_CURVE ( 'NONE', #12137, #3906, #9799, .T. ) ;
#22560=PLANE ( 'NONE',  #15253 ) ;
#22563=ORIENTED_EDGE ( 'NONE', *, *, #5889, .F. ) ;
#22565=CARTESIAN_POINT ( 'NONE',  ( -7.520331543250000195, 50.50000000000000000, -136.0552959530000123 ) ) ;
#22566=ORIENTED_EDGE ( 'NONE', *, *, #14869, .F. ) ;
#22568=VERTEX_POINT ( 'NONE', #8476 ) ;
#22592=CARTESIAN_POINT ( 'NONE',  ( 22.71475634692216516, -23.42191803000494588, -150.0552959529999839 ) ) ;
#22593=VERTEX_POINT ( 'NONE', #4352 ) ;
#22611=DIRECTION ( 'NONE',  ( 0.000000000000000000, 0.000000000000000000, 1.000000000000000000 ) ) ;
#22626=EDGE_CURVE ( 'NONE', #1030, #4038, #14431, .T. ) ;
#22630=ORIENTED_EDGE ( 'NONE', *, *, #7780, .F. ) ;
#22637=AXIS2_PLACEMENT_3D ( 'NONE', #5757, #20284, #414 ) ;
#22638=VECTOR ( 'NONE', #19334, 1000.000000000000000 ) ;
#22643=CARTESIAN_POINT ( 'NONE',  ( 0.8488229453495553800, 15.54483228932120120, -150.0552959529999839 ) ) ;
#22644=DIRECTION ( 'NONE',  ( 0.000000000000000000, 0.000000000000000000, 1.000000000000000000 ) ) ;
#22649=EDGE_CURVE ( 'NONE', #20697, #12372, #16336, .T. ) ;
#22650=EDGE_LOOP ( 'NONE', ( #9831, #5949, #15698, #15398 ) ) ;
#22654=CARTESIAN_POINT ( 'NONE',  ( 6.500000000000000000, 20.50000000000000000, -151.0552959529999839 ) ) ;
#22665=VECTOR ( 'NONE', #23023, 1000.000000000000227 ) ;
#22667=CARTESIAN_POINT ( 'NONE',  ( 0.000000000000000000, 33.50000000000000000, -150.0552959529999839 ) ) ;
#22679=VECTOR ( 'NONE', #22179, 1000.000000000000000 ) ;
#22680=ORIENTED_EDGE ( 'NONE', *, *, #21448, .F. ) ;
#22681=DIRECTION ( 'NONE',  ( 0.000000000000000000, -1.000000000000000000, 0.000000000000000000 ) ) ;
#22682=LINE ( 'NONE', #11962, #3431 ) ;
#22683=CARTESIAN_POINT ( 'NONE',  ( 23.50000000000000000, -20.50000000000000000, -135.0552959530000123 ) ) ;
#22691=CARTESIAN_POINT ( 'NONE',  ( 24.01462304342504339, 39.11919234682564195, -150.0552959530000123 ) ) ;
#22692=ORIENTED_EDGE ( 'NONE', *, *, #1313, .T. ) ;
#22700=ADVANCED_FACE ( 'NONE', ( #13100 ), #4067, .F. ) ;
#22708=EDGE_LOOP ( 'NONE', ( #14393, #17360, #10799, #15494 ) ) ;
#22710=VERTEX_POINT ( 'NONE', #9635 ) ;
#22721=EDGE_LOOP ( 'NONE', ( #5399, #3328, #7338, #11734 ) ) ;
#22724=LINE ( 'NONE', #2756, #21203 ) ;
#22731=CARTESIAN_POINT ( 'NONE',  ( 25.89900052719454493, -18.65635984007525394, -150.0552959529999839 ) ) ;
#22735=VECTOR ( 'NONE', #9230, 1000.000000000000000 ) ;
#22737=PLANE ( 'NONE',  #1225 ) ;
#22745=CARTESIAN_POINT ( 'NONE',  ( 5.961649142145938995, -3.109383212426971355, -150.0552959530000123 ) ) ;
#22750=EDGE_CURVE ( 'NONE', #20332, #2028, #2177, .T. ) ;
#22751=VECTOR ( 'NONE', #11898, 1000.000000000000000 ) ;
#22754=VERTEX_POINT ( 'NONE', #7742 ) ;
#22755=AXIS2_PLACEMENT_3D ( 'NONE', #171, #7644, #2082 ) ;
#22764=CARTESIAN_POINT ( 'NONE',  ( 25.31684607440000079, 45.26810052429999587, -150.0552959529999839 ) ) ;
#22767=AXIS2_PLACEMENT_3D ( 'NONE', #14183, #17637, #1463 ) ;
#22769=VECTOR ( 'NONE', #20865, 1000.000000000000000 ) ;
#22770=ORIENTED_EDGE ( 'NONE', *, *, #2362, .T. ) ;
#22776=EDGE_LOOP ( 'NONE', ( #20430, #18508, #19904, #18381, #19174, #14860, #1397, #19225, #10952, #22680, #9049, #8951, #806, #21167, #7760 ) ) ;
#22786=LINE ( 'NONE', #4346, #15181 ) ;
#22788=EDGE_CURVE ( 'NONE', #12707, #6962, #15474, .T. ) ;
#22794=CIRCLE ( 'NONE', #21273, 3.000000000000000000 ) ;
#22797=VERTEX_POINT ( 'NONE', #11651 ) ;
#22812=VECTOR ( 'NONE', #12675, 1000.000000000000000 ) ;
#22818=ORIENTED_EDGE ( 'NONE', *, *, #20869, .T. ) ;
#22819=PLANE ( 'NONE',  #5270 ) ;
#22820=EDGE_CURVE ( 'NONE', #11337, #20932, #12133, .T. ) ;
#22824=PLANE ( 'NONE',  #11672 ) ;
#22828=AXIS2_PLACEMENT_3D ( 'NONE', #3576, #240, #7480 ) ;
#22829=VECTOR ( 'NONE', #18256, 1000.000000000000000 ) ;
#22833=ORIENTED_EDGE ( 'NONE', *, *, #13015, .T. ) ;
#22836=ORIENTED_EDGE ( 'NONE', *, *, #1267, .T. ) ;
#22838=DIRECTION ( 'NONE',  ( 0.000000000000000000, 0.000000000000000000, 1.000000000000000000 ) ) ;
#22842=ORIENTED_EDGE ( 'NONE', *, *, #5183, .F. ) ;
#22845=ORIENTED_EDGE ( 'NONE', *, *, #18534, .T. ) ;
#22848=DIRECTION ( 'NONE',  ( 2.257252162960000001E-12, 0.000000000000000000, 1.000000000000000000 ) ) ;
#22853=VERTEX_POINT ( 'NONE', #17499 ) ;
#22862=CARTESIAN_POINT ( 'NONE',  ( 22.71475634692216161, -17.57808196999505768, -150.0552959529999839 ) ) ;
#22866=VECTOR ( 'NONE', #10601, 1000.000000000000000 ) ;
#22869=DIRECTION ( 'NONE',  ( 0.000000000000000000, -1.000000000000000000, 0.000000000000000000 ) ) ;
#22874=ORIENTED_EDGE ( 'NONE', *, *, #8018, .F. ) ;
#22883=AXIS2_PLACEMENT_3D ( 'NONE', #23533, #8528, #23065 ) ;
#22891=CARTESIAN_POINT ( 'NONE',  ( -0.6176558849483760882, 18.08432684250963263, -150.0552959529999555 ) ) ;
#22894=CARTESIAN_POINT ( 'NONE',  ( 0.5374248537122892078, 25.07581004119178658, -150.0552959529999839 ) ) ;
#22895=CARTESIAN_POINT ( 'NONE',  ( 4.579308732360918732, -33.90724429028959008, -150.0552959529999839 ) ) ;
#22896=ORIENTED_EDGE ( 'NONE', *, *, #2143, .T. ) ;
#22898=EDGE_CURVE ( 'NONE', #9410, #1301, #13450, .T. ) ;
#22915=CARTESIAN_POINT ( 'NONE',  ( 6.000000000000001776, -3.699089422736518085, -150.0552959530000123 ) ) ;
#22918=FACE_OUTER_BOUND ( 'NONE', #9997, .T. ) ;
#22919=CIRCLE ( 'NONE', #16443, 1.500000000000001332 ) ;
#22921=DIRECTION ( 'NONE',  ( 0.000000000000000000, -1.000000000000000000, 0.000000000000000000 ) ) ;
#22922=ORIENTED_EDGE ( 'NONE', *, *, #6753, .F. ) ;
#22924=EDGE_CURVE ( 'NONE', #10612, #384, #4886, .T. ) ;
#22926=DIRECTION ( 'NONE',  ( 0.000000000000000000, 0.000000000000000000, 1.000000000000000000 ) ) ;
#22928=ORIENTED_EDGE ( 'NONE', *, *, #22249, .F. ) ;
#22929=LINE ( 'NONE', #15667, #14066 ) ;
#22930=LINE ( 'NONE', #6847, #63 ) ;
#22950=LINE ( 'NONE', #9956, #3273 ) ;
#22956=EDGE_CURVE ( 'NONE', #1104, #13536, #5007, .T. ) ;
#22969=CARTESIAN_POINT ( 'NONE',  ( 7.500000000000000000, -3.500000000000000000, -150.0552959529999839 ) ) ;
#22973=ORIENTED_EDGE ( 'NONE', *, *, #14411, .T. ) ;
#22974=CARTESIAN_POINT ( 'NONE',  ( -32.50000000000000000, 1.000000000000000000, -137.0552959530000123 ) ) ;
#22975=DIRECTION ( 'NONE',  ( 1.000000000000000000, 0.000000000000000000, 0.000000000000000000 ) ) ;
#22977=CARTESIAN_POINT ( 'NONE',  ( 23.00000000000000000, 19.50000000000000000, -150.0552959529999839 ) ) ;
#22980=CARTESIAN_POINT ( 'NONE',  ( 16.13369214839999799, 51.50000000000000000, -136.0552959530000123 ) ) ;
#22981=VERTEX_POINT ( 'NONE', #3692 ) ;
#22987=ORIENTED_EDGE ( 'NONE', *, *, #13531, .T. ) ;
#22997=FACE_OUTER_BOUND ( 'NONE', #16583, .T. ) ;
#22999=VECTOR ( 'NONE', #2033, 1000.000000000000000 ) ;
#23008=EDGE_CURVE ( 'NONE', #16273, #2045, #21550, .T. ) ;
#23010=B_SPLINE_CURVE_WITH_KNOTS ( 'NONE', 3,
 ( #17193, #22232, #6247, #12828, #13496, #20101, #11153, #3803, #17557, #20896, #15527, #21248, #1273, #6490, #17427, #8604, #22915, #19100 ),
 .UNSPECIFIED., .F., .F.,
 ( 4, 2, 2, 2, 2, 2, 2, 2, 4 ),
 ( 0.000000000000000000, 0.1249999999999998612, 0.2499999999999997224, 0.3749999999999995559, 0.4999999999999992228, 0.6249999999999994449, 0.7499999999999995559, 0.8749999999999997780, 1.000000000000000000 ),
 .UNSPECIFIED. ) ;
#23011=ORIENTED_EDGE ( 'NONE', *, *, #17652, .T. ) ;
#23017=LINE ( 'NONE', #21238, #22053 ) ;
#23019=CIRCLE ( 'NONE', #13503, 2.999999999999999112 ) ;
#23023=DIRECTION ( 'NONE',  ( -0.6459422414661291079, 0.7633862853691523176, -2.245315045000450442E-12 ) ) ;
#23025=ADVANCED_FACE ( 'NONE', ( #1687 ), #15828, .F. ) ;
#23026=DIRECTION ( 'NONE',  ( -1.000000000000000000, 0.000000000000000000, 0.000000000000000000 ) ) ;
#23037=ORIENTED_EDGE ( 'NONE', *, *, #14777, .F. ) ;
#23038=DIRECTION ( 'NONE',  ( 0.000000000000000000, 2.256988247090000272E-12, 1.000000000000000000 ) ) ;
#23044=DIRECTION ( 'NONE',  ( 0.000000000000000000, 1.000000000000000000, 0.000000000000000000 ) ) ;
#23046=CARTESIAN_POINT ( 'NONE',  ( 15.50000000000000000, 39.50000000000000000, -150.0552959529999839 ) ) ;
#23059=DIRECTION ( 'NONE',  ( -2.257144641399999941E-12, 0.000000000000000000, -1.000000000000000000 ) ) ;
#23062=CARTESIAN_POINT ( 'NONE',  ( 31.50000000000000000, 0.000000000000000000, -136.0552959530000123 ) ) ;
#23063=ORIENTED_EDGE ( 'NONE', *, *, #1180, .F. ) ;
#23065=DIRECTION ( 'NONE',  ( 0.000000000000000000, 0.000000000000000000, 1.000000000000000000 ) ) ;
#23066=EDGE_LOOP ( 'NONE', ( #8238, #7096, #9715, #11817 ) ) ;
#23081=EDGE_CURVE ( 'NONE', #10244, #16283, #7138, .T. ) ;
#23090=CARTESIAN_POINT ( 'NONE',  ( -7.520331543250000195, 50.50000000000000000, -136.0552959530000123 ) ) ;
#23096=CIRCLE ( 'NONE', #5612, 1.500000000000001332 ) ;
#23097=LINE ( 'NONE', #8674, #20878 ) ;
#23102=ORIENTED_EDGE ( 'NONE', *, *, #9679, .T. ) ;
#23105=VERTEX_POINT ( 'NONE', #14 ) ;
#23108=DIRECTION ( 'NONE',  ( -1.000000000000000000, 0.000000000000000000, 2.257144641399999941E-12 ) ) ;
#23110=ORIENTED_EDGE ( 'NONE', *, *, #11564, .T. ) ;
#23112=VECTOR ( 'NONE', #16674, 1000.000000000000000 ) ;
#23127=LINE ( 'NONE', #14315, #96 ) ;
#23141=EDGE_CURVE ( 'NONE', #7563, #19876, #9559, .T. ) ;
#23148=AXIS2_PLACEMENT_3D ( 'NONE', #4993, #13676, #19151 ) ;
#23152=ORIENTED_EDGE ( 'NONE', *, *, #15508, .T. ) ;
#23153=CARTESIAN_POINT ( 'NONE',  ( -31.50000000000000000, -14.25000000000000000, -150.0552959529999839 ) ) ;
#23157=CARTESIAN_POINT ( 'NONE',  ( -4.500067286957687429, 22.89748944254456831, -150.0552959529999839 ) ) ;
#23168=FACE_OUTER_BOUND ( 'NONE', #1787, .T. ) ;
#23172=ORIENTED_EDGE ( 'NONE', *, *, #17732, .T. ) ;
#23180=ORIENTED_EDGE ( 'NONE', *, *, #10306, .F. ) ;
#23182=CARTESIAN_POINT ( 'NONE',  ( 31.50000000000000000, 40.03620104870000063, -136.0552959530000123 ) ) ;
#23185=AXIS2_PLACEMENT_3D ( 'NONE', #12359, #10344, #19280 ) ;
#23187=AXIS2_PLACEMENT_3D ( 'NONE', #21118, #1261, #11690 ) ;
#23189=VERTEX_POINT ( 'NONE', #479 ) ;
#23190=FACE_OUTER_BOUND ( 'NONE', #2972, .T. ) ;
#23192=FACE_OUTER_BOUND ( 'NONE', #20664, .T. ) ;
#23193=EDGE_LOOP ( 'NONE', ( #12779, #8923, #4693, #14720, #17320, #8681, #17198, #3616, #17012, #15808, #1744 ) ) ;
#23196=DIRECTION ( 'NONE',  ( 1.000000000000000000, 0.000000000000000000, 0.000000000000000000 ) ) ;
#23197=ORIENTED_EDGE ( 'NONE', *, *, #22457, .T. ) ;
#23200=VECTOR ( 'NONE', #364, 1000.000000000000000 ) ;
#23201=CARTESIAN_POINT ( 'NONE',  ( -15.50000000000000000, 47.50000000000000000, -151.0552959529999839 ) ) ;
#23206=ORIENTED_EDGE ( 'NONE', *, *, #9076, .T. ) ;
#23210=DIRECTION ( 'NONE',  ( 1.000000000000000000, 0.000000000000000000, -2.257157423930000049E-12 ) ) ;
#23213=ORIENTED_EDGE ( 'NONE', *, *, #5030, .T. ) ;
#23216=FACE_OUTER_BOUND ( 'NONE', #130, .T. ) ;
#23224=ORIENTED_EDGE ( 'NONE', *, *, #2443, .F. ) ;
#23232=CARTESIAN_POINT ( 'NONE',  ( 19.13369214879999802, -50.49999999980000354, -136.0552959530000123 ) ) ;
#23238=CARTESIAN_POINT ( 'NONE',  ( 0.8488726856734599702, 25.45511797032470369, -150.0552959529999839 ) ) ;
#23249=DIRECTION ( 'NONE',  ( -1.000000000000000000, 0.000000000000000000, -1.457985068979999943E-12 ) ) ;
#23250=VERTEX_POINT ( 'NONE', #2607 ) ;
#23255=ORIENTED_EDGE ( 'NONE', *, *, #21706, .F. ) ;
#23265=CARTESIAN_POINT ( 'NONE',  ( -12.00000000000000000, -43.00000000000000000, -150.0552959529999839 ) ) ;
#23285=ORIENTED_EDGE ( 'NONE', *, *, #1721, .F. ) ;
#23291=LINE ( 'NONE', #17934, #659 ) ;
#23292=VERTEX_POINT ( 'NONE', #4857 ) ;
#23293=LINE ( 'NONE', #15685, #6886 ) ;
#23294=EDGE_LOOP ( 'NONE', ( #10846, #4548, #20761, #20442 ) ) ;
#23297=EDGE_LOOP ( 'NONE', ( #19011, #12972, #10808, #9500 ) ) ;
#23298=CARTESIAN_POINT ( 'NONE',  ( 25.89900052719454848, -22.34364015992473895, -150.0552959529999839 ) ) ;
#23299=EDGE_LOOP ( 'NONE', ( #10493, #19775, #15469, #9374 ) ) ;
#23302=CARTESIAN_POINT ( 'NONE',  ( -5.500000000000000000, 44.23441892295282685, -150.0552959529999839 ) ) ;
#23306=EDGE_LOOP ( 'NONE', ( #18648, #21716, #17843, #17887 ) ) ;
#23312=ORIENTED_EDGE ( 'NONE', *, *, #11008, .T. ) ;
#23316=DIRECTION ( 'NONE',  ( -1.000000000000000000, 0.000000000000000000, 0.000000000000000000 ) ) ;
#23317=ADVANCED_FACE ( 'NONE', ( #2497 ), #4499, .F. ) ;
#23324=DIRECTION ( 'NONE',  ( 0.000000000000000000, -1.000000000000000000, 0.000000000000000000 ) ) ;
#23328=DIRECTION ( 'NONE',  ( 0.000000000000000000, 0.000000000000000000, 1.000000000000000000 ) ) ;
#23337=LINE ( 'NONE', #14291, #6452 ) ;
#23349=EDGE_CURVE ( 'NONE', #21958, #2149, #6170, .T. ) ;
#23355=EDGE_CURVE ( 'NONE', #15840, #9450, #18920, .T. ) ;
#23358=AXIS2_PLACEMENT_3D ( 'NONE', #9996, #17389, #21089 ) ;
#23359=ADVANCED_FACE ( 'NONE', ( #4977 ), #23413, .T. ) ;
#23360=ORIENTED_EDGE ( 'NONE', *, *, #19440, .F. ) ;
#23369=LINE ( 'NONE', #19919, #1547 ) ;
#23372=DIRECTION ( 'NONE',  ( 0.000000000000000000, -1.000000000000000000, 0.000000000000000000 ) ) ;
#23375=CARTESIAN_POINT ( 'NONE',  ( 3.000000000000000000, -3.500000000000000000, -140.0552959529999839 ) ) ;
#23379=PRODUCT_CONTEXT ( 'NONE', #18899, 'mechanical' ) ;
#23380=FACE_OUTER_BOUND ( 'NONE', #22708, .T. ) ;
#23382=CARTESIAN_POINT ( 'NONE',  ( -12.00000000000000000, -43.00000000000000000, -140.0552959529999839 ) ) ;
#23386=ORIENTED_EDGE ( 'NONE', *, *, #391, .T. ) ;
#23387=VECTOR ( 'NONE', #1355, 1000.000000000000000 ) ;
#23390=CARTESIAN_POINT ( 'NONE',  ( -13.86630785140000022, -51.50000000000000000, -136.5552959530000123 ) ) ;
#23393=ORIENTED_EDGE ( 'NONE', *, *, #12130, .F. ) ;
#23397=CARTESIAN_POINT ( 'NONE',  ( -32.50000000000000000, 1.000000000000000000, -149.5552959529999839 ) ) ;
#23403=DIRECTION ( 'NONE',  ( 1.000000000000000000, 0.000000000000000000, 0.000000000000000000 ) ) ;
#23411=CARTESIAN_POINT ( 'NONE',  ( -12.50000000000000000, 45.50000000000000000, -150.0552959529999839 ) ) ;
#23412=ORIENTED_EDGE ( 'NONE', *, *, #68, .T. ) ;
#23413=PLANE ( 'NONE',  #22883 ) ;
#23417=ORIENTED_EDGE ( 'NONE', *, *, #23349, .F. ) ;
#23422=CARTESIAN_POINT ( 'NONE',  ( 31.50000000000000000, 0.000000000000000000, -149.5552959529999839 ) ) ;
#23423=ORIENTED_EDGE ( 'NONE', *, *, #3889, .T. ) ;
#23424=VECTOR ( 'NONE', #1947, 1000.000000000000000 ) ;
#23428=VERTEX_POINT ( 'NONE', #14497 ) ;
#23430=ADVANCED_FACE ( 'NONE', ( #12225, #1773 ), #14139, .F. ) ;
#23434=DIRECTION ( 'NONE',  ( 0.000000000000000000, 0.7071067811870332953, 0.7071067811860618502 ) ) ;
#23436=DIRECTION ( 'NONE',  ( 0.000000000000000000, 1.000000000000000000, 0.000000000000000000 ) ) ;
#23438=VERTEX_POINT ( 'NONE', #6992 ) ;
#23449=DIRECTION ( 'NONE',  ( 1.000000000000000000, 0.000000000000000000, 0.000000000000000000 ) ) ;
#23459=ORIENTED_EDGE ( 'NONE', *, *, #2941, .T. ) ;
#23477=DIRECTION ( 'NONE',  ( -0.6459422414661292189, 0.7633862853691524286, 0.000000000000000000 ) ) ;
#23499=ADVANCED_FACE ( 'NONE', ( #10776 ), #106, .T. ) ;
#23506=CARTESIAN_POINT ( 'NONE',  ( 31.00000000000000000, -39.80430157320000006, -149.5552959529999839 ) ) ;
#23507=EDGE_LOOP ( 'NONE', ( #14419, #12215, #11983, #2451 ) ) ;
#23508=DIRECTION ( 'NONE',  ( 1.000000000000000000, 0.000000000000000000, 0.000000000000000000 ) ) ;
#23516=LINE ( 'NONE', #16380, #17902 ) ;
#23522=VECTOR ( 'NONE', #4486, 1000.000000000000000 ) ;
#23526=VECTOR ( 'NONE', #11992, 1000.000000000000000 ) ;
#23533=CARTESIAN_POINT ( 'NONE',  ( -13.86630785140000022, -51.50000000000000000, -137.0552959530000123 ) ) ;
ENDSEC;
END-ISO-10303-21;
